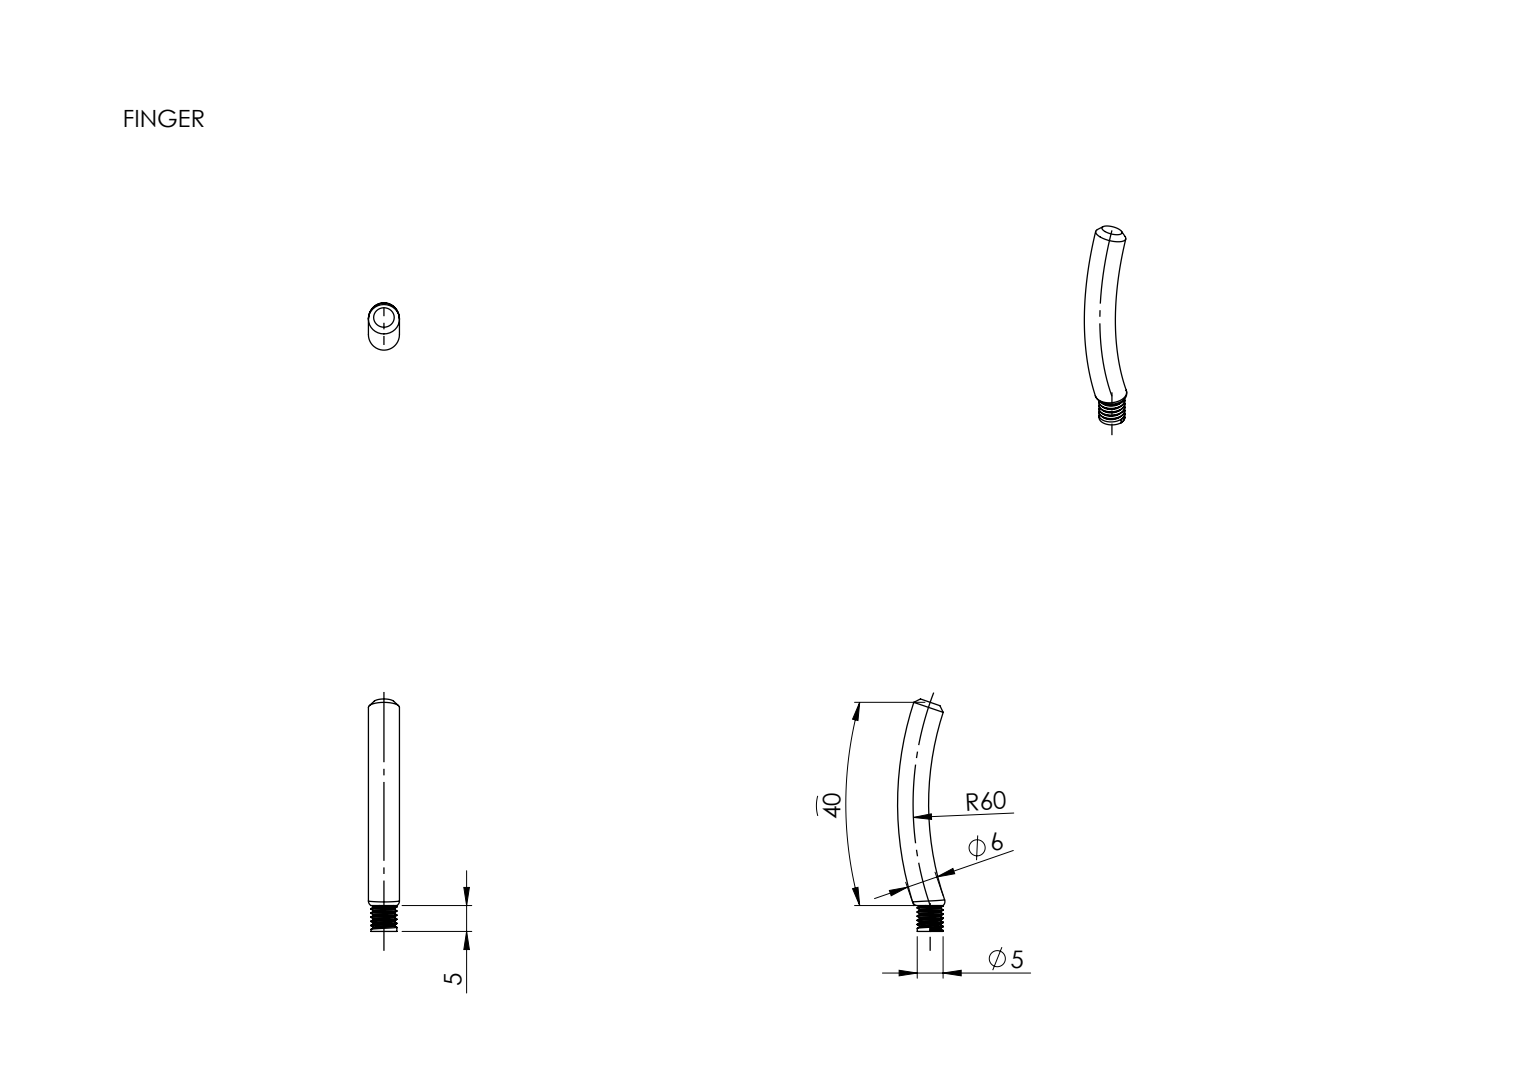
ISO-10303-21;
HEADER;
FILE_DESCRIPTION (('STEP AP214'),
    '1' );
FILE_NAME ('finger.step',
    '2026-10-04T10:31:01',
    ( '' ),
    ( '' ),
    'SwSTEP 2.0',
    'SolidWorks 2026',
    '' );
FILE_SCHEMA (( 'AUTOMOTIVE_DESIGN' ));
ENDSEC;

DATA;
#10=LINE ( 'NONE', #5828, #1733 ) ;
#16=CARTESIAN_POINT ( 'NONE',  ( 0.8561741729129460632, 185.8999999989075036, 9.066987299999999195 ) ) ;
#23=CARTESIAN_POINT ( 'NONE',  ( -2.191511056945971259, 226.6300844452854903, 5.385369267317587472 ) ) ;
#25=VERTEX_POINT ( 'NONE', #11007 ) ;
#31=CARTESIAN_POINT ( 'NONE',  ( -2.499999999999998224, 185.2500000000000284, 8.035533905932741305 ) ) ;
#33=CARTESIAN_POINT ( 'NONE',  ( -2.500000000000000444, 185.8999999978150584, 7.000000000000000000 ) ) ;
#39=CARTESIAN_POINT ( 'NONE',  ( -1.767766952966369320, 186.5999999978150754, 5.232233047033630235 ) ) ;
#40=CARTESIAN_POINT ( 'NONE',  ( 2.467000123265670641, 227.8390626820829823, 8.944723654098295285 ) ) ;
#43=CARTESIAN_POINT ( 'NONE',  ( -2.367714804004699136, 189.3873339094368191, 5.166511778942795452 ) ) ;
#55=CARTESIAN_POINT ( 'NONE',  ( -1.767766952966369765, 186.8300000002185186, 8.767766952966368876 ) ) ;
#57=CARTESIAN_POINT ( 'NONE',  ( 1.989910900261709470, 228.2393533748197569, 6.930657055068108363 ) ) ;
#64=CARTESIAN_POINT ( 'NONE',  ( -0.8561741729129470624, 185.5999999989075206, 9.066987300000000971 ) ) ;
#73=CARTESIAN_POINT ( 'NONE',  ( -1.732476358310940601, 189.0000000000000853, 8.805961798289683173 ) ) ;
#91=CARTESIAN_POINT ( 'NONE',  ( -1.461580736456473018, 188.7499999989075263, 5.538419263543527649 ) ) ;
#100=CARTESIAN_POINT ( 'NONE',  ( -2.809196860006122787, 226.9495188873497966, 6.326437523183426670 ) ) ;
#104=EDGE_LOOP ( 'NONE', ( #9975, #181, #5986, #469 ) ) ;
#106=CARTESIAN_POINT ( 'NONE',  ( 1.753917783834456179, 189.0000000000000568, 8.787807858281036388 ) ) ;
#116=DIRECTION ( 'NONE',  ( -6.123233995736766036E-17, 1.000000000000000000, 0.000000000000000000 ) ) ;
#118=CARTESIAN_POINT ( 'NONE',  ( -7.826584432629735133E-16, 189.2999999978150356, 9.500000000000001776 ) ) ;
#119=CARTESIAN_POINT ( 'NONE',  ( 1.829800800964088481, 226.5245823332902546, 5.074452397578279594 ) ) ;
#121=CARTESIAN_POINT ( 'NONE',  ( -2.425137606382978372, 188.9999999978561505, 7.628313597219490205 ) ) ;
#133=CARTESIAN_POINT ( 'NONE',  ( -2.500000000000000444, 186.7300000002184959, 7.000000000000000000 ) ) ;
#140=CARTESIAN_POINT ( 'NONE',  ( -1.461580736456473906, 186.3499999989074922, 8.461580736456474128 ) ) ;
#143=CARTESIAN_POINT ( 'NONE',  ( 8.809142651444723526E-17, 184.6499999989075320, 4.933012699999999029 ) ) ;
#148=B_SPLINE_CURVE_WITH_KNOTS ( 'NONE', 1,
 ( #12898, #4831 ),
 .UNSPECIFIED., .F., .F.,
 ( 2, 2 ),
 ( 0.000000000000000000, 1.000000000000000000 ),
 .UNSPECIFIED. ) ;
#150=CARTESIAN_POINT ( 'NONE',  ( 1.461580736456472573, 188.9499999989075150, 8.461580736456474128 ) ) ;
#164=VECTOR ( 'NONE', #7946, 1000.000000000000000 ) ;
#177=CARTESIAN_POINT ( 'NONE',  ( -2.923025936753522291, 227.5090509392885281, 7.973756422523831766 ) ) ;
#179=ORIENTED_EDGE ( 'NONE', *, *, #8379, .T. ) ;
#181=ORIENTED_EDGE ( 'NONE', *, *, #13568, .T. ) ;
#194=CARTESIAN_POINT ( 'NONE',  ( 4.404571325722361763E-17, 185.7699999975965568, 4.500000000000000000 ) ) ;
#195=CARTESIAN_POINT ( 'NONE',  ( -1.740752211025599738, 227.9442165381023528, 6.078285037125840340 ) ) ;
#196=CARTESIAN_POINT ( 'NONE',  ( 2.789580270747262780, 227.6450226773988845, 8.373868502673408543 ) ) ;
#197=CARTESIAN_POINT ( 'NONE',  ( 0.3061381340472814627, 189.0451911194899424, 10.17413847366682234 ) ) ;
#200=CARTESIAN_POINT ( 'NONE',  ( -0.2618185962740512407, 189.0446530151151023, 10.17853758010602760 ) ) ;
#208=CARTESIAN_POINT ( 'NONE',  ( 0.9639874461523436633, 228.2061259459514133, 10.02419290002115915 ) ) ;
#210=EDGE_CURVE ( 'NONE', #4790, #898, #15357, .T. ) ;
#217=CARTESIAN_POINT ( 'NONE',  ( -2.500000000000000444, 186.7800000002184504, 8.035533905932737753 ) ) ;
#219=CARTESIAN_POINT ( 'NONE',  ( 0.8799020092372641377, 228.8451675208714562, 8.680282862240067843 ) ) ;
#224=CARTESIAN_POINT ( 'NONE',  ( -2.066987300000001859, 187.8999999989075036, 7.856174172912944620 ) ) ;
#231=CARTESIAN_POINT ( 'NONE',  ( -0.8561741729129471734, 188.7999999989075093, 9.066987300000000971 ) ) ;
#233=CARTESIAN_POINT ( 'NONE',  ( -0.05280792143845736142, 189.0000000000001137, 9.499442202459045248 ) ) ;
#240=CARTESIAN_POINT ( 'NONE',  ( -0.8561741729129455081, 187.0999999989075206, 4.933012699999999029 ) ) ;
#250=CARTESIAN_POINT ( 'NONE',  ( -2.113934160113910998, 227.9745842263959048, 9.343330332359114365 ) ) ;
#251=CARTESIAN_POINT ( 'NONE',  ( -0.8561741729129470624, 188.9999999989074979, 9.066987299999999195 ) ) ;
#258=CARTESIAN_POINT ( 'NONE',  ( -2.548338711267991386, 226.7802694665861338, 5.827877803219676522 ) ) ;
#269=CARTESIAN_POINT ( 'NONE',  ( 1.035533905932737975, 184.8499999978150754, 4.500000000000000888 ) ) ;
#273=CARTESIAN_POINT ( 'NONE',  ( 1.767766952966369320, 185.6699999975965625, 5.232233047033630235 ) ) ;
#274=CARTESIAN_POINT ( 'NONE',  ( 0.1304739971030711432, 227.6100227634930775, 5.113114354890055502 ) ) ;
#276=CARTESIAN_POINT ( 'NONE',  ( -2.974673115704016713, 227.4156934420934419, 7.698994310615434600 ) ) ;
#277=CARTESIAN_POINT ( 'NONE',  ( -2.345330793980067607, 188.9999999986873149, 6.116719614743881372 ) ) ;
#283=CARTESIAN_POINT ( 'NONE',  ( 3.000012661665197200, 227.2854160473209504, 7.315512558684322819 ) ) ;
#291=CARTESIAN_POINT ( 'NONE',  ( -2.500000000000000444, 186.7500000000000000, 5.964466094067261359 ) ) ;
#293=CARTESIAN_POINT ( 'NONE',  ( -0.2610185499608090876, 227.6142484773064325, 5.125318457402467942 ) ) ;
#299=CARTESIAN_POINT ( 'NONE',  ( -1.965116437629976787E-16, 189.2499999989075263, 4.933012699999999029 ) ) ;
#301=CARTESIAN_POINT ( 'NONE',  ( -2.066987300000000971, 188.0999999989074922, 7.856174172912944620 ) ) ;
#309=CARTESIAN_POINT ( 'NONE',  ( 2.593621171579884699, 189.1921907459377792, 8.687688957072346341 ) ) ;
#311=CARTESIAN_POINT ( 'NONE',  ( 3.001999740804089711, 189.8855686313634124, 7.133436250992125416 ) ) ;
#316=CARTESIAN_POINT ( 'NONE',  ( 0.8561741729129460632, 186.6999999989075150, 9.066987299999999195 ) ) ;
#317=( BOUNDED_CURVE ( )  B_SPLINE_CURVE ( 2, ( #9057, #7531, #11422, #13807, #6512 ),
 .UNSPECIFIED., .F., .F. ) 
 B_SPLINE_CURVE_WITH_KNOTS ( ( 3, 2, 3 ),
 ( 0.8571428571428570953, 0.8750000000000000000, 0.8928571428571429047 ),
 .UNSPECIFIED. ) 
 CURVE ( )  GEOMETRIC_REPRESENTATION_ITEM ( )  RATIONAL_B_SPLINE_CURVE ( ( 1.000000000000000000, 0.9238795325112867385, 1.000000000000000000, 0.9238795325112867385, 1.000000000000000000 ) ) 
 REPRESENTATION_ITEM ( '' )  );
#320=VERTEX_POINT ( 'NONE', #684 ) ;
#327=CARTESIAN_POINT ( 'NONE',  ( -2.997549271363485701, 189.8887934741522088, 7.062685571753808844 ) ) ;
#330=( BOUNDED_CURVE ( )  B_SPLINE_CURVE ( 2, ( #15027, #7780, #6448, #7628, #12471, #4120, #1572, #12627, #6600 ),
 .UNSPECIFIED., .F., .F. ) 
 B_SPLINE_CURVE_WITH_KNOTS ( ( 3, 2, 2, 2, 3 ),
 ( 0.3571428571428572063, 0.3750000000000000555, 0.3928571428571429047, 0.4107142857142856984, 0.4285714285714285476 ),
 .UNSPECIFIED. ) 
 CURVE ( )  GEOMETRIC_REPRESENTATION_ITEM ( )  RATIONAL_B_SPLINE_CURVE ( ( 0.9999999999999997780, 0.9238795325112869605, 1.000000000000000000, 0.9238795325112867385, 1.000000000000000000, 0.9238795325112867385, 1.000000000000000000, 0.9238795325112867385, 1.000000000000000000 ) ) 
 REPRESENTATION_ITEM ( '' )  );
#340=CARTESIAN_POINT ( 'NONE',  ( 1.414552619335309291, 189.0000000000000853, 9.066428886377552843 ) ) ;
#347=CARTESIAN_POINT ( 'NONE',  ( -1.035533905932737753, 184.9499999978150413, 4.500000000000000888 ) ) ;
#352=CARTESIAN_POINT ( 'NONE',  ( 2.500000000000000444, 187.1199999975965795, 8.035533905932739529 ) ) ;
#353=CARTESIAN_POINT ( 'NONE',  ( -1.885954199498669270, 228.0508284750123664, 6.386186391668034368 ) ) ;
#354=CARTESIAN_POINT ( 'NONE',  ( -2.087773716237738331, 226.5967140655768048, 5.287030890998575927 ) ) ;
#356=CARTESIAN_POINT ( 'NONE',  ( -2.971600176645282421, 189.3276089958123976, 6.470516599052638540 ) ) ;
#363=CARTESIAN_POINT ( 'NONE',  ( 2.825502441289275968, 227.6141739403474844, 8.283116510204369121 ) ) ;
#369=CARTESIAN_POINT ( 'NONE',  ( -2.500000000000000444, 185.1500000000000057, 5.964466094067261359 ) ) ;
#371=CARTESIAN_POINT ( 'NONE',  ( -1.786743523428754976, 227.9724114945277051, 6.159713679416685572 ) ) ;
#375=CARTESIAN_POINT ( 'NONE',  ( -1.767766952966369542, 184.5000000000000000, 8.767766952966368876 ) ) ;
#377=CARTESIAN_POINT ( 'NONE',  ( -2.066987300000000083, 186.4499999989075150, 7.000000000000000000 ) ) ;
#380=CARTESIAN_POINT ( 'NONE',  ( 0.000000000000000000, 184.0000000000000000, 7.000000000000000000 ) ) ;
#381=CARTESIAN_POINT ( 'NONE',  ( -5.999999999999999112, 227.2817795252328210, 4.165129161027028459 ) ) ;
#383=CARTESIAN_POINT ( 'NONE',  ( 1.818048556411949068, 189.7463703733489524, 9.770364204685183296 ) ) ;
#388=CARTESIAN_POINT ( 'NONE',  ( -0.8070991676978370721, 189.0000000000000000, 4.628151146390497850 ) ) ;
#390=CARTESIAN_POINT ( 'NONE',  ( -1.461580736456473240, 185.7499999989074979, 8.461580736456472351 ) ) ;
#401=CARTESIAN_POINT ( 'NONE',  ( -0.3832019641432907187, 228.2493259063060691, 10.15123907897345568 ) ) ;
#410=CARTESIAN_POINT ( 'NONE',  ( 2.500000000000000444, 186.3499999978150754, 5.964466094067262247 ) ) ;
#414=ORIENTED_EDGE ( 'NONE', *, *, #5071, .T. ) ;
#416=CARTESIAN_POINT ( 'NONE',  ( 1.644293607015084646, 189.0000000000000568, 8.888752495498886574 ) ) ;
#422=CARTESIAN_POINT ( 'NONE',  ( -1.035533905932737975, 186.5499999978150640, 4.500000000000000888 ) ) ;
#423=CARTESIAN_POINT ( 'NONE',  ( 2.500000000000000444, 184.7499999978150527, 5.964466094067262247 ) ) ;
#427=CARTESIAN_POINT ( 'NONE',  ( -1.767766952966369765, 187.6699999975965625, 8.767766952966368876 ) ) ;
#428=CARTESIAN_POINT ( 'NONE',  ( 0.6320692372082544752, 228.2335842258707430, 10.10492066627648988 ) ) ;
#429=CARTESIAN_POINT ( 'NONE',  ( -2.980755195990519191, 227.3998431049529074, 7.652341518474168325 ) ) ;
#431=CARTESIAN_POINT ( 'NONE',  ( -2.464020019946891793, 189.7914691120035400, 9.078875626642586738 ) ) ;
#437=CARTESIAN_POINT ( 'NONE',  ( 2.938271602351877121, 227.0923189680254666, 6.746872328837914878 ) ) ;
#444=CARTESIAN_POINT ( 'NONE',  ( -1.035533905932739751, 186.9499999999999886, 9.500000000000003553 ) ) ;
#447=CARTESIAN_POINT ( 'NONE',  ( -1.385362557672197736, 227.7924883072852822, 5.640085252515396164 ) ) ;
#451=CARTESIAN_POINT ( 'NONE',  ( -1.456896669277396583E-16, 188.4499999989075150, 4.933012699999999029 ) ) ;
#453=CARTESIAN_POINT ( 'NONE',  ( -2.066987300000000527, 188.7999999989075093, 6.143825827087054492 ) ) ;
#454=ORIENTED_EDGE ( 'NONE', *, *, #12708, .F. ) ;
#461=CARTESIAN_POINT ( 'NONE',  ( 2.837060236510290157, 189.8314984584918079, 8.326472016722609837 ) ) ;
#469=ORIENTED_EDGE ( 'NONE', *, *, #9305, .F. ) ;
#470=CARTESIAN_POINT ( 'NONE',  ( -2.066987300000000971, 187.9999999989075263, 6.143825827087054492 ) ) ;
#488=EDGE_CURVE ( 'NONE', #14260, #5268, #1225, .T. ) ;
#504=CARTESIAN_POINT ( 'NONE',  ( -2.500000000000000444, 185.0999999978150754, 7.000000000000000000 ) ) ;
#506=CARTESIAN_POINT ( 'NONE',  ( 1.767766952966368654, 185.4699999975965454, 8.767766952966368876 ) ) ;
#507=CARTESIAN_POINT ( 'NONE',  ( 0.4870669733929915424, 228.2428440931186628, 10.13214456346285708 ) ) ;
#508=CARTESIAN_POINT ( 'NONE',  ( -0.3933619333212962643, 226.3329841201265253, 4.509674143907711041 ) ) ;
#517=CARTESIAN_POINT ( 'NONE',  ( 2.959395828221181191, 227.1267441636075262, 6.848257790201431661 ) ) ;
#523=CARTESIAN_POINT ( 'NONE',  ( -5.929230630780102373E-16, 186.2000000000000171, 9.500000000000001776 ) ) ;
#525=CARTESIAN_POINT ( 'NONE',  ( -1.313542798833678749, 227.7708088449086290, 5.577473728656160645 ) ) ;
#529=CARTESIAN_POINT ( 'NONE',  ( -2.500000000000000444, 185.2000000000000171, 7.000000000000000000 ) ) ;
#531=CARTESIAN_POINT ( 'NONE',  ( 2.066987300000000083, 186.8999999989075320, 6.143825827087054492 ) ) ;
#533=VECTOR ( 'NONE', #5560, 1000.000000000000000 ) ;
#534=EDGE_CURVE ( 'NONE', #7505, #3363, #14632, .T. ) ;
#537=CARTESIAN_POINT ( 'NONE',  ( 0.03982005317027621089, 190.0874997052910658, 4.201869497416318211 ) ) ;
#539=CARTESIAN_POINT ( 'NONE',  ( 3.012851251850296563, 189.2892816699357468, 7.217589605582900525 ) ) ;
#542=CARTESIAN_POINT ( 'NONE',  ( 1.582454879690585958, 190.0440573869416312, 4.656039093731057399 ) ) ;
#547=CARTESIAN_POINT ( 'NONE',  ( 0.8561741729129458411, 187.4999999989075548, 9.066987299999999195 ) ) ;
#555=EDGE_LOOP ( 'NONE', ( #8215, #1137, #7408, #11561, #3893 ) ) ;
#557=EDGE_CURVE ( 'NONE', #1272, #898, #148, .T. ) ;
#569=ORIENTED_EDGE ( 'NONE', *, *, #5071, .F. ) ;
#578=CARTESIAN_POINT ( 'NONE',  ( 2.500000000000000444, 187.0499999978150640, 8.035533905932739529 ) ) ;
#583=CARTESIAN_POINT ( 'NONE',  ( 1.035533905932738197, 189.4199999975965625, 9.500000000000003553 ) ) ;
#584=CARTESIAN_POINT ( 'NONE',  ( 2.379866841847371628, 227.8775224696199473, 9.057852156131547261 ) ) ;
#585=CARTESIAN_POINT ( 'NONE',  ( -2.521794825564176890, 226.7667903661470348, 5.788166807254388146 ) ) ;
#589=ORIENTED_EDGE ( 'NONE', *, *, #3180, .F. ) ;
#592=CARTESIAN_POINT ( 'NONE',  ( 1.461580736456473462, 184.3499999989074922, 5.538419263543526760 ) ) ;
#599=CARTESIAN_POINT ( 'NONE',  ( 2.500000000000000000, 188.7999999999999829, 7.000000000000000000 ) ) ;
#601=CARTESIAN_POINT ( 'NONE',  ( 2.500000000000000444, 186.4000000000000057, 7.000000000000000000 ) ) ;
#602=CARTESIAN_POINT ( 'NONE',  ( -1.938951794131667850, 228.1124887269953092, 6.564264716264994526 ) ) ;
#606=CARTESIAN_POINT ( 'NONE',  ( -2.500000000000000444, 188.3499999999999943, 5.964466094067261359 ) ) ;
#608=CARTESIAN_POINT ( 'NONE',  ( -2.066987300000000527, 187.2999999989075661, 7.856174172912944620 ) ) ;
#611=CARTESIAN_POINT ( 'NONE',  ( 2.500000000000000444, 186.2999999978150356, 7.000000000000000000 ) ) ;
#615=CARTESIAN_POINT ( 'NONE',  ( 1.855150134049648347, 188.9999999974870946, 5.314312548248043555 ) ) ;
#618=CARTESIAN_POINT ( 'NONE',  ( 1.579185070784824285, 228.6572036374857078, 8.137432446265082220 ) ) ;
#623=CARTESIAN_POINT ( 'NONE',  ( 0.8561741729129461742, 186.4999999989075263, 9.066987300000000971 ) ) ;
#625=ORIENTED_EDGE ( 'NONE', *, *, #13568, .F. ) ;
#627=CARTESIAN_POINT ( 'NONE',  ( 2.500000000000000444, 185.5999999999999943, 7.000000000000000000 ) ) ;
#630=CARTESIAN_POINT ( 'NONE',  ( 2.066987300000000527, 184.2499999989074979, 7.000000000000000000 ) ) ;
#649=CARTESIAN_POINT ( 'NONE',  ( -0.8561741729129466183, 184.9999999989074979, 9.066987299999999195 ) ) ;
#656=CARTESIAN_POINT ( 'NONE',  ( 1.498625850689462968, 228.1261123260860018, 9.788931089129667029 ) ) ;
#666=B_SPLINE_CURVE_WITH_KNOTS ( 'NONE', 3,
 ( #4284, #3090, #14057, #693, #7943, #3165, #8023, #4442, #1965, #6841, #9296, #8106, #12945, #2045, #9700, #7070, #6037, #13342, #14371, #11905, #7151, #2363 ),
 .UNSPECIFIED., .F., .F.,
 ( 4, 2, 2, 2, 2, 2, 2, 2, 2, 2, 4 ),
 ( 0.5000000000000000000, 0.5625000000000006661, 0.5937500000000005551, 0.6250000000000004441, 0.6875000000000004441, 0.7500000000000003331, 0.7812500000000003331, 0.8125000000000002220, 0.8750000000000002220, 0.9375000000000001110, 1.000000000000000000 ),
 .UNSPECIFIED. ) ;
#673=CARTESIAN_POINT ( 'NONE',  ( -7.420008617947670970E-16, 188.5999999999999943, 9.500000000000001776 ) ) ;
#674=CARTESIAN_POINT ( 'NONE',  ( -1.813734975128623139, 228.5291423394705532, 7.767584113458720019 ) ) ;
#681=CARTESIAN_POINT ( 'NONE',  ( 2.500000000000000444, 187.1499999999999773, 8.035533905932739529 ) ) ;
#683=ADVANCED_FACE ( 'NONE', ( #7913 ), #4483, .T. ) ;
#684=CARTESIAN_POINT ( 'NONE',  ( 2.500000000000000444, 184.7999999999999829, 7.000000000000000000 ) ) ;
#686=LINE ( 'NONE', #12938, #533 ) ;
#690=CARTESIAN_POINT ( 'NONE',  ( -0.9617334577332378176, 228.2042837055383302, 10.01878807149740602 ) ) ;
#691=CARTESIAN_POINT ( 'NONE',  ( 0.4407554187462536799, 188.9999999991368895, 4.532388850900320065 ) ) ;
#693=CARTESIAN_POINT ( 'NONE',  ( -0.8829701019949064422, 227.6750070165890349, 5.300792584290398679 ) ) ;
#694=CARTESIAN_POINT ( 'NONE',  ( 1.851056454904606685, 228.5003429013454763, 7.684409693542115782 ) ) ;
#699=CARTESIAN_POINT ( 'NONE',  ( -1.461580736456473018, 188.7499999989075263, 5.538419263543527649 ) ) ;
#701=CARTESIAN_POINT ( 'NONE',  ( 1.035533905932738419, 184.6500000000000057, 9.500000000000000000 ) ) ;
#710=CARTESIAN_POINT ( 'NONE',  ( -1.767766952966369098, 185.0999999999999943, 5.232233047033630235 ) ) ;
#716=CARTESIAN_POINT ( 'NONE',  ( -5.999999999999999112, 229.2449477060184222, 9.834870838912449287 ) ) ;
#728=CARTESIAN_POINT ( 'NONE',  ( 2.500000000000000444, 184.7999999999999829, 7.000000000000000000 ) ) ;
#733=CARTESIAN_POINT ( 'NONE',  ( -1.035533905932737975, 188.9499999978150697, 4.500000000000000888 ) ) ;
#741=CARTESIAN_POINT ( 'NONE',  ( 0.09789622041826544219, 228.2551367208810689, 10.16828408546989237 ) ) ;
#749=CARTESIAN_POINT ( 'NONE',  ( 1.035533905932738197, 189.3499999978150754, 9.500000000000000000 ) ) ;
#759=CARTESIAN_POINT ( 'NONE',  ( -1.035533905932737975, 188.2500000000000000, 4.500000000000000888 ) ) ;
#761=CARTESIAN_POINT ( 'NONE',  ( -1.987493679921816137, 228.2178828950600860, 6.868649084925799286 ) ) ;
#763=AXIS2_PLACEMENT_3D ( 'NONE', #4855, #7470, #14549 ) ;
#766=CARTESIAN_POINT ( 'NONE',  ( 1.767766952966369098, 187.2999999999999829, 5.232233047033630235 ) ) ;
#774=CARTESIAN_POINT ( 'NONE',  ( -0.1991118202061275544, 190.0875178197513549, 4.201689379953633008 ) ) ;
#777=CARTESIAN_POINT ( 'NONE',  ( 1.035533905932737975, 184.0800000002185186, 4.500000000000000888 ) ) ;
#779=CARTESIAN_POINT ( 'NONE',  ( 1.725625307041983136, 227.9349420198840903, 6.051499699527947307 ) ) ;
#784=CARTESIAN_POINT ( 'NONE',  ( 5.082197683525802034E-17, 185.2499999989074979, 4.933012699999999029 ) ) ;
#791=CARTESIAN_POINT ( 'NONE',  ( -1.461580736456473018, 185.3499999989074922, 5.538419263543526760 ) ) ;
#796=CARTESIAN_POINT ( 'NONE',  ( 3.659182332138577465E-16, 187.9952603975225713, 3.440894205938198613 ) ) ;
#811=CARTESIAN_POINT ( 'NONE',  ( -1.767766952966369765, 189.1999999978150697, 8.767766952966368876 ) ) ;
#813=CARTESIAN_POINT ( 'NONE',  ( 2.500000000000000444, 185.4999999978150527, 7.000000000000000000 ) ) ;
#819=CARTESIAN_POINT ( 'NONE',  ( 3.000032282732917555, 227.2742683068891552, 7.282695486718367306 ) ) ;
#823=( BOUNDED_CURVE ( )  B_SPLINE_CURVE ( 2, ( #1831, #12882, #13771, #14977, #5431, #11461, #11535, #11617, #4068 ),
 .UNSPECIFIED., .F., .F. ) 
 B_SPLINE_CURVE_WITH_KNOTS ( ( 3, 2, 2, 2, 3 ),
 ( 0.5000000000000000000, 0.5178571428571429047, 0.5357142857142856984, 0.5535714285714286031, 0.5714285714285713969 ),
 .UNSPECIFIED. ) 
 CURVE ( )  GEOMETRIC_REPRESENTATION_ITEM ( )  RATIONAL_B_SPLINE_CURVE ( ( 1.000000000000000000, 0.9238795325112867385, 1.000000000000000000, 0.9238795325112867385, 1.000000000000000000, 0.9238795325112867385, 1.000000000000000000, 0.9238795325112867385, 1.000000000000000000 ) ) 
 REPRESENTATION_ITEM ( '' )  );
#832=PRESENTATION_STYLE_ASSIGNMENT (( #6370 ) ) ;
#837=CARTESIAN_POINT ( 'NONE',  ( 1.035533905932737975, 184.8499999978150754, 4.500000000000000888 ) ) ;
#839=CARTESIAN_POINT ( 'NONE',  ( -0.6401557763822781633, 228.8776351522889172, 8.774051233606112277 ) ) ;
#843=CARTESIAN_POINT ( 'NONE',  ( 0.03582210218219494119, 189.0000000000000284, 4.500171129856880725 ) ) ;
#844=CARTESIAN_POINT ( 'NONE',  ( 2.500000000000000444, 188.0500000000000114, 5.964466094067262247 ) ) ;
#845=CARTESIAN_POINT ( 'NONE',  ( -1.767766952966369320, 187.3999999978150584, 5.232233047033630235 ) ) ;
#851=CARTESIAN_POINT ( 'NONE',  ( -2.781333881087624249, 226.9279571253883319, 6.262926915399051886 ) ) ;
#856=CARTESIAN_POINT ( 'NONE',  ( 1.362382138968808887, 227.7849605967929847, 5.618344795260735935 ) ) ;
#861=CARTESIAN_POINT ( 'NONE',  ( 2.066987299999999639, 189.2499999989075263, 7.000000000000000000 ) ) ;
#864=CARTESIAN_POINT ( 'NONE',  ( 2.500000000000000444, 186.4000000000000057, 7.000000000000000000 ) ) ;
#865=CARTESIAN_POINT ( 'NONE',  ( 1.461580736456473018, 185.3499999989075206, 5.538419263543527649 ) ) ;
#867=CARTESIAN_POINT ( 'NONE',  ( -9.825582188149883933E-17, 187.6499999989075320, 4.933012699999999029 ) ) ;
#872=CARTESIAN_POINT ( 'NONE',  ( 3.659182332138577465E-16, 195.9172377311516016, 6.220370292208427188 ) ) ;
#875=DIRECTION ( 'NONE',  ( -6.123233995736766036E-17, 1.000000000000000000, 0.000000000000000000 ) ) ;
#881=CARTESIAN_POINT ( 'NONE',  ( 1.002352689154774934, 228.8297273714526625, 8.635690830070354096 ) ) ;
#886=CARTESIAN_POINT ( 'NONE',  ( 0.8561741729129461742, 185.0999999989074922, 9.066987299999999195 ) ) ;
#892=CARTESIAN_POINT ( 'NONE',  ( 2.998712701283978710, 227.3219367242041926, 7.423021690895281743 ) ) ;
#893=CARTESIAN_POINT ( 'NONE',  ( -1.238695443643032412, 228.1695118093442716, 9.916540120957755278 ) ) ;
#898=VERTEX_POINT ( 'NONE', #13447 ) ;
#911=CARTESIAN_POINT ( 'NONE',  ( 2.500000000000000444, 185.5499999978150640, 5.964466094067262247 ) ) ;
#912=CARTESIAN_POINT ( 'NONE',  ( -1.785671180686238868, 228.5485690224869586, 7.823689482036285447 ) ) ;
#915=CARTESIAN_POINT ( 'NONE',  ( -0.1354819475358782221, 189.4421779970482760, 3.974290229956241038 ) ) ;
#916=CARTESIAN_POINT ( 'NONE',  ( 1.035533905932737753, 186.5499999999999829, 4.500000000000000888 ) ) ;
#923=EDGE_CURVE ( 'NONE', #15371, #5418, #15489, .T. ) ;
#925=CARTESIAN_POINT ( 'NONE',  ( -2.774519402982507543, 226.9225964823893378, 6.247138756163614914 ) ) ;
#926=PRESENTATION_STYLE_ASSIGNMENT (( #5953 ) ) ;
#927=CARTESIAN_POINT ( 'NONE',  ( 1.616071383507818870, 190.0421234246860820, 4.677467377199475251 ) ) ;
#928=CARTESIAN_POINT ( 'NONE',  ( -2.500000000000000444, 184.3800000002184731, 8.035533905932737753 ) ) ;
#931=CARTESIAN_POINT ( 'NONE',  ( 1.050562149602352946, 228.8138732705275231, 8.589903282340008772 ) ) ;
#936=CARTESIAN_POINT ( 'NONE',  ( -2.066987300000001415, 188.8999999989075320, 7.856174172912944620 ) ) ;
#946=CARTESIAN_POINT ( 'NONE',  ( -0.8561741729129457301, 185.2999999989075661, 4.933012699999999029 ) ) ;
#951=CARTESIAN_POINT ( 'NONE',  ( -5.999999999999999112, 187.2933328889893403, 9.583808270834989429 ) ) ;
#952=CARTESIAN_POINT ( 'NONE',  ( -1.097593809647108287, 189.0000000000000000, 9.257041379597499287 ) ) ;
#956=AXIS2_PLACEMENT_3D ( 'NONE', #13283, #2700, #14724 ) ;
#961=CARTESIAN_POINT ( 'NONE',  ( -0.8561741729129467293, 184.9999999989074979, 9.066987299999999195 ) ) ;
#963=ORIENTED_EDGE ( 'NONE', *, *, #15525, .T. ) ;
#967=CARTESIAN_POINT ( 'NONE',  ( -0.8561741729129455081, 186.2999999989075093, 4.933012699999999029 ) ) ;
#968=EDGE_CURVE ( 'NONE', #3363, #12097, #1421, .T. ) ;
#974=CARTESIAN_POINT ( 'NONE',  ( 2.257611286988003396, 226.6535225833466427, 5.454435118953909978 ) ) ;
#981=ORIENTED_EDGE ( 'NONE', *, *, #4957, .F. ) ;
#995=CARTESIAN_POINT ( 'NONE',  ( 2.500000000000000000, 188.0000000000000000, 7.000000000000000000 ) ) ;
#996=CARTESIAN_POINT ( 'NONE',  ( 1.455795469679321608, 228.1339131991090596, 9.811868761735363265 ) ) ;
#998=CARTESIAN_POINT ( 'NONE',  ( 0.07162669437691278340, 189.0000000000000000, 4.501026287322612340 ) ) ;
#1010=CARTESIAN_POINT ( 'NONE',  ( -2.999884802989111421, 227.2993432378640932, 7.356512168893465820 ) ) ;
#1011=( NAMED_UNIT ( * ) PLANE_ANGLE_UNIT ( ) SI_UNIT ( $, .RADIAN. ) );
#1013=CARTESIAN_POINT ( 'NONE',  ( -1.767766952966369542, 184.4300000002185129, 8.767766952966368876 ) ) ;
#1015=CARTESIAN_POINT ( 'NONE',  ( -1.986723294250032357, 228.3028615258686500, 7.114072217564876510 ) ) ;
#1020=CARTESIAN_POINT ( 'NONE',  ( 0.8561741729129460632, 188.0999999989074922, 9.066987300000000971 ) ) ;
#1023=CARTESIAN_POINT ( 'NONE',  ( 2.500000000000000444, 186.3499999999999943, 8.035533905932739529 ) ) ;
#1026=CARTESIAN_POINT ( 'NONE',  ( -2.500000000000000444, 186.6999999978150697, 7.000000000000000000 ) ) ;
#1027=CARTESIAN_POINT ( 'NONE',  ( -0.8561741729129469514, 186.3999999989075320, 9.066987300000000971 ) ) ;
#1041=CARTESIAN_POINT ( 'NONE',  ( -2.066987300000000083, 185.5999999989075491, 6.143825827087054492 ) ) ;
#1048=CARTESIAN_POINT ( 'NONE',  ( 2.066987299999999195, 188.3999999989075036, 7.856174172912946396 ) ) ;
#1054=CARTESIAN_POINT ( 'NONE',  ( 2.191560967657306680, 226.6301005958437145, 5.385416860794732585 ) ) ;
#1075=CARTESIAN_POINT ( 'NONE',  ( -1.035533905932739751, 188.4499999978150413, 9.500000000000003553 ) ) ;
#1076=CARTESIAN_POINT ( 'NONE',  ( 2.441738273555474681, 226.7282248110694809, 5.674544857840881029 ) ) ;
#1078=CARTESIAN_POINT ( 'NONE',  ( -2.102556124205833044, 189.0000000003525997, 5.635613679834785117 ) ) ;
#1079=EDGE_CURVE ( 'NONE', #14331, #15449, #9378, .T. ) ;
#1087=CARTESIAN_POINT ( 'NONE',  ( 2.658620627125748204, 226.8422998350077080, 6.010601022363255552 ) ) ;
#1090=CARTESIAN_POINT ( 'NONE',  ( -2.985771267271970064, 227.3851189813470910, 7.609035584520301043 ) ) ;
#1092=CARTESIAN_POINT ( 'NONE',  ( 1.035533905932737753, 188.0800000002184902, 4.500000000000000888 ) ) ;
#1094=CARTESIAN_POINT ( 'NONE',  ( -0.06647456835015956578, 227.6089819833846093, 5.110108522575333545 ) ) ;
#1098=ORIENTED_EDGE ( 'NONE', *, *, #5480, .T. ) ;
#1099=CARTESIAN_POINT ( 'NONE',  ( -0.8561741729129471734, 187.9999999989075263, 9.066987300000000971 ) ) ;
#1101=CARTESIAN_POINT ( 'NONE',  ( 2.066987300000000083, 187.3999999989075320, 7.856174172912946396 ) ) ;
#1107=CARTESIAN_POINT ( 'NONE',  ( 5.999999999999999112, 229.2449477060184222, 9.834870838912449287 ) ) ;
#1108=CARTESIAN_POINT ( 'NONE',  ( 1.461580736456472573, 188.1499999989075036, 8.461580736456474128 ) ) ;
#1113=DIRECTION ( 'NONE',  ( 2.168404344970946942E-15, -1.000000000000000000, -0.000000000000000000 ) ) ;
#1125=CARTESIAN_POINT ( 'NONE',  ( 1.461580736456472795, 188.5499999989075093, 5.538419263543527649 ) ) ;
#1131=CARTESIAN_POINT ( 'NONE',  ( 0.4902782441471901231, 226.3376063806459513, 4.523301387120397088 ) ) ;
#1136=ORIENTED_EDGE ( 'NONE', *, *, #3553, .F. ) ;
#1137=ORIENTED_EDGE ( 'NONE', *, *, #5238, .T. ) ;
#1150=CARTESIAN_POINT ( 'NONE',  ( -2.500000000000000444, 188.2499999978150242, 5.964466094067261359 ) ) ;
#1151=CARTESIAN_POINT ( 'NONE',  ( 2.734462269239809729, 226.8914732116195125, 6.155466831691636109 ) ) ;
#1158=EDGE_LOOP ( 'NONE', ( #4293, #1590, #2533, #13794 ) ) ;
#1164=CARTESIAN_POINT ( 'NONE',  ( -1.569056679521910747, 226.4669167303270285, 4.904463601914050841 ) ) ;
#1168=CARTESIAN_POINT ( 'NONE',  ( 2.500000000000000444, 187.9800000002184959, 5.964466094067262247 ) ) ;
#1170=CARTESIAN_POINT ( 'NONE',  ( 1.986575337946455022, 228.3035988107396292, 7.116201538324070874 ) ) ;
#1175=CARTESIAN_POINT ( 'NONE',  ( -2.066987300000000971, 187.8499999989074922, 7.000000000000000000 ) ) ;
#1176=CARTESIAN_POINT ( 'NONE',  ( -4.811147140404425926E-16, 185.6499999989075320, 9.066987300000000971 ) ) ;
#1185=CARTESIAN_POINT ( 'NONE',  ( 1.214065608363191773, 189.0732342899627554, 9.931872992141947520 ) ) ;
#1190=CARTESIAN_POINT ( 'NONE',  ( 2.500000000000000444, 187.2500000000000000, 5.964466094067262247 ) ) ;
#1192=ORIENTED_EDGE ( 'NONE', *, *, #7499, .T. ) ;
#1196=ORIENTED_EDGE ( 'NONE', *, *, #14425, .T. ) ;
#1201=CARTESIAN_POINT ( 'NONE',  ( -0.8561741729129467293, 186.5999999989075206, 9.066987299999999195 ) ) ;
#1208=CARTESIAN_POINT ( 'NONE',  ( -1.586193948774629714, 228.1096603596491832, 9.740555404025270647 ) ) ;
#1225=( BOUNDED_CURVE ( )  B_SPLINE_CURVE ( 2, ( #7222, #1312, #3703, #5945, #2434, #10948, #6026, #13171, #4990 ),
 .UNSPECIFIED., .F., .F. ) 
 B_SPLINE_CURVE_WITH_KNOTS ( ( 3, 2, 2, 2, 3 ),
 ( 0.6428571428571429047, 0.6607142857142856984, 0.6785714285714286031, 0.6964285714285713969, 0.7142857142857143016 ),
 .UNSPECIFIED. ) 
 CURVE ( )  GEOMETRIC_REPRESENTATION_ITEM ( )  RATIONAL_B_SPLINE_CURVE ( ( 1.000000000000000000, 0.9238795325112867385, 1.000000000000000000, 0.9238795325112867385, 1.000000000000000000, 0.9238795325112867385, 1.000000000000000000, 0.9238795325112867385, 1.000000000000000000 ) ) 
 REPRESENTATION_ITEM ( '' )  );
#1227=CARTESIAN_POINT ( 'NONE',  ( -1.767766952966369320, 188.2999999999999829, 5.232233047033630235 ) ) ;
#1230=CARTESIAN_POINT ( 'NONE',  ( 1.035533905932737753, 188.0499999978150640, 4.500000000000000888 ) ) ;
#1231=CARTESIAN_POINT ( 'NONE',  ( 1.978507955918972439, 228.0159604248740663, 9.465015589616863068 ) ) ;
#1235=CARTESIAN_POINT ( 'NONE',  ( -1.760080037233190620, 188.9999999985105887, 5.215340696719847458 ) ) ;
#1247=CARTESIAN_POINT ( 'NONE',  ( 1.767766952966369320, 184.0999999999999943, 5.232233047033630235 ) ) ;
#1249=CARTESIAN_POINT ( 'NONE',  ( 0.5151998000674417044, 228.8897689535086784, 8.809094343595948118 ) ) ;
#1253=CARTESIAN_POINT ( 'NONE',  ( -1.456896669277396583E-16, 188.4499999989075150, 4.933012699999999029 ) ) ;
#1254=CARTESIAN_POINT ( 'NONE',  ( 1.461580736456472573, 187.3499999989074922, 8.461580736456474128 ) ) ;
#1262=CARTESIAN_POINT ( 'NONE',  ( -1.474837674502392115, 189.0000000000000568, 9.021725798137643082 ) ) ;
#1272=VERTEX_POINT ( 'NONE', #10086 ) ;
#1281=CARTESIAN_POINT ( 'NONE',  ( -5.421010862427522170E-16, 186.6499999989075320, 9.066987300000000971 ) ) ;
#1288=CARTESIAN_POINT ( 'NONE',  ( -3.000008639299222235, 227.3051114066062155, 7.373492455173472848 ) ) ;
#1301=CARTESIAN_POINT ( 'NONE',  ( 0.000000000000000000, 184.0000000000000000, 7.000000000000000000 ) ) ;
#1303=CARTESIAN_POINT ( 'NONE',  ( -4.743384504624081899E-17, 187.2999999978150356, 4.500000000000000000 ) ) ;
#1305=CARTESIAN_POINT ( 'NONE',  ( 2.053141855112443626, 226.5855735425530497, 5.254201149538955562 ) ) ;
#1308=CARTESIAN_POINT ( 'NONE',  ( -2.990615845299959386, 189.8642828410552568, 7.611177514557324386 ) ) ;
#1312=CARTESIAN_POINT ( 'NONE',  ( -2.500000000000001776, 187.6500000000000057, 8.035533905932737753 ) ) ;
#1316=( BOUNDED_CURVE ( )  B_SPLINE_CURVE ( 2, ( #3770, #7290, #8570, #6015, #13628, #12126, #1227, #6178, #2507 ),
 .UNSPECIFIED., .F., .F. ) 
 B_SPLINE_CURVE_WITH_KNOTS ( ( 3, 2, 2, 2, 3 ),
 ( 0.7142857142857143016, 0.7321428571428570953, 0.7500000000000000000, 0.7678571428571429047, 0.7857142857142856984 ),
 .UNSPECIFIED. ) 
 CURVE ( )  GEOMETRIC_REPRESENTATION_ITEM ( )  RATIONAL_B_SPLINE_CURVE ( ( 1.000000000000000000, 0.9238795325112867385, 1.000000000000000000, 0.9238795325112867385, 1.000000000000000000, 0.9238795325112867385, 1.000000000000000000, 0.9238795325112867385, 1.000000000000000000 ) ) 
 REPRESENTATION_ITEM ( '' )  );
#1322=CARTESIAN_POINT ( 'NONE',  ( 1.035533905932738197, 186.9800000002184674, 9.500000000000003553 ) ) ;
#1325=CARTESIAN_POINT ( 'NONE',  ( 1.159630251547017377, 228.7900363578050928, 8.521060918829135744 ) ) ;
#1329=ADVANCED_FACE ( 'NONE', ( #15019 ), #4027, .T. ) ;
#1331=CARTESIAN_POINT ( 'NONE',  ( 1.461580736456473240, 186.7499999989075263, 5.538419263543526760 ) ) ;
#1332=CARTESIAN_POINT ( 'NONE',  ( -0.8561741729129469514, 184.7999999989075093, 9.066987300000000971 ) ) ;
#1340=CARTESIAN_POINT ( 'NONE',  ( 5.999999999999999112, 188.6555110544239824, 3.692234042173051289 ) ) ;
#1348=( BOUNDED_CURVE ( )  B_SPLINE_CURVE ( 2, ( #10407, #14208, #8258, #15500, #4597, #14130, #12939, #9217, #6837 ),
 .UNSPECIFIED., .F., .F. ) 
 B_SPLINE_CURVE_WITH_KNOTS ( ( 3, 2, 2, 2, 3 ),
 ( 0.4285714285714285476, 0.4464285714285714524, 0.4642857142857143016, 0.4821428571428571508, 0.5000000000000000000 ),
 .UNSPECIFIED. ) 
 CURVE ( )  GEOMETRIC_REPRESENTATION_ITEM ( )  RATIONAL_B_SPLINE_CURVE ( ( 1.000000000000000000, 0.9238795325112867385, 1.000000000000000000, 0.9238795325112867385, 1.000000000000000000, 0.9238795325112867385, 1.000000000000000000, 0.9238795325112867385, 1.000000000000000000 ) ) 
 REPRESENTATION_ITEM ( '' )  );
#1353=DIRECTION ( 'NONE',  ( -1.000000000000000000, -6.123233995736766036E-17, 0.000000000000000000 ) ) ;
#1368=CARTESIAN_POINT ( 'NONE',  ( -2.980755195990519191, 227.3998431049529074, 7.652341518474168325 ) ) ;
#1374=CARTESIAN_POINT ( 'NONE',  ( 0.6408967124214390854, 189.0000000000000000, 9.420550828545728450 ) ) ;
#1383=CARTESIAN_POINT ( 'NONE',  ( 1.035533905932737975, 185.7199999975966023, 4.500000000000000888 ) ) ;
#1384=CARTESIAN_POINT ( 'NONE',  ( -1.673363231402341000, 227.9073979391035891, 5.971950823222174520 ) ) ;
#1385=CARTESIAN_POINT ( 'NONE',  ( 1.059913075168976260, 226.3867898013274669, 4.668296007112484602 ) ) ;
#1386=CARTESIAN_POINT ( 'NONE',  ( -0.2831953767659359800, 189.6983146630735177, 10.38325066061015178 ) ) ;
#1392=CARTESIAN_POINT ( 'NONE',  ( 0.07962197837297851910, 190.0874091994478761, 4.202769589527710181 ) ) ;
#1397=CARTESIAN_POINT ( 'NONE',  ( -1.035533905932737975, 186.5800000002185470, 4.500000000000000888 ) ) ;
#1400=CARTESIAN_POINT ( 'NONE',  ( 1.637003574519428017, 228.6312591184326948, 8.062503195461440342 ) ) ;
#1405=CARTESIAN_POINT ( 'NONE',  ( 1.767766952966368654, 185.5000000000000000, 8.767766952966368876 ) ) ;
#1421=LINE ( 'NONE', #10104, #7537 ) ;
#1424=CARTESIAN_POINT ( 'NONE',  ( -6.403569081242510563E-16, 188.2499999989075263, 9.066987300000000971 ) ) ;
#1434=CARTESIAN_POINT ( 'NONE',  ( -1.815878914417024204, 228.0587508443335309, 9.590870893335578629 ) ) ;
#1441=CARTESIAN_POINT ( 'NONE',  ( -1.585166063744550602, 226.4701105292460568, 4.913902397277155387 ) ) ;
#1446=CARTESIAN_POINT ( 'NONE',  ( 1.742858872693429761, 189.0000000000000000, 5.171082332538968984 ) ) ;
#1453=CARTESIAN_POINT ( 'NONE',  ( -6.844026213814746740E-16, 187.6999999978150697, 9.500000000000001776 ) ) ;
#1454=CARTESIAN_POINT ( 'NONE',  ( 2.066987300000000527, 185.0499999989075093, 7.000000000000000000 ) ) ;
#1459=CARTESIAN_POINT ( 'NONE',  ( 1.767766952966369320, 184.8699999975965511, 5.232233047033630235 ) ) ;
#1460=CARTESIAN_POINT ( 'NONE',  ( -1.987493679921816137, 228.2178828950600860, 6.868649084925799286 ) ) ;
#1461=CARTESIAN_POINT ( 'NONE',  ( -2.753288529192227774, 227.6732037325579654, 8.456785184543583966 ) ) ;
#1464=CARTESIAN_POINT ( 'NONE',  ( -2.880481771649630485, 189.8381383517797758, 8.187469944237161457 ) ) ;
#1470=CARTESIAN_POINT ( 'NONE',  ( 2.773164530494548696, 227.6577475117620679, 8.411308552413421680 ) ) ;
#1478=CARTESIAN_POINT ( 'NONE',  ( -1.035533905932739529, 185.3499999999999659, 9.500000000000003553 ) ) ;
#1480=CARTESIAN_POINT ( 'NONE',  ( 0.6402346998162695701, 228.8776282932165600, 8.774031424212344277 ) ) ;
#1484=CARTESIAN_POINT ( 'NONE',  ( 2.066987300000000083, 189.0999999989075206, 6.143825827087054492 ) ) ;
#1487=CARTESIAN_POINT ( 'NONE',  ( -0.8561741729129455081, 186.2999999989075093, 4.933012699999999029 ) ) ;
#1493=CARTESIAN_POINT ( 'NONE',  ( -5.999999999999999112, 194.5935680195190116, 12.11154058223188379 ) ) ;
#1497=FACE_OUTER_BOUND ( 'NONE', #555, .T. ) ;
#1499=CARTESIAN_POINT ( 'NONE',  ( -2.500000000000000444, 188.2499999978150527, 5.964466094067261359 ) ) ;
#1500=CARTESIAN_POINT ( 'NONE',  ( 2.390857953333830554, 189.7853064097493530, 9.182117214708636510 ) ) ;
#1505=CARTESIAN_POINT ( 'NONE',  ( 2.066987300000000083, 186.0499999989075093, 7.000000000000000000 ) ) ;
#1515=CARTESIAN_POINT ( 'NONE',  ( -1.055448890735882106, 228.1934063406578446, 9.986798501930948646 ) ) ;
#1524=CARTESIAN_POINT ( 'NONE',  ( -1.035533905932737975, 186.5499999978150356, 4.500000000000001776 ) ) ;
#1531=CARTESIAN_POINT ( 'NONE',  ( 2.392413149609226686, 188.9999999999999716, 7.742749228504306025 ) ) ;
#1538=CARTESIAN_POINT ( 'NONE',  ( -1.767766952966369765, 186.7999999978150356, 8.767766952966368876 ) ) ;
#1543=CARTESIAN_POINT ( 'NONE',  ( -2.500000000000000444, 185.2199999975965738, 8.035533905932737753 ) ) ;
#1544=CARTESIAN_POINT ( 'NONE',  ( 0.8818167416564541838, 227.6759890937897239, 5.303628879260831042 ) ) ;
#1545=CARTESIAN_POINT ( 'NONE',  ( -1.104351905119298705, 226.3927175376774699, 4.685770134608635118 ) ) ;
#1546=CARTESIAN_POINT ( 'NONE',  ( -1.934526094385236483, 189.7531569016572632, 9.674728188581434907 ) ) ;
#1547=B_SPLINE_CURVE_WITH_KNOTS ( 'NONE', 3,
 ( #15097, #11740, #843, #5708, #10551 ),
 .UNSPECIFIED., .F., .F.,
 ( 4, 1, 4 ),
 ( 0.7688659053744423266, 0.7708896602024635225, 0.7729134150304846074 ),
 .UNSPECIFIED. ) ;
#1553=CARTESIAN_POINT ( 'NONE',  ( 2.968835193067500988, 227.4419886495170715, 7.776466547877070923 ) ) ;
#1560=CARTESIAN_POINT ( 'NONE',  ( -1.767766952966369098, 185.0999999999999943, 5.232233047033630235 ) ) ;
#1562=CARTESIAN_POINT ( 'NONE',  ( -1.454198809819935878, 227.8150368499753995, 5.705206729889046535 ) ) ;
#1567=CARTESIAN_POINT ( 'NONE',  ( 2.066987300000000083, 188.2999999989075093, 6.143825827087054492 ) ) ;
#1569=CARTESIAN_POINT ( 'NONE',  ( -1.461580736456473462, 188.1499999989075320, 8.461580736456472351 ) ) ;
#1572=CARTESIAN_POINT ( 'NONE',  ( 1.767766952966368432, 186.9999999978150527, 8.767766952966368876 ) ) ;
#1573=CARTESIAN_POINT ( 'NONE',  ( 3.659182332138577465E-16, 221.4150671951173308, 6.196499129422101682 ) ) ;
#1576=CARTESIAN_POINT ( 'NONE',  ( 1.447897648385842562, 188.9999999996366569, 4.953942678156875168 ) ) ;
#1578=CARTESIAN_POINT ( 'NONE',  ( 1.410416696976425799, 190.0533888663666175, 4.554553427631445217 ) ) ;
#1583=CARTESIAN_POINT ( 'NONE',  ( 2.066987300000000083, 186.8499999989075206, 7.000000000000000000 ) ) ;
#1590=ORIENTED_EDGE ( 'NONE', *, *, #15629, .T. ) ;
#1593=CARTESIAN_POINT ( 'NONE',  ( -2.986011043896227513, 189.8622845448325052, 7.656297732253541710 ) ) ;
#1606=CARTESIAN_POINT ( 'NONE',  ( 0.2265647687538700217, 188.9999999999999716, 9.493607779905927302 ) ) ;
#1614=CARTESIAN_POINT ( 'NONE',  ( -2.500000000000000444, 186.6999999978150697, 7.000000000000000000 ) ) ;
#1619=CARTESIAN_POINT ( 'NONE',  ( -2.500000000000000444, 186.0199999975965568, 8.035533905932737753 ) ) ;
#1620=CARTESIAN_POINT ( 'NONE',  ( -1.212431555520800508, 228.7775460029053534, 8.484988061474600940 ) ) ;
#1621=CARTESIAN_POINT ( 'NONE',  ( -2.191511056945971259, 226.6300844452854903, 5.385369267317587472 ) ) ;
#1623=CARTESIAN_POINT ( 'NONE',  ( -2.353560662074906773, 189.1623160119228544, 9.042440134401656948 ) ) ;
#1627=EDGE_CURVE ( 'NONE', #1738, #3723, #666, .T. ) ;
#1631=CARTESIAN_POINT ( 'NONE',  ( 2.988911113477941583, 227.2040587690521534, 7.075956526733278018 ) ) ;
#1634=CARTESIAN_POINT ( 'NONE',  ( -2.500000000000001776, 188.4500000000000171, 8.035533905932737753 ) ) ;
#1635=CARTESIAN_POINT ( 'NONE',  ( 2.500000000000000444, 185.5500000000000114, 8.035533905932739529 ) ) ;
#1638=CARTESIAN_POINT ( 'NONE',  ( 0.8818167416564541838, 227.6759890937897239, 5.303628879260831042 ) ) ;
#1643=CARTESIAN_POINT ( 'NONE',  ( -2.066987300000001415, 187.7999999989075093, 6.143825827087054492 ) ) ;
#1645=CARTESIAN_POINT ( 'NONE',  ( 2.066987299999999195, 188.3999999989075320, 7.856174172912946396 ) ) ;
#1651=DIRECTION ( 'NONE',  ( 1.000000000000000000, 0.000000000000000000, 0.000000000000000000 ) ) ;
#1652=CARTESIAN_POINT ( 'NONE',  ( 1.292454554785913867, 188.9999999995436610, 9.144800990124029028 ) ) ;
#1653=CARTESIAN_POINT ( 'NONE',  ( -2.500000000000000888, 188.2999999978150356, 7.000000000000000000 ) ) ;
#1660=CARTESIAN_POINT ( 'NONE',  ( -1.084202172485504434E-16, 187.8499999989074922, 4.933012699999999029 ) ) ;
#1661=AXIS2_PLACEMENT_3D ( 'NONE', #4362, #10562, #11676 ) ;
#1665=LINE ( 'NONE', #12794, #2767 ) ;
#1671=CARTESIAN_POINT ( 'NONE',  ( 1.461580736456472351, 189.1499999989075320, 8.461580736456474128 ) ) ;
#1684=ORIENTED_EDGE ( 'NONE', *, *, #2925, .F. ) ;
#1689=CARTESIAN_POINT ( 'NONE',  ( 1.035533905932738419, 185.3499999978151038, 9.500000000000003553 ) ) ;
#1694=CARTESIAN_POINT ( 'NONE',  ( -1.767766952966369098, 185.8699999975965511, 5.232233047033630235 ) ) ;
#1695=CARTESIAN_POINT ( 'NONE',  ( 1.057043591443594943, 228.1937260751906820, 9.987734910156856216 ) ) ;
#1696=CARTESIAN_POINT ( 'NONE',  ( -1.585166063744550602, 226.4701105292460568, 4.913902397277155387 ) ) ;
#1711=CARTESIAN_POINT ( 'NONE',  ( -2.500000000000000888, 187.5999999999999943, 7.000000000000000000 ) ) ;
#1714=CARTESIAN_POINT ( 'NONE',  ( -0.7328022267957914337, 227.6546247107034446, 5.241927322362504249 ) ) ;
#1719=CARTESIAN_POINT ( 'NONE',  ( -2.066987300000000971, 187.8499999989074922, 7.000000000000000000 ) ) ;
#1722=CARTESIAN_POINT ( 'NONE',  ( -2.066987300000000083, 187.1999999989075434, 6.143825827087054492 ) ) ;
#1727=CARTESIAN_POINT ( 'NONE',  ( 0.000000000000000000, 185.8606548077538321, 9.048340948986950849 ) ) ;
#1729=CARTESIAN_POINT ( 'NONE',  ( 1.382634503510036250, 189.0823306087117430, 9.850504157829032437 ) ) ;
#1732=CARTESIAN_POINT ( 'NONE',  ( 2.866460994376960336, 189.9235028716541933, 6.357051353814127559 ) ) ;
#1733=VECTOR ( 'NONE', #8292, 1000.000000000000000 ) ;
#1738=VERTEX_POINT ( 'NONE', #10723 ) ;
#1739=CARTESIAN_POINT ( 'NONE',  ( -0.8561741729129455081, 186.2999999989075093, 4.933012699999999029 ) ) ;
#1770=CARTESIAN_POINT ( 'NONE',  ( 2.500000000000000444, 187.1499999978150868, 5.964466094067262247 ) ) ;
#1771=CIRCLE ( 'NONE', #763, 1.000000000000000444 ) ;
#1772=CARTESIAN_POINT ( 'NONE',  ( -1.035533905932737753, 184.9499999978150413, 4.500000000000001776 ) ) ;
#1776=CARTESIAN_POINT ( 'NONE',  ( 2.255245247391631569, 227.9269692368775395, 9.203290779546277278 ) ) ;
#1777=CARTESIAN_POINT ( 'NONE',  ( -1.979540121751099724, 226.5646310999674427, 5.192482286045976281 ) ) ;
#1782=CARTESIAN_POINT ( 'NONE',  ( -2.500000000000000444, 189.0500374527063343, 5.965241810263807842 ) ) ;
#1785=CARTESIAN_POINT ( 'NONE',  ( 2.174380334507205248, 227.9547525935562646, 9.285006124859036092 ) ) ;
#1791=CARTESIAN_POINT ( 'NONE',  ( 1.767766952966369320, 185.7000000000000171, 5.232233047033630235 ) ) ;
#1792=CARTESIAN_POINT ( 'NONE',  ( -1.914314807121730633, 228.0813985855225212, 6.474474614426593888 ) ) ;
#1797=CARTESIAN_POINT ( 'NONE',  ( 2.500000000000000444, 185.6500000000000341, 5.964466094067262247 ) ) ;
#1799=CARTESIAN_POINT ( 'NONE',  ( 2.066987299999999639, 186.7999999989075093, 7.856174172912946396 ) ) ;
#1807=CARTESIAN_POINT ( 'NONE',  ( 2.989629975077807256, 189.8928756713021357, 6.972882067819393015 ) ) ;
#1811=CARTESIAN_POINT ( 'NONE',  ( 1.813601955701626300, 228.5298646585827385, 7.769670212251800656 ) ) ;
#1816=CARTESIAN_POINT ( 'NONE',  ( -5.285485590866834116E-16, 186.4499999989075150, 9.066987300000000971 ) ) ;
#1826=( BOUNDED_CURVE ( )  B_SPLINE_CURVE ( 2, ( #10332, #15186, #11209, #4283, #3089, #8836, #7632, #1499, #1653 ),
 .UNSPECIFIED., .F., .F. ) 
 B_SPLINE_CURVE_WITH_KNOTS ( ( 3, 2, 2, 2, 3 ),
 ( 0.5714285714285713969, 0.5892857142857143016, 0.6071428571428570953, 0.6250000000000000000, 0.6428571428571429047 ),
 .UNSPECIFIED. ) 
 CURVE ( )  GEOMETRIC_REPRESENTATION_ITEM ( )  RATIONAL_B_SPLINE_CURVE ( ( 1.000000000000000000, 0.9238795325112867385, 1.000000000000000000, 0.9238795325112867385, 1.000000000000000000, 0.9238795325112867385, 1.000000000000000000, 0.9238795325112867385, 1.000000000000000000 ) ) 
 REPRESENTATION_ITEM ( '' )  );
#1831=CARTESIAN_POINT ( 'NONE',  ( -2.500000000000000444, 186.7999999999999829, 7.000000000000000000 ) ) ;
#1844=CARTESIAN_POINT ( 'NONE',  ( 1.767766952966368432, 187.7999999978150356, 8.767766952966368876 ) ) ;
#1845=CARTESIAN_POINT ( 'NONE',  ( -1.035533905932739751, 189.2499999978150811, 9.500000000000003553 ) ) ;
#1851=CARTESIAN_POINT ( 'NONE',  ( -1.035533905932739751, 189.3199999975965682, 9.500000000000003553 ) ) ;
#1852=CARTESIAN_POINT ( 'NONE',  ( -0.6401557763822781633, 228.8776351522889172, 8.774051233606112277 ) ) ;
#1859=ORIENTED_EDGE ( 'NONE', *, *, #3113, .F. ) ;
#1864=LINE ( 'NONE', #3218, #4114 ) ;
#1870=CARTESIAN_POINT ( 'NONE',  ( -1.035533905932739529, 186.0499999978150356, 9.500000000000003553 ) ) ;
#1871=CARTESIAN_POINT ( 'NONE',  ( 0.5489208960863538600, 227.6341400683239726, 5.182766506802777506 ) ) ;
#1875=CARTESIAN_POINT ( 'NONE',  ( -1.035533905932737975, 185.8500000000000227, 4.500000000000000888 ) ) ;
#1881=AXIS2_PLACEMENT_3D ( 'NONE', #7229, #12222, #14622 ) ;
#1883=CARTESIAN_POINT ( 'NONE',  ( -1.898822140593172669, 189.7510425599547261, 9.704729509603533089 ) ) ;
#1886=CARTESIAN_POINT ( 'NONE',  ( -4.912791094074941967E-16, 184.5300000002184788, 9.500000000000001776 ) ) ;
#1888=CARTESIAN_POINT ( 'NONE',  ( 0.06495987523896813720, 228.9118724015956730, 8.872930362369002566 ) ) ;
#1892=EDGE_LOOP ( 'NONE', ( #8151, #8211, #9561, #6789 ) ) ;
#1893=CARTESIAN_POINT ( 'NONE',  ( 1.461580736456473462, 185.1499999989075320, 5.538419263543526760 ) ) ;
#1895=CARTESIAN_POINT ( 'NONE',  ( 2.500000000000000444, 184.7500000000000000, 8.035533905932739529 ) ) ;
#1900=CARTESIAN_POINT ( 'NONE',  ( -2.066987300000000083, 184.7999999989075093, 6.143825827087054492 ) ) ;
#1902=CARTESIAN_POINT ( 'NONE',  ( -2.066987300000000527, 184.6499999989075320, 7.000000000000000000 ) ) ;
#1907=CARTESIAN_POINT ( 'NONE',  ( 0.000000000000000000, 201.6409668649146738, 13.30942870683726298 ) ) ;
#1924=CARTESIAN_POINT ( 'NONE',  ( 2.500000000000000000, 188.6499999978150584, 8.035533905932739529 ) ) ;
#1929=CARTESIAN_POINT ( 'NONE',  ( -1.524659305057740610E-16, 188.9699999975965738, 4.500000000000000000 ) ) ;
#1930=CARTESIAN_POINT ( 'NONE',  ( -1.864336199031810581, 228.4898043637318779, 7.653973795834509097 ) ) ;
#1939=ORIENTED_EDGE ( 'NONE', *, *, #7499, .F. ) ;
#1944=CYLINDRICAL_SURFACE ( 'NONE', #14809, 2.500000000000000444 ) ;
#1949=CARTESIAN_POINT ( 'NONE',  ( 1.767766952966368654, 185.3999999978150584, 8.767766952966368876 ) ) ;
#1950=CARTESIAN_POINT ( 'NONE',  ( -1.990689658724532629, 228.2709309767465697, 7.021854970500988280 ) ) ;
#1954=CARTESIAN_POINT ( 'NONE',  ( -2.500000000000000444, 186.7999999999999829, 7.000000000000000000 ) ) ;
#1962=CARTESIAN_POINT ( 'NONE',  ( -2.977464457213339077, 189.8978568417799693, 6.866500699578031330 ) ) ;
#1963=CARTESIAN_POINT ( 'NONE',  ( 0.07162629256299407610, 188.9999999999999716, 4.501026275805653398 ) ) ;
#1964=CARTESIAN_POINT ( 'NONE',  ( -1.767766952966369098, 185.0300000002184788, 5.232233047033630235 ) ) ;
#1965=CARTESIAN_POINT ( 'NONE',  ( -1.739397458836472676, 227.9323402172746853, 6.043985545194606956 ) ) ;
#1966=CARTESIAN_POINT ( 'NONE',  ( 1.923823996436629047, 228.4292023995385250, 7.478951866735841669 ) ) ;
#1971=CARTESIAN_POINT ( 'NONE',  ( -1.461580736456473906, 186.3499999989074922, 8.461580736456474128 ) ) ;
#1973=CARTESIAN_POINT ( 'NONE',  ( -1.035533905932739529, 184.5499999999999829, 9.500000000000000000 ) ) ;
#1982=CARTESIAN_POINT ( 'NONE',  ( 1.461580736456472795, 184.9499999989075150, 8.461580736456474128 ) ) ;
#1987=CARTESIAN_POINT ( 'NONE',  ( 5.999999999999999112, 221.4150671951173592, 6.196499129422101682 ) ) ;
#1990=LINE ( 'NONE', #7015, #12015 ) ;
#1992=ORIENTED_EDGE ( 'NONE', *, *, #488, .T. ) ;
#1995=CARTESIAN_POINT ( 'NONE',  ( 3.659182332138073087E-16, 190.0875178197511275, 4.201689379953569947 ) ) ;
#2002=CARTESIAN_POINT ( 'NONE',  ( -1.461580736456473240, 184.9499999989075150, 8.461580736456472351 ) ) ;
#2005=CARTESIAN_POINT ( 'NONE',  ( 2.283493650000000486, 184.1249999994537632, 7.000000000000000000 ) ) ;
#2009=CARTESIAN_POINT ( 'NONE',  ( 2.809728313654571430, 226.9499418402095046, 6.327683296853605199 ) ) ;
#2025=CARTESIAN_POINT ( 'NONE',  ( 1.035533905932738197, 187.8500000000000227, 9.500000000000003553 ) ) ;
#2027=CARTESIAN_POINT ( 'NONE',  ( -1.964265005259087538, 228.3667458257928047, 7.298573719466742382 ) ) ;
#2032=CARTESIAN_POINT ( 'NONE',  ( -5.421010862427522170E-17, 187.4000000000000057, 4.500000000000000000 ) ) ;
#2036=EDGE_CURVE ( 'NONE', #7505, #5259, #3571, .T. ) ;
#2040=CARTESIAN_POINT ( 'NONE',  ( -3.000003100478683571, 227.2950289990915564, 7.343811503137294139 ) ) ;
#2041=( LENGTH_UNIT ( ) NAMED_UNIT ( * ) SI_UNIT ( .MILLI., .METRE. ) );
#2044=CARTESIAN_POINT ( 'NONE',  ( 9.486769009248163798E-17, 184.9300000002185129, 4.500000000000000000 ) ) ;
#2045=CARTESIAN_POINT ( 'NONE',  ( -1.926973947205288917, 228.4293926868652136, 7.479501427387623913 ) ) ;
#2046=CARTESIAN_POINT ( 'NONE',  ( 1.498060502294345175, 227.8308734224802095, 5.750943654540091821 ) ) ;
#2051=CARTESIAN_POINT ( 'NONE',  ( -2.066987300000000971, 188.7999999989075093, 6.143825827087054492 ) ) ;
#2056=CARTESIAN_POINT ( 'NONE',  ( 2.066987300000000083, 185.2999999989075377, 6.143825827087054492 ) ) ;
#2058=CARTESIAN_POINT ( 'NONE',  ( 2.066987300000000527, 187.4999999989075263, 6.143825827087054492 ) ) ;
#2062=B_SPLINE_CURVE_WITH_KNOTS ( 'NONE', 3,
 ( #7636, #8840, #3888, #10029, #388, #12560, #11291, #5258 ),
 .UNSPECIFIED., .F., .F.,
 ( 4, 2, 2, 4 ),
 ( 0.7729134150304844963, 0.8008314270218360731, 0.8287494390131875388, 0.8845854629958906923 ),
 .UNSPECIFIED. ) ;
#2063=CARTESIAN_POINT ( 'NONE',  ( 0.000000000000000000, 201.6409668649146738, 13.30942870683726298 ) ) ;
#2072=CARTESIAN_POINT ( 'NONE',  ( 0.8561741729129455081, 186.1999999989075150, 4.933012699999999029 ) ) ;
#2079=CARTESIAN_POINT ( 'NONE',  ( 0.8561741729129456191, 184.5999999989075206, 4.933012699999999029 ) ) ;
#2082=CARTESIAN_POINT ( 'NONE',  ( 1.767766952966369098, 188.8999999999999773, 5.232233047033630235 ) ) ;
#2085=CARTESIAN_POINT ( 'NONE',  ( 0.8272382227408706656, 226.3624115040579738, 4.596429122765971265 ) ) ;
#2104=CARTESIAN_POINT ( 'NONE',  ( 1.767766952966369320, 186.3999999978150584, 5.232233047033630235 ) ) ;
#2106=CARTESIAN_POINT ( 'NONE',  ( 1.237590631448066469, 228.1696616696178808, 9.916980740552745033 ) ) ;
#2111=CARTESIAN_POINT ( 'NONE',  ( -1.035533905932737975, 188.2500000000000000, 4.500000000000000888 ) ) ;
#2120=CARTESIAN_POINT ( 'NONE',  ( 1.035533905932737975, 185.6800000002185129, 4.500000000000000888 ) ) ;
#2122=CARTESIAN_POINT ( 'NONE',  ( 1.454231928715901123, 227.8150477629479269, 5.705238247175231869 ) ) ;
#2127=CARTESIAN_POINT ( 'NONE',  ( 0.8561741729129461742, 185.6999999989075434, 9.066987300000000971 ) ) ;
#2134=CARTESIAN_POINT ( 'NONE',  ( -2.066987300000000971, 187.7999999989075093, 6.143825827087054492 ) ) ;
#2138=CARTESIAN_POINT ( 'NONE',  ( 5.999999999999999112, 187.9952603975225429, 3.440894205938198613 ) ) ;
#2143=ORIENTED_EDGE ( 'NONE', *, *, #2200, .F. ) ;
#2154=CARTESIAN_POINT ( 'NONE',  ( -1.461580736456472795, 184.7499999989074979, 5.538419263543527649 ) ) ;
#2160=CARTESIAN_POINT ( 'NONE',  ( 2.961265621965179395, 227.4473031124620377, 7.792030372366526514 ) ) ;
#2163=CARTESIAN_POINT ( 'NONE',  ( -1.035533905932739529, 186.0499999978150356, 9.500000000000000000 ) ) ;
#2170=CARTESIAN_POINT ( 'NONE',  ( -5.454892180317694184E-16, 185.4000000000000057, 9.500000000000001776 ) ) ;
#2179=CARTESIAN_POINT ( 'NONE',  ( 2.500000000000000444, 188.0500000000000114, 5.964466094067262247 ) ) ;
#2180=ADVANCED_FACE ( 'NONE', ( #2774 ), #3877, .T. ) ;
#2181=CARTESIAN_POINT ( 'NONE',  ( -1.212431555520800508, 228.7775460029053534, 8.484988061474600940 ) ) ;
#2183=CARTESIAN_POINT ( 'NONE',  ( -0.1126307680551840440, 188.9999999999637623, 4.495745018146146244 ) ) ;
#2194=CARTESIAN_POINT ( 'NONE',  ( -2.175328470913686196, 226.6252516911083603, 5.371125302583743988 ) ) ;
#2198=CARTESIAN_POINT ( 'NONE',  ( -5.895349312889930360E-16, 186.1300000002185016, 9.500000000000001776 ) ) ;
#2200=EDGE_CURVE ( 'NONE', #2929, #7504, #330, .T. ) ;
#2202=CARTESIAN_POINT ( 'NONE',  ( -1.618809023786734747, 227.8806835185142461, 5.894798052868548410 ) ) ;
#2208=CARTESIAN_POINT ( 'NONE',  ( -1.965116437629976787E-16, 189.2499999989075263, 4.933012699999999029 ) ) ;
#2215=CARTESIAN_POINT ( 'NONE',  ( -0.8561741729129457301, 186.0999999989074922, 4.933012699999999029 ) ) ;
#2219=CARTESIAN_POINT ( 'NONE',  ( 0.000000000000000000, 187.2933328889893687, 9.583808270834989429 ) ) ;
#2227=EDGE_LOOP ( 'NONE', ( #15670, #11895 ) ) ;
#2229=CARTESIAN_POINT ( 'NONE',  ( 1.583819872848719834, 227.8634474321731034, 5.845019252434271451 ) ) ;
#2235=CARTESIAN_POINT ( 'NONE',  ( -2.066987300000000527, 188.0499999989075093, 7.000000000000000000 ) ) ;
#2242=CARTESIAN_POINT ( 'NONE',  ( 2.856278104602718138, 227.5851434513726019, 8.197675965640897289 ) ) ;
#2253=CARTESIAN_POINT ( 'NONE',  ( -1.035533905932739529, 185.3499999999999943, 9.500000000000000000 ) ) ;
#2262=CARTESIAN_POINT ( 'NONE',  ( -2.500000000000000444, 186.6499999978150299, 5.964466094067261359 ) ) ;
#2263=CARTESIAN_POINT ( 'NONE',  ( 0.1954887924997270876, 228.2535971796124556, 10.16375797564445804 ) ) ;
#2265=CARTESIAN_POINT ( 'NONE',  ( -1.815566070620405315, 190.0296528384676549, 4.819757843237718831 ) ) ;
#2274=CARTESIAN_POINT ( 'NONE',  ( 2.363901779514900880, 226.6922819415928245, 5.568617383738656557 ) ) ;
#2278=CARTESIAN_POINT ( 'NONE',  ( -1.485687618429907486, 226.4511214500596168, 4.857910484922783212 ) ) ;
#2281=CARTESIAN_POINT ( 'NONE',  ( 1.767766952966368432, 187.0300000002185072, 8.767766952966368876 ) ) ;
#2283=CARTESIAN_POINT ( 'NONE',  ( -1.361823383409473953, 227.7851450847494448, 5.618877607002349173 ) ) ;
#2288=CARTESIAN_POINT ( 'NONE',  ( 1.461580736456472795, 185.7499999989074979, 8.461580736456474128 ) ) ;
#2297=CARTESIAN_POINT ( 'NONE',  ( -1.461580736456473906, 187.9499999989075150, 8.461580736456474128 ) ) ;
#2302=CARTESIAN_POINT ( 'NONE',  ( -1.768703179866833342, 189.0000639513403939, 5.233169770031948609 ) ) ;
#2308=ORIENTED_EDGE ( 'NONE', *, *, #15367, .T. ) ;
#2309=CARTESIAN_POINT ( 'NONE',  ( 1.938829455441115623, 228.0900040983942745, 6.499327826426426924 ) ) ;
#2315=CARTESIAN_POINT ( 'NONE',  ( -2.066987300000000083, 187.1999999989075434, 6.143825827087054492 ) ) ;
#2319=DIRECTION ( 'NONE',  ( -6.123233995736766036E-17, 1.000000000000000000, 0.000000000000000000 ) ) ;
#2320=CARTESIAN_POINT ( 'NONE',  ( -0.9181233697252281223, 226.3712865412501003, 4.622592831843514993 ) ) ;
#2321=CARTESIAN_POINT ( 'NONE',  ( 2.500000000000000444, 187.2000000000000171, 7.000000000000000000 ) ) ;
#2326=VERTEX_POINT ( 'NONE', #611 ) ;
#2327=ORIENTED_EDGE ( 'NONE', *, *, #5021, .F. ) ;
#2344=CARTESIAN_POINT ( 'NONE',  ( 1.767766952966368432, 186.9999999978150527, 8.767766952966368876 ) ) ;
#2345=CARTESIAN_POINT ( 'NONE',  ( 2.976061188595913176, 227.1638826975962502, 6.957706536906315797 ) ) ;
#2349=ORIENTED_EDGE ( 'NONE', *, *, #11851, .F. ) ;
#2360=CARTESIAN_POINT ( 'NONE',  ( -2.773146674828778302, 226.9215239162201669, 6.243979701131443072 ) ) ;
#2362=CARTESIAN_POINT ( 'NONE',  ( 2.500000000000000000, 188.7300000002184959, 7.000000000000000000 ) ) ;
#2363=CARTESIAN_POINT ( 'NONE',  ( -2.940898392866930777E-15, 228.9118723800512498, 8.872930300147352511 ) ) ;
#2364=CARTESIAN_POINT ( 'NONE',  ( -1.454198809819935878, 227.8150368499753995, 5.705206729889046535 ) ) ;
#2365=CARTESIAN_POINT ( 'NONE',  ( 1.895314869936763680, 228.4599366835234093, 7.567714231851713436 ) ) ;
#2369=CARTESIAN_POINT ( 'NONE',  ( -2.066987300000001415, 187.7999999989075093, 6.143825827087054492 ) ) ;
#2370=CARTESIAN_POINT ( 'NONE',  ( -2.066987300000000971, 185.3999999989075604, 6.143825827087054492 ) ) ;
#2379=CARTESIAN_POINT ( 'NONE',  ( 0.8561741729129461742, 186.4999999989074695, 9.066987300000000971 ) ) ;
#2383=CARTESIAN_POINT ( 'NONE',  ( 2.500000000000000444, 184.0499999999999829, 5.964466094067262247 ) ) ;
#2389=EDGE_LOOP ( 'NONE', ( #13309, #7223, #2539, #4850 ) ) ;
#2396=CARTESIAN_POINT ( 'NONE',  ( 1.461580736456472351, 186.7499999989075263, 8.461580736456474128 ) ) ;
#2404=CARTESIAN_POINT ( 'NONE',  ( -1.238695443643032412, 228.1695118093442716, 9.916540120957755278 ) ) ;
#2406=VERTEX_POINT ( 'NONE', #33 ) ;
#2407=ORIENTED_EDGE ( 'NONE', *, *, #15632, .T. ) ;
#2409=CARTESIAN_POINT ( 'NONE',  ( 1.767766952966368654, 186.1999999978150697, 8.767766952966368876 ) ) ;
#2423=CARTESIAN_POINT ( 'NONE',  ( -2.500000000000000444, 187.5499999978150356, 8.035533905932737753 ) ) ;
#2424=CARTESIAN_POINT ( 'NONE',  ( 2.843216347914732101, 226.9801049014886587, 6.416521247196312672 ) ) ;
#2427=EDGE_CURVE ( 'NONE', #13484, #14260, #6091, .T. ) ;
#2428=CARTESIAN_POINT ( 'NONE',  ( -2.276077516478379525, 188.9999999996472866, 5.950350810759988285 ) ) ;
#2433=ADVANCED_FACE ( 'NONE', ( #14677 ), #9904, .T. ) ;
#2434=CARTESIAN_POINT ( 'NONE',  ( -6.911788849595090767E-16, 187.7999999999999829, 9.500000000000001776 ) ) ;
#2437=FACE_OUTER_BOUND ( 'NONE', #2227, .T. ) ;
#2444=CARTESIAN_POINT ( 'NONE',  ( 2.500000000000000444, 184.0500000000000114, 5.964466094067262247 ) ) ;
#2446=CARTESIAN_POINT ( 'NONE',  ( 1.312858199469658427, 228.7505821040874139, 8.407114783769989330 ) ) ;
#2452=CARTESIAN_POINT ( 'NONE',  ( -6.268043809681822509E-16, 188.0499999989075093, 9.066987300000000971 ) ) ;
#2453=CARTESIAN_POINT ( 'NONE',  ( 2.066987300000000527, 185.0499999989075093, 7.000000000000000000 ) ) ;
#2454=CARTESIAN_POINT ( 'NONE',  ( -1.965116437629976787E-16, 189.2499999989075263, 4.933012699999999029 ) ) ;
#2460=CARTESIAN_POINT ( 'NONE',  ( 0.000000000000000000, 186.5669965222008386, 9.317226423031119253 ) ) ;
#2461=CARTESIAN_POINT ( 'NONE',  ( -2.066987300000001415, 188.6999999989075150, 7.856174172912944620 ) ) ;
#2468=( BOUNDED_CURVE ( )  B_SPLINE_CURVE ( 2, ( #14032, #1782, #4490, #3141, #11647, #12915, #7993, #749, #4256, #11488, #5614, #7837, #4176, #12685, #4417 ),
 .UNSPECIFIED., .F., .F. ) 
 B_SPLINE_CURVE_WITH_KNOTS ( ( 3, 2, 2, 2, 2, 2, 2, 3 ),
 ( 0.7678695020645334157, 0.7857142857142856984, 0.8035714285714286031, 0.8214285714285713969, 0.8392857142857143016, 0.8571428571428570953, 0.8750000000000000000, 0.8928571428571429047 ),
 .UNSPECIFIED. ) 
 CURVE ( )  GEOMETRIC_REPRESENTATION_ITEM ( )  RATIONAL_B_SPLINE_CURVE ( ( 0.9998947045988972882, 0.9239322166753706211, 1.000000000000000000, 0.9238795325112867385, 1.000000000000000000, 0.9238795325112867385, 1.000000000000000000, 0.9238795325112867385, 1.000000000000000000, 0.9238795325112867385, 1.000000000000000000, 0.9238795325112867385, 1.000000000000000000, 0.9238795325112867385, 1.000000000000000000 ) ) 
 REPRESENTATION_ITEM ( '' )  );
#2473=ORIENTED_EDGE ( 'NONE', *, *, #2427, .F. ) ;
#2482=CARTESIAN_POINT ( 'NONE',  ( -1.461580736456473018, 187.1499999989075320, 5.538419263543527649 ) ) ;
#2489=CARTESIAN_POINT ( 'NONE',  ( -2.995192278888715975, 227.2265329420484647, 7.142163989385624134 ) ) ;
#2496=CARTESIAN_POINT ( 'NONE',  ( 0.9085682363223165359, 189.0000000000000000, 9.333306381406472951 ) ) ;
#2502=UNCERTAINTY_MEASURE_WITH_UNIT (LENGTH_MEASURE( 1.000000000000000082E-05 ), #2041, 'distance_accuracy_value', 'NONE');
#2507=CARTESIAN_POINT ( 'NONE',  ( -2.500000000000000888, 188.3999999999999773, 7.000000000000000000 ) ) ;
#2511=CARTESIAN_POINT ( 'NONE',  ( 2.500000000000000444, 187.8499999978150470, 8.035533905932739529 ) ) ;
#2513=CARTESIAN_POINT ( 'NONE',  ( 2.961752869269595134, 227.1327854310254111, 6.866142280206398496 ) ) ;
#2515=CARTESIAN_POINT ( 'NONE',  ( -0.8793070671816629602, 189.7084256268280456, 10.26238677585280179 ) ) ;
#2521=CARTESIAN_POINT ( 'NONE',  ( 1.129999918305732987, 226.3961343599838756, 4.695842443849920222 ) ) ;
#2526=CARTESIAN_POINT ( 'NONE',  ( 1.035533905932738197, 187.7800000002184788, 9.500000000000003553 ) ) ;
#2529=CARTESIAN_POINT ( 'NONE',  ( 1.814481968427068992, 227.9916212483514641, 6.215192544112370321 ) ) ;
#2533=ORIENTED_EDGE ( 'NONE', *, *, #557, .T. ) ;
#2534=CARTESIAN_POINT ( 'NONE',  ( 2.066987300000000083, 187.3999999989075320, 7.856174172912946396 ) ) ;
#2536=CARTESIAN_POINT ( 'NONE',  ( 0.8561741729129461742, 184.8999999989075320, 9.066987300000000971 ) ) ;
#2539=ORIENTED_EDGE ( 'NONE', *, *, #6410, .F. ) ;
#2543=CARTESIAN_POINT ( 'NONE',  ( 5.999999999999999112, 215.7452399395091618, 13.29567785264566027 ) ) ;
#2544=CARTESIAN_POINT ( 'NONE',  ( -2.369853004795346330, 188.9999999999999716, 6.157114161223693038 ) ) ;
#2555=ORIENTED_EDGE ( 'NONE', *, *, #7831, .F. ) ;
#2556=DIRECTION ( 'NONE',  ( -6.123233995736766036E-17, 1.000000000000000000, 0.000000000000000000 ) ) ;
#2561=CARTESIAN_POINT ( 'NONE',  ( 1.461580736456472351, 188.3499999989074922, 8.461580736456474128 ) ) ;
#2567=CARTESIAN_POINT ( 'NONE',  ( -2.842171547016528965, 226.9791356524935395, 6.413666598675894726 ) ) ;
#2584=CARTESIAN_POINT ( 'NONE',  ( -1.456896669277396583E-16, 188.8999999978150584, 4.500000000000000000 ) ) ;
#2585=CARTESIAN_POINT ( 'NONE',  ( 2.923766376317260551, 227.0711491207812855, 6.684645050985161596 ) ) ;
#2587=CARTESIAN_POINT ( 'NONE',  ( -0.4847600579890295469, 189.7005989459862860, 10.35649496429148897 ) ) ;
#2598=CARTESIAN_POINT ( 'NONE',  ( -2.500000000000000888, 187.5300000002185072, 7.000000000000000000 ) ) ;
#2601=CARTESIAN_POINT ( 'NONE',  ( 0.06495987523896813720, 228.9118724015956730, 8.872930362369002566 ) ) ;
#2608=CARTESIAN_POINT ( 'NONE',  ( -2.066987300000000971, 184.5999999989074922, 6.143825827087054492 ) ) ;
#2618=CARTESIAN_POINT ( 'NONE',  ( 0.000000000000000000, 215.7452399395091049, 13.29567785264566027 ) ) ;
#2619=CARTESIAN_POINT ( 'NONE',  ( 0.8561741729129458411, 188.8999999989075320, 9.066987300000000971 ) ) ;
#2628=CARTESIAN_POINT ( 'NONE',  ( -1.461580736456473462, 187.3499999989075206, 8.461580736456472351 ) ) ;
#2629=ADVANCED_FACE ( 'NONE', ( #9885 ), #6153, .T. ) ;
#2638=CARTESIAN_POINT ( 'NONE',  ( -1.735141101668105090, 228.0777902684043852, 9.646862769529031212 ) ) ;
#2648=CARTESIAN_POINT ( 'NONE',  ( -1.747606509155581689, 226.5054486174500994, 5.018058692477180394 ) ) ;
#2658=CARTESIAN_POINT ( 'NONE',  ( -5.861467994999758346E-16, 186.0999999978150754, 9.500000000000001776 ) ) ;
#2663=CARTESIAN_POINT ( 'NONE',  ( 1.767766952966369098, 187.2699999975965568, 5.232233047033630235 ) ) ;
#2664=CARTESIAN_POINT ( 'NONE',  ( -1.786743523428754976, 227.9724114945277051, 6.159713679416685572 ) ) ;
#2665=CARTESIAN_POINT ( 'NONE',  ( -2.809592974547592714, 227.6294044507834542, 8.327915135215583575 ) ) ;
#2668=CARTESIAN_POINT ( 'NONE',  ( -1.830453387431577816, 189.0000000012350938, 8.709453706375219539 ) ) ;
#2674=CARTESIAN_POINT ( 'NONE',  ( 2.903473946076591705, 227.5344354822965443, 8.048524736755723552 ) ) ;
#2680=CARTESIAN_POINT ( 'NONE',  ( 1.767766952966369098, 186.5000000000000000, 5.232233047033630235 ) ) ;
#2686=CARTESIAN_POINT ( 'NONE',  ( -6.776263578034402713E-16, 188.8499999989074922, 9.066987300000000971 ) ) ;
#2689=CARTESIAN_POINT ( 'NONE',  ( -0.8561741729129467293, 186.5999999989075206, 9.066987299999999195 ) ) ;
#2695=( NAMED_UNIT ( * ) SI_UNIT ( $, .STERADIAN. ) SOLID_ANGLE_UNIT ( ) );
#2697=CARTESIAN_POINT ( 'NONE',  ( -6.776263578034402713E-16, 188.8499999989074922, 9.066987300000000971 ) ) ;
#2700=DIRECTION ( 'NONE',  ( -6.123233995736766036E-17, 1.000000000000000000, 0.000000000000000000 ) ) ;
#2701=CARTESIAN_POINT ( 'NONE',  ( 0.8628399698974030807, 190.0753276663367330, 4.324387286082350457 ) ) ;
#2707=CARTESIAN_POINT ( 'NONE',  ( -1.461580736456473462, 186.5499999989075093, 8.461580736456472351 ) ) ;
#2717=CARTESIAN_POINT ( 'NONE',  ( -1.839562682118536241, 190.0280088719464402, 4.838899882289354970 ) ) ;
#2718=CARTESIAN_POINT ( 'NONE',  ( -1.461580736456473462, 188.9499999989075150, 8.461580736456472351 ) ) ;
#2725=CARTESIAN_POINT ( 'NONE',  ( -1.748661130334981051, 228.0746845563984095, 9.637707355516731411 ) ) ;
#2726=ORIENTED_EDGE ( 'NONE', *, *, #10094, .T. ) ;
#2731=CARTESIAN_POINT ( 'NONE',  ( 2.208001385524885674, 189.0000000000000000, 8.182568187910820967 ) ) ;
#2737=CARTESIAN_POINT ( 'NONE',  ( -1.035533905932739751, 187.6499999978150584, 9.500000000000000000 ) ) ;
#2738=CARTESIAN_POINT ( 'NONE',  ( 2.500000000000000444, 185.4999999978150527, 7.000000000000000000 ) ) ;
#2744=CARTESIAN_POINT ( 'NONE',  ( 9.486769009248163798E-17, 184.9699999975965454, 4.500000000000000000 ) ) ;
#2745=CARTESIAN_POINT ( 'NONE',  ( -1.923034433439944513, 228.0917019039344495, 6.504231185664401949 ) ) ;
#2746=CARTESIAN_POINT ( 'NONE',  ( -1.978640506925948062, 228.0159251728749155, 9.464911921216582869 ) ) ;
#2748=CARTESIAN_POINT ( 'NONE',  ( -1.383648599222811360, 188.9999999995481517, 9.087128311603166253 ) ) ;
#2761=CARTESIAN_POINT ( 'NONE',  ( 2.500000000000000444, 184.7999999999999829, 7.000000000000000000 ) ) ;
#2763=CARTESIAN_POINT ( 'NONE',  ( -0.9962072163307928996, 227.6960174938032537, 5.361472040843871412 ) ) ;
#2767=VECTOR ( 'NONE', #7880, 1000.000000000000000 ) ;
#2768=CARTESIAN_POINT ( 'NONE',  ( 0.8561741729129456191, 188.3999999989075036, 4.933012699999999029 ) ) ;
#2771=CARTESIAN_POINT ( 'NONE',  ( 2.066987299999999195, 189.1999999989075434, 7.856174172912946396 ) ) ;
#2774=FACE_OUTER_BOUND ( 'NONE', #12641, .T. ) ;
#2775=CARTESIAN_POINT ( 'NONE',  ( 0.000000000000000000, 187.2933328889893687, 9.583808270834989429 ) ) ;
#2778=CARTESIAN_POINT ( 'NONE',  ( 2.746701853510111757, 189.9419816681355542, 6.030501831987404415 ) ) ;
#2780=CARTESIAN_POINT ( 'NONE',  ( 2.997605338728016378, 189.8677746345552748, 7.530719179693556420 ) ) ;
#2785=CARTESIAN_POINT ( 'NONE',  ( 2.066987300000000083, 186.0999999989075206, 6.143825827087054492 ) ) ;
#2796=CARTESIAN_POINT ( 'NONE',  ( -1.514810195292803918, 190.0478454264466848, 4.614282054999431004 ) ) ;
#2805=CARTESIAN_POINT ( 'NONE',  ( -0.09789622041826565035, 228.2551366570249343, 10.16828389758070550 ) ) ;
#2818=CARTESIAN_POINT ( 'NONE',  ( -1.035533905932737753, 185.7499999978150527, 4.500000000000000888 ) ) ;
#2824=CARTESIAN_POINT ( 'NONE',  ( 2.500000000000000444, 187.1699999975965625, 7.000000000000000000 ) ) ;
#2825=CARTESIAN_POINT ( 'NONE',  ( -0.3256308520141213414, 228.9034500205340237, 8.848606045481535176 ) ) ;
#2826=CARTESIAN_POINT ( 'NONE',  ( -2.990426535912302786, 227.3682058476787233, 7.559219386994686651 ) ) ;
#2828=CARTESIAN_POINT ( 'NONE',  ( -0.9975586949907861989, 189.0634563462267010, 10.01833148473745894 ) ) ;
#2836=EDGE_CURVE ( 'NONE', #15371, #8616, #14150, .T. ) ;
#2840=CARTESIAN_POINT ( 'NONE',  ( 1.767766952966368432, 188.7000000000000171, 8.767766952966368876 ) ) ;
#2843=CARTESIAN_POINT ( 'NONE',  ( -5.421010862427522170E-17, 187.4000000000000057, 4.500000000000000000 ) ) ;
#2845=CARTESIAN_POINT ( 'NONE',  ( 1.314367061980813878, 227.7707019980692564, 5.577165148888615143 ) ) ;
#2849=CARTESIAN_POINT ( 'NONE',  ( -1.461580736456473906, 187.9499999989075150, 8.461580736456474128 ) ) ;
#2851=CARTESIAN_POINT ( 'NONE',  ( 0.8561741729129455081, 186.9999999989075263, 4.933012699999999029 ) ) ;
#2856=CARTESIAN_POINT ( 'NONE',  ( 2.265240160886509813, 189.1526725940605331, 9.149827916924719418 ) ) ;
#2859=CARTESIAN_POINT ( 'NONE',  ( 2.985698417011507733, 189.8946583874339638, 6.934546546956198654 ) ) ;
#2864=CARTESIAN_POINT ( 'NONE',  ( -2.066987300000000083, 185.6499999989075320, 7.000000000000000000 ) ) ;
#2874=CARTESIAN_POINT ( 'NONE',  ( -2.900132499248337936, 189.9172581111519094, 6.475756817537924093 ) ) ;
#2875=CARTESIAN_POINT ( 'NONE',  ( 0.8561741729129457301, 189.0999999989075206, 9.066987299999999195 ) ) ;
#2883=ORIENTED_EDGE ( 'NONE', *, *, #3113, .T. ) ;
#2895=FACE_OUTER_BOUND ( 'NONE', #7060, .T. ) ;
#2900=CARTESIAN_POINT ( 'NONE',  ( 1.035533905932738197, 187.8199999975965682, 9.500000000000003553 ) ) ;
#2901=CARTESIAN_POINT ( 'NONE',  ( 1.625192428541204714, 228.1012562471100011, 9.715842694323066908 ) ) ;
#2902=CARTESIAN_POINT ( 'NONE',  ( -0.9651034952757481244, 226.3762748196293728, 4.637298184581183591 ) ) ;
#2918=CARTESIAN_POINT ( 'NONE',  ( 1.035533905932737975, 185.7500000000000568, 4.500000000000000888 ) ) ;
#2920=CARTESIAN_POINT ( 'NONE',  ( -1.864073305829632599, 228.0308260764439297, 6.328418323741104246 ) ) ;
#2921=DIRECTION ( 'NONE',  ( -1.000000000000000000, 0.000000000000000000, 0.000000000000000000 ) ) ;
#2925=EDGE_CURVE ( 'NONE', #3329, #5268, #5890, .T. ) ;
#2926=CARTESIAN_POINT ( 'NONE',  ( 1.461580736456473240, 188.3499999989074922, 5.538419263543526760 ) ) ;
#2928=CARTESIAN_POINT ( 'NONE',  ( -1.461580736456473462, 187.3499999989075206, 8.461580736456472351 ) ) ;
#2929=VERTEX_POINT ( 'NONE', #1026 ) ;
#2931=( GEOMETRIC_REPRESENTATION_CONTEXT ( 3 ) GLOBAL_UNCERTAINTY_ASSIGNED_CONTEXT ( ( #13315 ) ) GLOBAL_UNIT_ASSIGNED_CONTEXT ( ( #7998, #8752, #2695 ) ) REPRESENTATION_CONTEXT ( 'NONE', 'WORKASPACE' ) );
#2933=CARTESIAN_POINT ( 'NONE',  ( -0.001074311305641557088, 226.3251817249170017, 4.486671161788877704 ) ) ;
#2936=CARTESIAN_POINT ( 'NONE',  ( 2.927574602831448658, 189.9114408209157148, 6.589606913355709139 ) ) ;
#2939=CARTESIAN_POINT ( 'NONE',  ( 2.917903144078069833, 189.9135866353617814, 6.547191606018472498 ) ) ;
#2944=CARTESIAN_POINT ( 'NONE',  ( -4.946672411965113980E-16, 185.8499999989075206, 9.066987300000000971 ) ) ;
#2951=( BOUNDED_CURVE ( )  B_SPLINE_CURVE ( 2, ( #813, #4638, #12904, #9411, #9332, #14174, #5756, #11636, #8063 ),
 .UNSPECIFIED., .F., .F. ) 
 B_SPLINE_CURVE_WITH_KNOTS ( ( 3, 2, 2, 2, 3 ),
 ( 0.1428571428571428492, 0.1607142857142857262, 0.1785714285714285754, 0.1964285714285714246, 0.2142857142857142738 ),
 .UNSPECIFIED. ) 
 CURVE ( )  GEOMETRIC_REPRESENTATION_ITEM ( )  RATIONAL_B_SPLINE_CURVE ( ( 1.000000000000000000, 0.9238795325112867385, 1.000000000000000000, 0.9238795325112867385, 1.000000000000000000, 0.9238795325112867385, 1.000000000000000000, 0.9238795325112867385, 1.000000000000000000 ) ) 
 REPRESENTATION_ITEM ( '' )  );
#2972=CARTESIAN_POINT ( 'NONE',  ( -1.035533905932739529, 185.2499999978150811, 9.500000000000003553 ) ) ;
#2976=CARTESIAN_POINT ( 'NONE',  ( -1.767766952966369098, 185.0699999975965397, 5.232233047033630235 ) ) ;
#2977=CARTESIAN_POINT ( 'NONE',  ( -1.619108980504621043, 228.6400225536183655, 8.087812496111112637 ) ) ;
#2978=CARTESIAN_POINT ( 'NONE',  ( -2.439580969806472321, 226.7272467340407331, 5.671663139905907869 ) ) ;
#2979=( BOUNDED_CURVE ( )  B_SPLINE_CURVE ( 2, ( #8358, #9308, #14146, #6929, #4376, #11762, #10652, #1023, #864 ),
 .UNSPECIFIED., .F., .F. ) 
 B_SPLINE_CURVE_WITH_KNOTS ( ( 3, 2, 2, 2, 3 ),
 ( 0.3571428571428571508, 0.3750000000000000000, 0.3928571428571428492, 0.4107142857142856984, 0.4285714285714285476 ),
 .UNSPECIFIED. ) 
 CURVE ( )  GEOMETRIC_REPRESENTATION_ITEM ( )  RATIONAL_B_SPLINE_CURVE ( ( 1.000000000000000000, 0.9238795325112867385, 1.000000000000000000, 0.9238795325112867385, 1.000000000000000000, 0.9238795325112867385, 1.000000000000000000, 0.9238795325112867385, 1.000000000000000000 ) ) 
 REPRESENTATION_ITEM ( '' )  );
#2993=DIRECTION ( 'NONE',  ( -6.123233995736766036E-17, 1.000000000000000000, 0.000000000000000000 ) ) ;
#2996=CARTESIAN_POINT ( 'NONE',  ( 2.500000000000000444, 187.1499999999999773, 8.035533905932739529 ) ) ;
#2997=CARTESIAN_POINT ( 'NONE',  ( -0.1316767729515891938, 227.6100531710845587, 5.113202173749356483 ) ) ;
#3002=CARTESIAN_POINT ( 'NONE',  ( 1.035533905932738419, 185.4499999999999886, 9.500000000000003553 ) ) ;
#3003=CARTESIAN_POINT ( 'NONE',  ( -1.035533905932737975, 187.3499999978151038, 4.500000000000001776 ) ) ;
#3005=CARTESIAN_POINT ( 'NONE',  ( -2.066987300000000083, 187.2499999989075263, 7.000000000000000000 ) ) ;
#3009=CARTESIAN_POINT ( 'NONE',  ( 3.659182332138073087E-16, 190.0875178197511275, 4.201689379953569947 ) ) ;
#3011=CARTESIAN_POINT ( 'NONE',  ( 2.763434297034058407, 189.2181571714553741, 8.347543543386905185 ) ) ;
#3014=CARTESIAN_POINT ( 'NONE',  ( 0.2786071629746884604, 190.0868662572826793, 4.208169715142605405 ) ) ;
#3020=CARTESIAN_POINT ( 'NONE',  ( -2.066987300000000527, 186.2499999989074979, 7.000000000000000000 ) ) ;
#3049=CARTESIAN_POINT ( 'NONE',  ( 1.035533905932738197, 187.7499999978150527, 9.500000000000000000 ) ) ;
#3050=CARTESIAN_POINT ( 'NONE',  ( 1.767766952966369098, 187.9999999978150527, 5.232233047033630235 ) ) ;
#3051=CARTESIAN_POINT ( 'NONE',  ( 2.500000000000000444, 184.6999999978150697, 7.000000000000000000 ) ) ;
#3054=CARTESIAN_POINT ( 'NONE',  ( 2.500000000000000444, 188.8199999975965682, 5.964466094067262247 ) ) ;
#3055=CARTESIAN_POINT ( 'NONE',  ( -1.691178964804313178, 228.6047289695326583, 7.985882612257780622 ) ) ;
#3063=CARTESIAN_POINT ( 'NONE',  ( 2.066987300000000527, 184.2499999989074979, 7.000000000000000000 ) ) ;
#3069=CARTESIAN_POINT ( 'NONE',  ( 0.000000000000000000, 184.0000000000000000, 7.000000000000000000 ) ) ;
#3071=CARTESIAN_POINT ( 'NONE',  ( 1.767766952966368432, 187.8999999999999773, 8.767766952966368876 ) ) ;
#3073=CARTESIAN_POINT ( 'NONE',  ( 1.052850409966403333, 227.7074407335792614, 5.394463008855642450 ) ) ;
#3079=CARTESIAN_POINT ( 'NONE',  ( 2.500000000000000000, 188.7500000000000000, 8.035533905932739529 ) ) ;
#3086=PLANE ( 'NONE',  #12655 ) ;
#3087=ADVANCED_FACE ( 'NONE', ( #13355 ), #5220, .T. ) ;
#3088=CARTESIAN_POINT ( 'NONE',  ( 2.757857370799680297, 189.3567818799732549, 5.841158458801078979 ) ) ;
#3089=CARTESIAN_POINT ( 'NONE',  ( -9.825582188149883933E-17, 188.0999999978150754, 4.500000000000000000 ) ) ;
#3090=CARTESIAN_POINT ( 'NONE',  ( -0.2612047379802446279, 227.6089814726536531, 5.110107047554619975 ) ) ;
#3091=CARTESIAN_POINT ( 'NONE',  ( 1.965304387191771029, 228.1545866171788930, 6.685845824222668377 ) ) ;
#3097=CARTESIAN_POINT ( 'NONE',  ( -0.8561741729129469514, 184.7999999989075093, 9.066987300000000971 ) ) ;
#3110=CARTESIAN_POINT ( 'NONE',  ( 0.000000000000000000, 222.7460571280668091, 12.08513476933103625 ) ) ;
#3113=EDGE_CURVE ( 'NONE', #5590, #13467, #11017, .T. ) ;
#3114=CARTESIAN_POINT ( 'NONE',  ( -2.710505431213761085E-17, 228.2551366889530016, 10.16828399152529983 ) ) ;
#3126=CARTESIAN_POINT ( 'NONE',  ( -7.826584432629735133E-16, 189.2999999978150356, 9.500000000000001776 ) ) ;
#3132=CARTESIAN_POINT ( 'NONE',  ( -1.767766952966369765, 188.4699999975965738, 8.767766952966368876 ) ) ;
#3133=CARTESIAN_POINT ( 'NONE',  ( 2.189302528786933877, 227.9503441805575505, 9.272039875547573473 ) ) ;
#3134=CARTESIAN_POINT ( 'NONE',  ( -1.586193948774629714, 228.1096603596491832, 9.740555404025270647 ) ) ;
#3135=EDGE_CURVE ( 'NONE', #8762, #10770, #8481, .T. ) ;
#3141=CARTESIAN_POINT ( 'NONE',  ( -2.500000000000001776, 189.1499999978151152, 8.035533905932737753 ) ) ;
#3151=CARTESIAN_POINT ( 'NONE',  ( 1.767766952966368432, 188.7000000000000171, 8.767766952966368876 ) ) ;
#3152=CARTESIAN_POINT ( 'NONE',  ( 1.826454486347603767, 228.0556294925947896, 9.581672574142119814 ) ) ;
#3156=CARTESIAN_POINT ( 'NONE',  ( -1.767766952966369765, 186.9000000000000057, 8.767766952966368876 ) ) ;
#3159=ORIENTED_EDGE ( 'NONE', *, *, #10911, .T. ) ;
#3162=CARTESIAN_POINT ( 'NONE',  ( -0.1882270327582609148, 228.2551366869376182, 10.16828399218531587 ) ) ;
#3164=CARTESIAN_POINT ( 'NONE',  ( -2.500000000000000444, 184.3300000002185186, 7.000000000000000000 ) ) ;
#3165=CARTESIAN_POINT ( 'NONE',  ( -1.214607412227127980, 227.7425047733634642, 5.495729955674467426 ) ) ;
#3166=CARTESIAN_POINT ( 'NONE',  ( 0.3231974900581740529, 228.9035839249116009, 8.848992768962338218 ) ) ;
#3172=CARTESIAN_POINT ( 'NONE',  ( -2.066987300000001415, 185.4999999989075548, 7.856174172912944620 ) ) ;
#3174=ADVANCED_FACE ( 'NONE', ( #4359 ), #3086, .F. ) ;
#3179=CARTESIAN_POINT ( 'NONE',  ( -2.066987300000000971, 184.8999999989075320, 7.856174172912944620 ) ) ;
#3180=EDGE_CURVE ( 'NONE', #10913, #9483, #1348, .T. ) ;
#3181=DIRECTION ( 'NONE',  ( -6.123233995736766036E-17, 1.000000000000000000, 0.000000000000000000 ) ) ;
#3186=CARTESIAN_POINT ( 'NONE',  ( 5.999999999999999112, 189.3270225533669020, 3.938484906660877805 ) ) ;
#3190=CARTESIAN_POINT ( 'NONE',  ( -0.05145228733558462192, 189.6978048838913651, 10.38925534086671654 ) ) ;
#3202=CARTESIAN_POINT ( 'NONE',  ( -2.066987300000000083, 185.6499999989075320, 7.000000000000000000 ) ) ;
#3206=CARTESIAN_POINT ( 'NONE',  ( 1.767766952966369098, 189.6699999975965341, 5.232233047033630235 ) ) ;
#3207=CARTESIAN_POINT ( 'NONE',  ( 2.600554376340839635, 226.8075635770346139, 5.908288162427849599 ) ) ;
#3218=CARTESIAN_POINT ( 'NONE',  ( 2.283493650000000041, 184.5749999983613066, 7.000000000000000000 ) ) ;
#3223=CARTESIAN_POINT ( 'NONE',  ( 2.500000000000000444, 185.4999999978150527, 7.000000000000000000 ) ) ;
#3224=B_SPLINE_CURVE_WITH_KNOTS ( 'NONE', 3,
 ( #8127, #4706, #3190, #3501, #15605, #4623 ),
 .UNSPECIFIED., .F., .F.,
 ( 4, 2, 4 ),
 ( 0.01906023950618289733, 0.01909837383777384864, 0.01913650816936479995 ),
 .UNSPECIFIED. ) ;
#3225=CARTESIAN_POINT ( 'NONE',  ( -1.498122667687309173, 228.6899413643594983, 8.231980868713440813 ) ) ;
#3229=CARTESIAN_POINT ( 'NONE',  ( -1.035533905932739751, 187.7500000000000284, 9.500000000000003553 ) ) ;
#3237=CARTESIAN_POINT ( 'NONE',  ( -2.966128040510949582, 227.4385277522438287, 7.766262359440736951 ) ) ;
#3238=CARTESIAN_POINT ( 'NONE',  ( 0.5294602902338498840, 189.4400223437018553, 4.020063421733246933 ) ) ;
#3239=CARTESIAN_POINT ( 'NONE',  ( 1.767766952966369320, 184.0300000002184788, 5.232233047033630235 ) ) ;
#3241=CARTESIAN_POINT ( 'NONE',  ( 1.984332343511774788, 228.2073501340537973, 6.838229870390527765 ) ) ;
#3246=CARTESIAN_POINT ( 'NONE',  ( -2.066987300000000527, 184.6499999989075320, 7.000000000000000000 ) ) ;
#3251=CARTESIAN_POINT ( 'NONE',  ( 2.066987299999999639, 185.1999999989075150, 7.856174172912946396 ) ) ;
#3253=CARTESIAN_POINT ( 'NONE',  ( -0.8561741729129469514, 185.5999999989074922, 9.066987300000000971 ) ) ;
#3258=CARTESIAN_POINT ( 'NONE',  ( -5.999999999999999112, 221.4150671951173592, 6.196499129422101682 ) ) ;
#3277=CARTESIAN_POINT ( 'NONE',  ( 2.500000000000000000, 189.4499999978150697, 8.035533905932739529 ) ) ;
#3285=CARTESIAN_POINT ( 'NONE',  ( 2.843216347914732101, 226.9801049014886587, 6.416521247196312672 ) ) ;
#3302=CARTESIAN_POINT ( 'NONE',  ( -5.861467994999758346E-16, 186.0999999978150754, 9.500000000000001776 ) ) ;
#3304=CARTESIAN_POINT ( 'NONE',  ( -2.913793338554793166E-15, 228.9118723800512782, 8.872930300147347182 ) ) ;
#3311=CARTESIAN_POINT ( 'NONE',  ( -2.500000000000000444, 186.8499999999999943, 8.035533905932737753 ) ) ;
#3322=CARTESIAN_POINT ( 'NONE',  ( 1.895314869936763680, 228.4599366835234093, 7.567714231851713436 ) ) ;
#3327=CARTESIAN_POINT ( 'NONE',  ( 2.066987300000000527, 185.0499999989075093, 7.000000000000000000 ) ) ;
#3329=VERTEX_POINT ( 'NONE', #7129 ) ;
#3331=CARTESIAN_POINT ( 'NONE',  ( -4.438452643612533777E-16, 185.0499999989075093, 9.066987300000000971 ) ) ;
#3333=CARTESIAN_POINT ( 'NONE',  ( 1.461580736456472573, 187.3499999989074922, 8.461580736456474128 ) ) ;
#3337=CARTESIAN_POINT ( 'NONE',  ( -5.999999999999999112, 186.5669965222008670, 9.317226423031115701 ) ) ;
#3353=CARTESIAN_POINT ( 'NONE',  ( 1.035533905932737753, 188.0499999978150640, 4.500000000000000888 ) ) ;
#3358=CARTESIAN_POINT ( 'NONE',  ( -1.035533905932737975, 188.2199999975965738, 4.500000000000000888 ) ) ;
#3359=CARTESIAN_POINT ( 'NONE',  ( 2.923766376317260551, 227.0711491207812855, 6.684645050985161596 ) ) ;
#3363=VERTEX_POINT ( 'NONE', #8492 ) ;
#3378=CARTESIAN_POINT ( 'NONE',  ( 2.500000000000000000, 188.7999999999999829, 7.000000000000000000 ) ) ;
#3379=CARTESIAN_POINT ( 'NONE',  ( -1.724643626337419855, 228.5864753960848077, 7.933165251024266063 ) ) ;
#3383=CARTESIAN_POINT ( 'NONE',  ( 2.500000000000000000, 187.9500000000000455, 8.035533905932739529 ) ) ;
#3390=DIRECTION ( 'NONE',  ( 0.000000000000000000, 0.000000000000000000, 1.000000000000000000 ) ) ;
#3391=CARTESIAN_POINT ( 'NONE',  ( -2.829488734775190473, 226.9686955073827619, 6.382877614595673599 ) ) ;
#3393=CARTESIAN_POINT ( 'NONE',  ( -1.035533905932739751, 186.0800000002184902, 9.500000000000003553 ) ) ;
#3395=CARTESIAN_POINT ( 'NONE',  ( -0.2610185499608090876, 227.6142484773064325, 5.125318457402467942 ) ) ;
#3401=CARTESIAN_POINT ( 'NONE',  ( 2.066987299999999639, 188.9999999989074979, 7.856174172912946396 ) ) ;
#3404=ORIENTED_EDGE ( 'NONE', *, *, #8079, .T. ) ;
#3409=CARTESIAN_POINT ( 'NONE',  ( -1.461580736456473240, 186.1499999989075320, 5.538419263543526760 ) ) ;
#3413=CARTESIAN_POINT ( 'NONE',  ( 3.659182332138577465E-16, 221.4150671951173308, 6.196499129422101682 ) ) ;
#3414=CARTESIAN_POINT ( 'NONE',  ( -1.456896669277396583E-16, 188.8999999978150584, 4.500000000000000000 ) ) ;
#3415=CARTESIAN_POINT ( 'NONE',  ( -2.500000000000001332, 185.1499999978150584, 8.035533905932735976 ) ) ;
#3428=CARTESIAN_POINT ( 'NONE',  ( -1.084202172485504434E-16, 187.8499999989074922, 4.933012699999999029 ) ) ;
#3435=CARTESIAN_POINT ( 'NONE',  ( 2.994032664863047533, 227.2266946368854690, 7.142638454998203379 ) ) ;
#3456=B_SPLINE_SURFACE_WITH_KNOTS ( 'NONE', 1, 3, ( 
 ( #10179, #1888, #14137, #14058, #3166, #10492, #6683, #12784, #14214, #15423, #9225, #8024, #15505, #13985, #4603, #931, #4521, #9454, #4443, #4285, #14289, #5723, #5641, #9376, #9150, #7871, #618, #5797, #6842, #6763, #12712, #5490, #1811, #694, #12862, #10643, #3322, #1966, #6919, #11517, #10565, #9297, #10334, #11824, #11595, #5568, #10414, #15264, #3241, #15188, #3091, #7944, #8107, #8186, #4365, #11680, #13023, #779, #11753, #12946, #15346, #2046, #2122, #856, #6995, #11989, #8347, #4762, #15660, #10724, #5878, #1544, #9618, #7152, #5058, #9990, #8802, #13101, #12444, #3925, #11174, #274, #13265, #1094, #13185, #3395, #9535, #14458, #12071, #5957, #3560, #3849, #8428, #14765, #15582, #11906, #6419, #13555, #6259, #8264, #8722, #10801, #5137, #2283, #9911, #2364, #7232, #11097, #2202, #1384, #14839, #13631, #195, #2664, #11252, #14372, #353, #5218, #2745, #10068, #7517, #4684, #7071, #1460, #12363, #7596, #3476, #1015, #6338, #7986, #13865, #13792, #5607, #12521, #12826, #9115, #1930, #4247, #14917, #13946, #7906, #5376, #3055, #2977, #6649, #7674, #11406, #4007, #6804, #1620, #8886, #9040, #10223, #15152, #15226, #13718, #1852, #12748, #7828, #2825, #6496, #11639, #4329, #6726 ),
 ( #11331, #741, #12678, #5453, #507, #428, #11559, #5299, #10147, #4091, #1695, #12595, #15000, #6571, #656, #9187, #2901, #5528, #8961, #7750, #15074, #4168, #14027, #3133, #1776, #11481, #584, #10300, #10376, #9416, #12982, #13141, #10605, #10531, #4410, #5839, #2242, #15386, #11716, #2160, #7033, #9495, #11864, #892, #7113, #819, #14177, #3435, #4482, #9336, #14251, #3359, #7193, #3285, #2009, #6883, #13062, #3207, #11949, #8066, #8303, #974, #1054, #14328, #10685, #8227, #15545, #9264, #6958, #13228, #12032, #4642, #8391, #5918, #8148, #2085, #5684, #11791, #15307, #1131, #14099, #10765, #5762, #15620, #15464, #3520, #14415, #9573, #4724, #2320, #4566, #10454, #12908, #15702, #13540, #3833, #1441, #14501, #2648, #13613, #6241, #11002, #4885, #8475, #8555, #23, #9744, #14581, #13465, #8630, #258, #7347, #5118, #13379, #12424, #100, #2567, #8705, #12189, #3677, #10922, #5996, #12107, #2489, #14666, #1288, #6162, #11078, #4967, #1368, #13305, #3597, #3908, #177, #7424, #10839, #5041, #9818, #7501, #3755, #12268, #9894, #14747, #12346, #4804, #6319, #11156, #9972, #14823, #8783, #2725, #1208, #7577, #9660, #2404, #7272, #6079, #13695, #14005, #15133, #15055, #9096, #2805, #3114 ) ),
 .UNSPECIFIED., .F., .T., .F.,
 ( 2, 2 ),
 ( 4, 2, 2, 2, 2, 2, 2, 2, 2, 2, 2, 2, 2, 2, 2, 2, 2, 2, 2, 2, 2, 2, 2, 2, 2, 2, 2, 2, 2, 2, 2, 2, 2, 2, 2, 2, 2, 2, 2, 2, 2, 2, 2, 2, 2, 2, 2, 2, 2, 2, 2, 2, 2, 2, 2, 2, 2, 2, 2, 2, 2, 2, 2, 2, 2, 2, 2, 2, 2, 2, 2, 2, 2, 2, 2, 2, 2, 2, 2, 2, 2, 4 ),
 ( 0.000000000000000000, 1.000000000000000000 ),
 ( 0.0002080168337970193793, 0.0004025046291346534252, 0.0005969924244722874711, 0.0006942363221411045754, 0.0007914802198099215712, 0.0009859680151475555630, 0.001180455810485189772, 0.001277699708154006767, 0.001374943605822823763, 0.001472187503491640759, 0.001569431401160457755, 0.001763919196498091747, 0.001958406991835725738, 0.002055650889504542951, 0.002152894787173360164, 0.002347382582510994155, 0.002541870377848628147, 0.002639114275517445360, 0.002736358173186262139, 0.002930845968523896131, 0.003125333763861530122, 0.003222577661530346901, 0.003319821559199164114, 0.003417065456867981327, 0.003514309354536798539, 0.003708797149874432531, 0.003903284945212066523, 0.004097772740549700948, 0.004292260535887335374, 0.004486748331224968932, 0.004681236126562602490, 0.004875723921900236915, 0.005070211717237871341, 0.005264699512575504899, 0.005361943410244322111, 0.005459187307913138457, 0.005653675103250772882, 0.005848162898588407307, 0.005945406796257223653, 0.006042650693926040865, 0.006237138489263674423, 0.006431626284601308849, 0.006626114079938943274, 0.006820601875276577700, 0.007015089670614212125, 0.007112333568283028470, 0.007209577465951845683, 0.007404065261289479241, 0.007598553056627113667, 0.007695796954295930879, 0.007793040851964748092, 0.007890284749633564437, 0.007987528647302382517, 0.008182016442640016943, 0.008376504237977651368, 0.008473748135646467713, 0.008570992033315284059, 0.008765479828652918484, 0.008959967623990552910, 0.009057211521659369255, 0.009154455419328185600, 0.009348943214665820026, 0.009543431010003454451, 0.009640674907672272531, 0.009737918805341088876, 0.009835162703009905222, 0.009932406600678723302, 0.01012689439601635599, 0.01032138219135399042, 0.01041862608902280676, 0.01051586998669162484, 0.01071035778202925753, 0.01090484557736689196, 0.01109933337270452638, 0.01129382116804216081, 0.01148830896337979524, 0.01168279675871742793, 0.01187728455405506235, 0.01207177234939269678, 0.01226626014473032947, 0.01246074794006796389, 0.01265523573540559832 ),
 .UNSPECIFIED. ) ;
#3457=CARTESIAN_POINT ( 'NONE',  ( -6.369687763352338550E-16, 186.8999999978150584, 9.500000000000001776 ) ) ;
#3459=CARTESIAN_POINT ( 'NONE',  ( -0.8817132232236292166, 228.8448810635624682, 8.679455557192847337 ) ) ;
#3462=CARTESIAN_POINT ( 'NONE',  ( -0.7316483636516097899, 190.0789992933224255, 4.287069741549627722 ) ) ;
#3472=CARTESIAN_POINT ( 'NONE',  ( -2.129935357778863558, 226.6102832534906213, 5.327017555938296844 ) ) ;
#3474=CARTESIAN_POINT ( 'NONE',  ( -2.500000000000000888, 187.5800000002184902, 8.035533905932737753 ) ) ;
#3476=CARTESIAN_POINT ( 'NONE',  ( -1.989902382949138460, 228.2815652486739282, 7.052567354366601649 ) ) ;
#3480=FACE_OUTER_BOUND ( 'NONE', #11846, .T. ) ;
#3482=CARTESIAN_POINT ( 'NONE',  ( -4.743384504624081899E-17, 186.8499999989074922, 4.933012699999999029 ) ) ;
#3484=CARTESIAN_POINT ( 'NONE',  ( -1.461580736456473240, 186.1499999989075320, 5.538419263543526760 ) ) ;
#3493=CARTESIAN_POINT ( 'NONE',  ( -1.461580736456473240, 186.9499999989075150, 5.538419263543526760 ) ) ;
#3501=CARTESIAN_POINT ( 'NONE',  ( -0.02572782006998338561, 189.6977761910882805, 10.38959324765381709 ) ) ;
#3514=CARTESIAN_POINT ( 'NONE',  ( 2.066987300000000083, 187.6499999989075320, 7.000000000000000000 ) ) ;
#3520=CARTESIAN_POINT ( 'NONE',  ( -0.3933619333212962643, 226.3329841201265253, 4.509674143907711041 ) ) ;
#3540=CARTESIAN_POINT ( 'NONE',  ( -1.035533905932739751, 186.8499999978150470, 9.500000000000003553 ) ) ;
#3541=CARTESIAN_POINT ( 'NONE',  ( 0.6843230633849453071, 226.3504559366005537, 4.561183366923295068 ) ) ;
#3553=EDGE_CURVE ( 'NONE', #6574, #9005, #6937, .T. ) ;
#3555=CARTESIAN_POINT ( 'NONE',  ( -2.718436142382103071, 227.6979080801118300, 8.529473091820765518 ) ) ;
#3558=CARTESIAN_POINT ( 'NONE',  ( -2.500000000000000444, 187.4800000002184959, 5.964466094067261359 ) ) ;
#3560=CARTESIAN_POINT ( 'NONE',  ( -0.6404026449181154934, 227.6435107573390724, 5.209829591148105621 ) ) ;
#3561=CARTESIAN_POINT ( 'NONE',  ( 0.4515139163396761357, 228.8949857255690290, 8.824160678851793449 ) ) ;
#3563=CYLINDRICAL_SURFACE ( 'NONE', #5189, 2.500000000000000444 ) ;
#3565=CARTESIAN_POINT ( 'NONE',  ( -2.066987300000000527, 187.0499999989075093, 7.000000000000000000 ) ) ;
#3566=CARTESIAN_POINT ( 'NONE',  ( 2.066987300000000971, 186.6999999989075150, 6.143825827087054492 ) ) ;
#3569=( BOUNDED_SURFACE ( )  B_SPLINE_SURFACE ( 3, 2, ( 
 ( #233, #10976, #3883 ),
 ( #8756, #4941, #14642 ),
 ( #14478, #197, #13588 ),
 ( #3730, #8608, #7550 ),
 ( #10818, #15679, #7248 ),
 ( #12086, #1185, #6057 ),
 ( #10902, #1729, #12709 ),
 ( #1652, #7868, #383 ),
 ( #7784, #4282, #6374 ),
 ( #4044, #6526, #14952 ),
 ( #7705, #2856, #13665 ),
 ( #13749, #8915, #5334 ),
 ( #11514, #309, #15185 ),
 ( #13900, #3011, #461 ),
 ( #11286, #11208, #12475 ),
 ( #15030, #12554, #11361 ),
 ( #10177, #6604, #8835 ),
 ( #9147, #539, #8996 ),
 ( #11438, #4124, #1807 ),
 ( #12630, #13823, #2936 ),
 ( #5170, #5253, #6681 ),
 ( #5408, #13982, #2778 ),
 ( #10100, #3088, #12781 ),
 ( #10023, #10255, #9074 ),
 ( #7631, #15107, #4205 ),
 ( #615, #5487, #10331 ),
 ( #3961, #7941, #14871 ),
 ( #1576, #6454, #927 ),
 ( #8104, #6991, #5719 ),
 ( #10411, #14133, #8343 ),
 ( #15260, #11591, #11750 ),
 ( #691, #3238, #4681 ),
 ( #11820, #15579, #13098 ),
 ( #1963, #9222, #12942 ) ),
 .UNSPECIFIED., .F., .F., .F. ) 
 B_SPLINE_SURFACE_WITH_KNOTS ( ( 4, 2, 2, 2, 2, 2, 2, 2, 2, 2, 2, 2, 2, 2, 2, 2, 4 ),
 ( 3, 3 ),
 ( 0.000000000000000000, 0.0004059453939305676402, 0.0008118907878611352803, 0.001217836181791702920, 0.001623781575722270561, 0.002029726969652837984, 0.002435672363583405841, 0.002841617757513973698, 0.003247563151444541121, 0.003653508545375108545, 0.004059453939305675968, 0.004465399333236244259, 0.004871344727166811682, 0.005277290121097379105, 0.005683235515027947396, 0.006089180908958514819, 0.006495126302889082243 ),
 ( 0.000000000000000000, 1.000000000000000000 ),
 .UNSPECIFIED. ) 
 GEOMETRIC_REPRESENTATION_ITEM ( )  RATIONAL_B_SPLINE_SURFACE ( (
 ( 1.000000000000000000, 0.8248771365966364177, 1.000000000000000000),
 ( 1.000000000000000000, 0.8247993752883225893, 1.000000000000000000),
 ( 1.000000000000000000, 0.8250334644212878876, 1.000000000000000000),
 ( 1.000000000000000000, 0.8260937318508657645, 1.000000000000000000),
 ( 1.000000000000000000, 0.8269351727486546899, 1.000000000000000000),
 ( 1.000000000000000000, 0.8291161194214680119, 1.000000000000000000),
 ( 1.000000000000000000, 0.8304526363639401776, 1.000000000000000000),
 ( 1.000000000000000000, 0.8335574816758006822, 1.000000000000000000),
 ( 1.000000000000000000, 0.8353047682308820665, 1.000000000000000000),
 ( 1.000000000000000000, 0.8389997731991114538, 1.000000000000000000),
 ( 1.000000000000000000, 0.8409810165338121868, 1.000000000000000000),
 ( 1.000000000000000000, 0.8449567606309243972, 1.000000000000000000),
 ( 1.000000000000000000, 0.8469382525847787280, 1.000000000000000000),
 ( 1.000000000000000000, 0.8507236134161916263, 1.000000000000000000),
 ( 1.000000000000000000, 0.8525331645253796387, 1.000000000000000000),
 ( 1.000000000000000000, 0.8556292709850843448, 1.000000000000000000),
 ( 1.000000000000000000, 0.8569340980096278315, 1.000000000000000000),
 ( 1.000000000000000000, 0.8588235378423549893, 1.000000000000000000),
 ( 1.000000000000000000, 0.8593913334868529263, 1.000000000000000000),
 ( 1.000000000000000000, 0.8595838334664910318, 1.000000000000000000),
 ( 1.000000000000000000, 0.8592170625035302489, 1.000000000000000000),
 ( 1.000000000000000000, 0.8574834265527571109, 1.000000000000000000),
 ( 1.000000000000000000, 0.8561196021166810333, 1.000000000000000000),
 ( 1.000000000000000000, 0.8526284468138234374, 1.000000000000000000),
 ( 1.000000000000000000, 0.8504944293460048321, 1.000000000000000000),
 ( 1.000000000000000000, 0.8457235101200186733, 1.000000000000000000),
 ( 1.000000000000000000, 0.8431479293774302164, 1.000000000000000000),
 ( 1.000000000000000000, 0.8381225573515114213, 1.000000000000000000),
 ( 1.000000000000000000, 0.8356411947703757948, 1.000000000000000000),
 ( 1.000000000000000000, 0.8312972710846878721, 1.000000000000000000),
 ( 1.000000000000000000, 0.8294811344191250768, 1.000000000000000000),
 ( 1.000000000000000000, 0.8268651351247819914, 1.000000000000000000),
 ( 1.000000000000000000, 0.8260641663560207570, 1.000000000000000000),
 ( 1.000000000000000000, 0.8259116551296904474, 1.000000000000000000) ) ) 
 REPRESENTATION_ITEM ( '' )  SURFACE ( )  );
#3571=LINE ( 'NONE', #10971, #4513 ) ;
#3573=CARTESIAN_POINT ( 'NONE',  ( 1.461580736456473240, 186.7499999989075263, 5.538419263543526760 ) ) ;
#3581=CARTESIAN_POINT ( 'NONE',  ( -1.767766952966369320, 187.5000000000000000, 5.232233047033630235 ) ) ;
#3584=ORIENTED_EDGE ( 'NONE', *, *, #1627, .F. ) ;
#3591=CARTESIAN_POINT ( 'NONE',  ( -2.066987300000000527, 188.8499999989074922, 7.000000000000000000 ) ) ;
#3596=CYLINDRICAL_SURFACE ( 'NONE', #15727, 2.500000000000000444 ) ;
#3597=CARTESIAN_POINT ( 'NONE',  ( -2.960186505457850892, 227.4470585832885661, 7.791309201570119747 ) ) ;
#3618=CARTESIAN_POINT ( 'NONE',  ( 1.767766952966368432, 188.5999999978150470, 8.767766952966368876 ) ) ;
#3619=CARTESIAN_POINT ( 'NONE',  ( 1.751153496549405775, 226.5057898163625794, 5.019064844972819017 ) ) ;
#3623=ORIENTED_EDGE ( 'NONE', *, *, #9073, .F. ) ;
#3627=ORIENTED_EDGE ( 'NONE', *, *, #7831, .T. ) ;
#3635=CARTESIAN_POINT ( 'NONE',  ( 2.500000000000000000, 187.8800000002185016, 8.035533905932739529 ) ) ;
#3637=CARTESIAN_POINT ( 'NONE',  ( 1.724621985266778568, 228.5864789591000488, 7.933175541215780946 ) ) ;
#3641=CARTESIAN_POINT ( 'NONE',  ( -2.066987300000001859, 188.6999999989075150, 7.856174172912944620 ) ) ;
#3642=CARTESIAN_POINT ( 'NONE',  ( -1.461580736456473684, 185.5499999989075093, 8.461580736456474128 ) ) ;
#3650=CARTESIAN_POINT ( 'NONE',  ( -1.649561345686224145, 189.0000000000000000, 8.881879043882671354 ) ) ;
#3653=DIRECTION ( 'NONE',  ( -6.123233995736766036E-17, 1.000000000000000000, 0.000000000000000000 ) ) ;
#3670=CARTESIAN_POINT ( 'NONE',  ( -1.461580736456473462, 187.3499999989075206, 8.461580736456472351 ) ) ;
#3677=CARTESIAN_POINT ( 'NONE',  ( -2.922039326512111401, 227.0704416020563201, 6.682560001249291837 ) ) ;
#3686=CARTESIAN_POINT ( 'NONE',  ( 2.500000000000000444, 185.5999999999999943, 7.000000000000000000 ) ) ;
#3688=DIRECTION ( 'NONE',  ( 1.000000000000000000, 6.123233995736603333E-17, 6.123233995738439900E-17 ) ) ;
#3694=ADVANCED_FACE ( 'NONE', ( #9720 ), #13590, .T. ) ;
#3695=CARTESIAN_POINT ( 'NONE',  ( 2.500000000000000444, 187.0499999978150640, 8.035533905932739529 ) ) ;
#3696=CARTESIAN_POINT ( 'NONE',  ( 2.961265621965179395, 227.4473031124620377, 7.792030372366526514 ) ) ;
#3703=CARTESIAN_POINT ( 'NONE',  ( -1.767766952966369765, 187.7000000000000171, 8.767766952966368876 ) ) ;
#3705=CARTESIAN_POINT ( 'NONE',  ( 0.9161293052571292117, 226.3710829030681566, 4.621973948928255638 ) ) ;
#3712=CARTESIAN_POINT ( 'NONE',  ( -1.035533905932739751, 188.4800000002184959, 9.500000000000003553 ) ) ;
#3714=CARTESIAN_POINT ( 'NONE',  ( 1.886647494277889692, 228.0514830721454871, 6.388076905524764371 ) ) ;
#3719=CARTESIAN_POINT ( 'NONE',  ( -6.776263578034402713E-16, 188.8499999989074922, 9.066987300000000971 ) ) ;
#3720=CARTESIAN_POINT ( 'NONE',  ( 2.066987300000000083, 184.9999999989074979, 7.856174172912946396 ) ) ;
#3722=CARTESIAN_POINT ( 'NONE',  ( -2.066987300000000083, 185.6499999989075320, 7.000000000000000000 ) ) ;
#3723=VERTEX_POINT ( 'NONE', #15729 ) ;
#3728=CARTESIAN_POINT ( 'NONE',  ( 2.066987300000000083, 188.2999999989075093, 6.143825827087054492 ) ) ;
#3730=CARTESIAN_POINT ( 'NONE',  ( 0.5022380393797636344, 188.9999999999267004, 9.452991704445535603 ) ) ;
#3747=CARTESIAN_POINT ( 'NONE',  ( -1.461580736456473240, 185.7499999989074979, 8.461580736456472351 ) ) ;
#3755=CARTESIAN_POINT ( 'NONE',  ( -2.691043998642291157, 227.7164964219492163, 8.584158233643494285 ) ) ;
#3757=EDGE_LOOP ( 'NONE', ( #6304, #1136, #14751, #12410 ) ) ;
#3761=CARTESIAN_POINT ( 'NONE',  ( 2.079732659162522257, 189.0000000000000284, 5.600772967838274496 ) ) ;
#3766=CARTESIAN_POINT ( 'NONE',  ( -1.626303258728256651E-16, 189.0624999997268390, 4.608253174999999757 ) ) ;
#3770=CARTESIAN_POINT ( 'NONE',  ( 2.500000000000000000, 188.0000000000000000, 7.000000000000000000 ) ) ;
#3773=CARTESIAN_POINT ( 'NONE',  ( 1.767766952966368432, 189.3999999978150584, 8.767766952966368876 ) ) ;
#3774=CARTESIAN_POINT ( 'NONE',  ( 1.586671692599169736, 226.4708623422775418, 4.916117818249839289 ) ) ;
#3775=CARTESIAN_POINT ( 'NONE',  ( -1.507559010347591544, 189.0898762284225825, 9.781293306605691740 ) ) ;
#3782=CARTESIAN_POINT ( 'NONE',  ( 1.318933956306606925, 226.4213524663575754, 4.770181869611323400 ) ) ;
#3788=CARTESIAN_POINT ( 'NONE',  ( -1.035533905932737975, 187.3800000002185016, 4.500000000000000888 ) ) ;
#3791=CARTESIAN_POINT ( 'NONE',  ( 0.1297182620452491941, 228.9108343529357228, 8.869932418632497928 ) ) ;
#3797=ADVANCED_FACE ( 'NONE', ( #6292 ), #13444, .T. ) ;
#3798=CARTESIAN_POINT ( 'NONE',  ( -5.793705359219414319E-16, 187.2499999989075263, 9.066987300000000971 ) ) ;
#3800=CARTESIAN_POINT ( 'NONE',  ( -1.461580736456472795, 184.7499999989074979, 5.538419263543527649 ) ) ;
#3807=CARTESIAN_POINT ( 'NONE',  ( 5.999999999999999112, 227.2817795252328210, 4.165129161027028459 ) ) ;
#3808=CARTESIAN_POINT ( 'NONE',  ( 2.066987300000000083, 189.0499999989075093, 7.000000000000000000 ) ) ;
#3818=CARTESIAN_POINT ( 'NONE',  ( 1.461580736456472351, 186.7499999989075263, 8.461580736456474128 ) ) ;
#3833=CARTESIAN_POINT ( 'NONE',  ( -1.501309217710235622, 226.4539600517547910, 4.866297710963618073 ) ) ;
#3835=ORIENTED_EDGE ( 'NONE', *, *, #13288, .T. ) ;
#3843=CARTESIAN_POINT ( 'NONE',  ( -1.767766952966369542, 185.1999999978150697, 8.767766952966368876 ) ) ;
#3848=CARTESIAN_POINT ( 'NONE',  ( 1.767766952966368654, 186.2699999975965568, 8.767766952966368876 ) ) ;
#3849=CARTESIAN_POINT ( 'NONE',  ( -0.7022813136239680620, 227.6507649362739585, 5.230780073663146013 ) ) ;
#3850=CARTESIAN_POINT ( 'NONE',  ( 2.599042177021809508, 227.7726851971488315, 8.749463102108622437 ) ) ;
#3860=CARTESIAN_POINT ( 'NONE',  ( 2.878492383785107744, 227.5628096391837971, 8.132007509143102553 ) ) ;
#3865=CARTESIAN_POINT ( 'NONE',  ( 2.500000000000000444, 185.5999999999999943, 7.000000000000000000 ) ) ;
#3867=CARTESIAN_POINT ( 'NONE',  ( 1.923823996436629047, 228.4292023995385250, 7.478951866735841669 ) ) ;
#3872=CARTESIAN_POINT ( 'NONE',  ( 0.8561741729129458411, 188.8999999989074752, 9.066987300000000971 ) ) ;
#3874=CARTESIAN_POINT ( 'NONE',  ( 0.8561741729129455081, 185.3999999989075889, 4.933012699999999029 ) ) ;
#3877=CYLINDRICAL_SURFACE ( 'NONE', #12628, 2.500000000000000444 ) ;
#3880=CARTESIAN_POINT ( 'NONE',  ( -5.999999999999999112, 215.7452399395091618, 13.29567785264566027 ) ) ;
#3883=CARTESIAN_POINT ( 'NONE',  ( -0.07717340183324516989, 189.6978550888158850, 10.38866401756453328 ) ) ;
#3885=CARTESIAN_POINT ( 'NONE',  ( 2.843793502989464983, 189.8324628781118690, 8.306572263327813843 ) ) ;
#3888=CARTESIAN_POINT ( 'NONE',  ( -0.3303979037561528553, 189.0000000000000284, 4.516547480436640782 ) ) ;
#3890=CARTESIAN_POINT ( 'NONE',  ( 2.066987299999999639, 188.4999999989074979, 6.143825827087054492 ) ) ;
#3893=ORIENTED_EDGE ( 'NONE', *, *, #8071, .F. ) ;
#3895=FACE_OUTER_BOUND ( 'NONE', #6208, .T. ) ;
#3899=CARTESIAN_POINT ( 'NONE',  ( -2.696515973634777907, 189.9486803746651162, 5.919686589971288271 ) ) ;
#3908=CARTESIAN_POINT ( 'NONE',  ( -2.951760543192366804, 227.4626507460308744, 7.837199003427246069 ) ) ;
#3913=CARTESIAN_POINT ( 'NONE',  ( 0.4407554183254575597, 188.9999999999999716, 4.532388849764692473 ) ) ;
#3918=CARTESIAN_POINT ( 'NONE',  ( 2.500000000000000444, 187.8999999978150584, 7.000000000000000000 ) ) ;
#3919=CARTESIAN_POINT ( 'NONE',  ( 0.000000000000000000, 186.4999999978150527, 4.500000000000000000 ) ) ;
#3920=CARTESIAN_POINT ( 'NONE',  ( -2.500000000000000444, 185.2000000000000171, 7.000000000000000000 ) ) ;
#3924=CARTESIAN_POINT ( 'NONE',  ( 2.500000000000000444, 186.3199999975965966, 8.035533905932739529 ) ) ;
#3925=CARTESIAN_POINT ( 'NONE',  ( 0.3253281796544252868, 227.6173729869818771, 5.134342219554626219 ) ) ;
#3926=CARTESIAN_POINT ( 'NONE',  ( -2.191791664054325572, 227.9495085101182781, 9.269582106420829248 ) ) ;
#3928=CARTESIAN_POINT ( 'NONE',  ( -2.815864604846499919, 189.2275809052524664, 8.215757671725111067 ) ) ;
#3935=CARTESIAN_POINT ( 'NONE',  ( 0.7710626327916485501, 228.2248363320221642, 10.07924096547705872 ) ) ;
#3941=CARTESIAN_POINT ( 'NONE',  ( 2.500000000000000444, 184.8499999999999943, 5.964466094067262247 ) ) ;
#3944=CARTESIAN_POINT ( 'NONE',  ( -1.288813234857717038, 227.7638191499166851, 5.557287090853593625 ) ) ;
#3949=CARTESIAN_POINT ( 'NONE',  ( 1.423015351387224570E-16, 184.1999999999999886, 4.500000000000000000 ) ) ;
#3952=CARTESIAN_POINT ( 'NONE',  ( -0.8561741729129469514, 188.9999999989075263, 9.066987299999999195 ) ) ;
#3956=DIRECTION ( 'NONE',  ( -1.000000000000000000, 0.000000000000000000, 0.000000000000000000 ) ) ;
#3957=CARTESIAN_POINT ( 'NONE',  ( 3.659182332138577465E-16, 227.2817795252328210, 4.165129161027028459 ) ) ;
#3959=CARTESIAN_POINT ( 'NONE',  ( -1.968030457003884015, 189.0000000000000000, 8.558443299018994921 ) ) ;
#3961=CARTESIAN_POINT ( 'NONE',  ( 1.727510648855079767, 189.0000000003634000, 5.183832296574240495 ) ) ;
#3963=CARTESIAN_POINT ( 'NONE',  ( 2.046795664782080415, 190.0128272625842953, 5.019430763338620594 ) ) ;
#3968=CARTESIAN_POINT ( 'NONE',  ( 0.8561741729129458411, 188.2999999989075093, 9.066987299999999195 ) ) ;
#3973=CYLINDRICAL_SURFACE ( 'NONE', #15468, 2.500000000000000444 ) ;
#3977=CARTESIAN_POINT ( 'NONE',  ( -0.7858668154420391794, 190.0775333035548158, 4.301934987860914106 ) ) ;
#4001=CARTESIAN_POINT ( 'NONE',  ( 2.500000000000000444, 185.4499999978150981, 8.035533905932739529 ) ) ;
#4006=CARTESIAN_POINT ( 'NONE',  ( -3.388131789017201356E-18, 186.5699999975965397, 4.500000000000000000 ) ) ;
#4007=CARTESIAN_POINT ( 'NONE',  ( -1.361424426418679889, 228.7361946629245892, 8.365563033085530620 ) ) ;
#4008=CARTESIAN_POINT ( 'NONE',  ( -1.942272232823049061, 226.5542875158922129, 5.161998670295230518 ) ) ;
#4011=CARTESIAN_POINT ( 'NONE',  ( -2.665324589450957848, 189.8106497419773291, 8.736655013898124267 ) ) ;
#4017=CARTESIAN_POINT ( 'NONE',  ( 2.273809214555841951, 227.9194763741126906, 9.181262328259517602 ) ) ;
#4024=CARTESIAN_POINT ( 'NONE',  ( 1.767766952966369098, 187.2999999999999829, 5.232233047033630235 ) ) ;
#4026=CARTESIAN_POINT ( 'NONE',  ( -1.238081232355301875, 227.7501834494555055, 5.517906410191214306 ) ) ;
#4027=CYLINDRICAL_SURFACE ( 'NONE', #6528, 2.500000000000000444 ) ;
#4031=CARTESIAN_POINT ( 'NONE',  ( -0.8561741729129472844, 188.7999999989075093, 9.066987300000000971 ) ) ;
#4034=CARTESIAN_POINT ( 'NONE',  ( -2.066987300000000083, 186.3999999989075320, 6.143825827087054492 ) ) ;
#4044=CARTESIAN_POINT ( 'NONE',  ( 1.644293605570781969, 188.9999999996334168, 8.888752494527455639 ) ) ;
#4051=CARTESIAN_POINT ( 'NONE',  ( 2.066987300000000083, 186.8999999989075036, 6.143825827087054492 ) ) ;
#4062=CARTESIAN_POINT ( 'NONE',  ( -1.032108583833363236, 228.1961951329309954, 9.994999926284295455 ) ) ;
#4063=CARTESIAN_POINT ( 'NONE',  ( 1.461580736456472795, 189.3499999989074922, 5.538419263543527649 ) ) ;
#4068=CARTESIAN_POINT ( 'NONE',  ( 2.500000000000000444, 187.2000000000000171, 7.000000000000000000 ) ) ;
#4077=CARTESIAN_POINT ( 'NONE',  ( 1.955037903476808836, 189.0000000000000000, 8.565347030709547838 ) ) ;
#4080=EDGE_CURVE ( 'NONE', #3329, #14887, #1826, .T. ) ;
#4084=CARTESIAN_POINT ( 'NONE',  ( 1.767766952966368654, 186.1999999978150697, 8.767766952966368876 ) ) ;
#4090=CARTESIAN_POINT ( 'NONE',  ( -1.035533905932739529, 186.1199999975965511, 9.500000000000003553 ) ) ;
#4091=CARTESIAN_POINT ( 'NONE',  ( 0.9648499430152943646, 228.2043505555869274, 10.01897217821435859 ) ) ;
#4092=CARTESIAN_POINT ( 'NONE',  ( -2.257095642740105212, 226.6533546677793538, 5.453940291146690988 ) ) ;
#4093=( BOUNDED_CURVE ( )  B_SPLINE_CURVE ( 2, ( #627, #11300, #5500, #13680, #10343, #12646, #12796, #15121, #11451 ),
 .UNSPECIFIED., .F., .F. ) 
 B_SPLINE_CURVE_WITH_KNOTS ( ( 3, 2, 2, 2, 3 ),
 ( 0.2857142857142856984, 0.3035714285714285476, 0.3214285714285714524, 0.3392857142857143016, 0.3571428571428571508 ),
 .UNSPECIFIED. ) 
 CURVE ( )  GEOMETRIC_REPRESENTATION_ITEM ( )  RATIONAL_B_SPLINE_CURVE ( ( 1.000000000000000000, 0.9238795325112867385, 1.000000000000000000, 0.9238795325112867385, 1.000000000000000000, 0.9238795325112867385, 1.000000000000000000, 0.9238795325112867385, 1.000000000000000000 ) ) 
 REPRESENTATION_ITEM ( '' )  );
#4096=EDGE_LOOP ( 'NONE', ( #2726, #14804, #12967, #2473 ) ) ;
#4100=CARTESIAN_POINT ( 'NONE',  ( -2.066760391300492827E-16, 189.4499999989075150, 4.933012699999999029 ) ) ;
#4102=CARTESIAN_POINT ( 'NONE',  ( 2.135537325812093989, 227.9676068176768524, 9.322809720636362485 ) ) ;
#4109=CARTESIAN_POINT ( 'NONE',  ( -1.767766952966369320, 185.9000000000000057, 5.232233047033630235 ) ) ;
#4110=CARTESIAN_POINT ( 'NONE',  ( 0.9965032137571403492, 227.6963699622695287, 5.362489989878645780 ) ) ;
#4111=DIRECTION ( 'NONE',  ( -6.123233995736766036E-17, 1.000000000000000000, 0.000000000000000000 ) ) ;
#4114=VECTOR ( 'NONE', #11652, 1000.000000000000114 ) ;
#4115=CARTESIAN_POINT ( 'NONE',  ( 2.066987300000000083, 188.2499999989075263, 7.000000000000000000 ) ) ;
#4117=CARTESIAN_POINT ( 'NONE',  ( -1.461580736456473018, 188.7499999989075263, 5.538419263543527649 ) ) ;
#4118=ORIENTED_EDGE ( 'NONE', *, *, #9073, .T. ) ;
#4120=CARTESIAN_POINT ( 'NONE',  ( 1.035533905932738197, 186.9499999978150413, 9.500000000000000000 ) ) ;
#4124=CARTESIAN_POINT ( 'NONE',  ( 3.013685100799304184, 189.2999267616114878, 7.018152099054431048 ) ) ;
#4131=CARTESIAN_POINT ( 'NONE',  ( -2.066987300000001415, 188.0999999989074922, 7.856174172912944620 ) ) ;
#4135=AXIS2_PLACEMENT_3D ( 'NONE', #14602, #13398, #12282 ) ;
#4152=ADVANCED_FACE ( 'NONE', ( #10563 ), #14974, .T. ) ;
#4163=CARTESIAN_POINT ( 'NONE',  ( -1.767766952966369765, 187.5999999978150754, 8.767766952966368876 ) ) ;
#4164=CARTESIAN_POINT ( 'NONE',  ( -6.369687763352338550E-16, 186.8999999978150584, 9.500000000000001776 ) ) ;
#4167=CARTESIAN_POINT ( 'NONE',  ( -2.500000000000000444, 186.7199999975965454, 5.964466094067261359 ) ) ;
#4168=CARTESIAN_POINT ( 'NONE',  ( 1.978507955918972439, 228.0159604248740663, 9.465015589616863068 ) ) ;
#4169=CARTESIAN_POINT ( 'NONE',  ( -2.548643141829932901, 227.7997363639018147, 8.829041127271985090 ) ) ;
#4173=ORIENTED_EDGE ( 'NONE', *, *, #11196, .T. ) ;
#4176=CARTESIAN_POINT ( 'NONE',  ( 1.767766952966369098, 189.5999999978150470, 5.232233047033630235 ) ) ;
#4179=CARTESIAN_POINT ( 'NONE',  ( 1.485919012929320271, 228.1288645930629286, 9.797042361818872891 ) ) ;
#4186=CARTESIAN_POINT ( 'NONE',  ( 2.500000000000000444, 187.2000000000000171, 7.000000000000000000 ) ) ;
#4188=CARTESIAN_POINT ( 'NONE',  ( -1.724657202313207849, 227.9349080091615178, 6.051401474621576071 ) ) ;
#4189=PRODUCT_DEFINITION_CONTEXT ( 'detailed design', #4761, 'design' ) ;
#4194=CARTESIAN_POINT ( 'NONE',  ( -1.767766952966369542, 185.2999999999999829, 8.767766952966368876 ) ) ;
#4197=CARTESIAN_POINT ( 'NONE',  ( -5.895349312889930360E-16, 187.4499999989075150, 9.066987300000000971 ) ) ;
#4203=CARTESIAN_POINT ( 'NONE',  ( 0.01327486276323468564, 190.0875178197512696, 4.201689379953597481 ) ) ;
#4205=CARTESIAN_POINT ( 'NONE',  ( 2.348212394088349253, 189.9869324597729587, 5.353485886314879316 ) ) ;
#4208=CARTESIAN_POINT ( 'NONE',  ( 0.07962197837297851910, 190.0874091994478761, 4.202769589527710181 ) ) ;
#4213=CARTESIAN_POINT ( 'NONE',  ( 0.8561741729129461742, 184.8999999989075320, 9.066987300000000971 ) ) ;
#4241=CARTESIAN_POINT ( 'NONE',  ( -2.500000000000000888, 189.0999999978150470, 7.000000000000000000 ) ) ;
#4245=ADVANCED_FACE ( 'NONE', ( #9743 ), #3596, .T. ) ;
#4247=CARTESIAN_POINT ( 'NONE',  ( -1.826974499845722466, 228.5193582813216153, 7.739327195479140720 ) ) ;
#4248=CARTESIAN_POINT ( 'NONE',  ( -2.998822209637060254, 227.3208645008386668, 7.419865387590665939 ) ) ;
#4256=CARTESIAN_POINT ( 'NONE',  ( 1.767766952966368432, 189.3999999978150584, 8.767766952966368876 ) ) ;
#4257=CARTESIAN_POINT ( 'NONE',  ( 2.066987300000000971, 184.2999999989074809, 6.143825827087054492 ) ) ;
#4263=FACE_OUTER_BOUND ( 'NONE', #5596, .T. ) ;
#4267=CARTESIAN_POINT ( 'NONE',  ( 1.035533905932737753, 188.1499999999999773, 4.500000000000000888 ) ) ;
#4268=CARTESIAN_POINT ( 'NONE',  ( 1.454231928715901123, 227.8150477629479269, 5.705238247175231869 ) ) ;
#4272=CARTESIAN_POINT ( 'NONE',  ( 1.767766952966368432, 186.2999999999999829, 8.767766952966368876 ) ) ;
#4282=CARTESIAN_POINT ( 'NONE',  ( 1.857821011765909747, 189.1149986214457783, 9.541363111238132078 ) ) ;
#4283=CARTESIAN_POINT ( 'NONE',  ( 1.035533905932737753, 188.0499999978150356, 4.500000000000001776 ) ) ;
#4284=CARTESIAN_POINT ( 'NONE',  ( -0.0007128680628333008105, 227.6089742637946642, 5.110086227958842819 ) ) ;
#4285=CARTESIAN_POINT ( 'NONE',  ( 1.211961328308884367, 228.7773363860045492, 8.484382675910040916 ) ) ;
#4291=CARTESIAN_POINT ( 'NONE',  ( -2.066987300000001415, 186.2999999989075093, 7.856174172912944620 ) ) ;
#4292=CARTESIAN_POINT ( 'NONE',  ( 1.767766952966368654, 184.7000000000000171, 8.767766952966368876 ) ) ;
#4293=ORIENTED_EDGE ( 'NONE', *, *, #8957, .T. ) ;
#4300=CARTESIAN_POINT ( 'NONE',  ( 2.066987300000000527, 184.2999999989075093, 6.143825827087054492 ) ) ;
#4305=CARTESIAN_POINT ( 'NONE',  ( -5.999999999999999112, 185.8606548077538321, 9.048340948986950849 ) ) ;
#4310=( GEOMETRIC_REPRESENTATION_CONTEXT ( 3 ) GLOBAL_UNCERTAINTY_ASSIGNED_CONTEXT ( ( #2502 ) ) GLOBAL_UNIT_ASSIGNED_CONTEXT ( ( #2041, #14210, #4679 ) ) REPRESENTATION_CONTEXT ( 'NONE', 'WORKASPACE' ) );
#4321=CARTESIAN_POINT ( 'NONE',  ( 2.500000000000000444, 189.5499999978150640, 5.964466094067262247 ) ) ;
#4328=CARTESIAN_POINT ( 'NONE',  ( 2.500000000000000444, 189.6199999975965795, 5.964466094067262247 ) ) ;
#4329=CARTESIAN_POINT ( 'NONE',  ( -0.06495987523897406302, 228.9118723585069120, 8.872930237925691799 ) ) ;
#4331=CARTESIAN_POINT ( 'NONE',  ( -2.710505431213761085E-17, 228.2551366889530016, 10.16828399152529983 ) ) ;
#4341=SURFACE_STYLE_FILL_AREA ( #9198 ) ;
#4345=CARTESIAN_POINT ( 'NONE',  ( 1.035533905932737975, 186.4499999978150697, 4.500000000000000888 ) ) ;
#4347=CARTESIAN_POINT ( 'NONE',  ( -1.923824245924939058, 228.4291822535419954, 7.478893683947804405 ) ) ;
#4353=CARTESIAN_POINT ( 'NONE',  ( -2.500000000000000444, 186.0500000000000114, 8.035533905932737753 ) ) ;
#4359=FACE_OUTER_BOUND ( 'NONE', #2389, .T. ) ;
#4360=CARTESIAN_POINT ( 'NONE',  ( -0.3990466364818540668, 190.0854366310740318, 4.222250755151196522 ) ) ;
#4362=CARTESIAN_POINT ( 'NONE',  ( 0.000000000000000000, 184.0000000000000000, 7.000000000000000000 ) ) ;
#4363=CARTESIAN_POINT ( 'NONE',  ( 1.035533905932738419, 184.5800000002185186, 9.500000000000003553 ) ) ;
#4365=CARTESIAN_POINT ( 'NONE',  ( 1.864425960470169619, 228.0311117417621745, 6.329243341474429130 ) ) ;
#4371=CARTESIAN_POINT ( 'NONE',  ( -0.8561741729129456191, 184.4999999989074979, 4.933012699999999029 ) ) ;
#4374=EDGE_LOOP ( 'NONE', ( #2327, #4118, #1098, #589 ) ) ;
#4376=CARTESIAN_POINT ( 'NONE',  ( -5.929230630780102373E-16, 186.2000000000000171, 9.500000000000001776 ) ) ;
#4382=CARTESIAN_POINT ( 'NONE',  ( -1.461580736456473684, 184.7499999989074979, 8.461580736456474128 ) ) ;
#4387=CARTESIAN_POINT ( 'NONE',  ( 0.000000000000000000, 187.2933328889893687, 9.583808270834989429 ) ) ;
#4398=ORIENTED_EDGE ( 'NONE', *, *, #5480, .F. ) ;
#4399=CARTESIAN_POINT ( 'NONE',  ( 2.500000000000000444, 184.8499999999999943, 5.964466094067262247 ) ) ;
#4403=CARTESIAN_POINT ( 'NONE',  ( -1.461580736456472795, 185.5499999989075093, 5.538419263543527649 ) ) ;
#4409=CARTESIAN_POINT ( 'NONE',  ( 1.767766952966369098, 188.0699999975965397, 5.232233047033630235 ) ) ;
#4410=CARTESIAN_POINT ( 'NONE',  ( 2.807343268925317492, 227.6302376672054208, 8.330365510804844220 ) ) ;
#4411=CARTESIAN_POINT ( 'NONE',  ( -0.1960076320828026963, 228.2536001344089982, 10.16376666290868336 ) ) ;
#4417=CARTESIAN_POINT ( 'NONE',  ( -1.965116437629976787E-16, 189.6999999978150697, 4.500000000000000000 ) ) ;
#4425=CARTESIAN_POINT ( 'NONE',  ( -1.050320854595332420E-16, 188.2000000000000171, 4.500000000000000000 ) ) ;
#4426=CARTESIAN_POINT ( 'NONE',  ( -0.8219475227482178070, 228.8541360017199224, 8.706184346459185264 ) ) ;
#4430=CARTESIAN_POINT ( 'NONE',  ( 2.500000000000000444, 187.2000000000000171, 7.000000000000000000 ) ) ;
#4433=ORIENTED_EDGE ( 'NONE', *, *, #5650, .T. ) ;
#4438=CARTESIAN_POINT ( 'NONE',  ( -0.7711655121432159365, 228.2232134260211183, 10.07446308542475499 ) ) ;
#4439=( NAMED_UNIT ( * ) SI_UNIT ( $, .STERADIAN. ) SOLID_ANGLE_UNIT ( ) );
#4441=CARTESIAN_POINT ( 'NONE',  ( -2.500000000000000444, 185.1800000002184561, 8.035533905932737753 ) ) ;
#4442=CARTESIAN_POINT ( 'NONE',  ( -1.592078987458502848, 227.8601693307692813, 5.835551908609170724 ) ) ;
#4443=CARTESIAN_POINT ( 'NONE',  ( 1.159630251547017377, 228.7900363578050928, 8.521060918829135744 ) ) ;
#4448=CARTESIAN_POINT ( 'NONE',  ( 2.066987299999999639, 189.2999999989075377, 6.143825827087054492 ) ) ;
#4454=CARTESIAN_POINT ( 'NONE',  ( 0.8561741729129461742, 185.0999999989074922, 9.066987299999999195 ) ) ;
#4456=CARTESIAN_POINT ( 'NONE',  ( 1.461580736456472795, 185.7499999989074979, 8.461580736456474128 ) ) ;
#4460=CARTESIAN_POINT ( 'NONE',  ( -5.999999999999999112, 189.3270225533669020, 3.938484906660875584 ) ) ;
#4467=ORIENTED_EDGE ( 'NONE', *, *, #14690, .F. ) ;
#4471=ORIENTED_EDGE ( 'NONE', *, *, #8071, .T. ) ;
#4475=CARTESIAN_POINT ( 'NONE',  ( -2.500000000000000888, 188.2999999978150356, 7.000000000000000000 ) ) ;
#4482=CARTESIAN_POINT ( 'NONE',  ( 2.990428124265142706, 227.2109326449624120, 7.096232946303270950 ) ) ;
#4483=( BOUNDED_SURFACE ( )  B_SPLINE_SURFACE ( 1, 2, ( 
 ( #3063, #4257, #592, #5462, #12756, #6658, #4852, #2608, #9627, #8436, #12307, #1332, #5964, #2536, #14379, #3720, #2453, #8597, #4929, #7316, #14545, #13348, #4691, #2370, #8672, #5884, #3642, #64, #1176, #8518, #2288, #11042, #12077, #10731, #7465, #15589, #12156, #6044, #3484, #6205, #4531, #8355, #140, #5005, #9541, #14467, #4769, #13192, #7160, #3566, #7238, #10808, #9858, #14710, #13503, #10966, #11997, #9784, #7389, #10891, #3798, #13272, #1254, #1101, #9708, #15668, #6130, #14630, #13432, #12231, #7621, #1643, #1719, #224, #2849, #12546, #13577, #7539, #5083, #10089, #4115, #1567, #2926, #2768, #451, #10247, #12465, #6363, #12385, #9934, #15022, #4031, #2686, #3872, #7697, #7860, #14786, #1484, #11199, #5160, #299 ),
 ( #8986, #8824, #10014, #8745, #3949, #14861, #13652, #6443, #6519, #11276, #375, #5243, #14939, #13814, #5323, #8906, #13741, #11353, #10167, #7775, #6594, #12622, #11429, #5399, #529, #15098, #4194, #9064, #13890, #3002, #1405, #6280, #11120, #1797, #6907, #9138, #14273, #1875, #15252, #10401, #10322, #4353, #9212, #10553, #14123, #11742, #4272, #5554, #8171, #4591, #11812, #916, #5632, #9287, #6672, #14047, #1954, #3311, #3156, #15409, #12851, #12771, #9362, #681, #4430, #9442, #766, #8011, #2032, #6750, #6829, #7928, #11665, #13011, #10479, #3229, #11505, #15333, #15495, #3383, #8095, #844, #12933, #5709, #13973, #2111, #4507, #606, #12701, #5478, #14203, #6983, #15173, #5786, #10632, #3079, #11583, #8064, #2082, #7111, #14024 ) ),
 .UNSPECIFIED., .F., .F., .F. ) 
 B_SPLINE_SURFACE_WITH_KNOTS ( ( 2, 2 ),
 ( 3, 2, 2, 2, 2, 2, 2, 2, 2, 2, 2, 2, 2, 2, 2, 2, 2, 2, 2, 2, 2, 2, 2, 2, 2, 2, 2, 2, 2, 2, 2, 2, 2, 2, 2, 2, 2, 2, 2, 2, 2, 2, 2, 2, 2, 2, 2, 2, 2, 2, 3 ),
 ( 0.000000000000000000, 1.000000000000000000 ),
 ( 0.000000000000000000, 0.01785714285714285615, 0.03571428571428571230, 0.05357142857142856845, 0.07142857142857142461, 0.08928571428571428770, 0.1071428571428571369, 0.1250000000000000000, 0.1428571428571428492, 0.1607142857142857262, 0.1785714285714285754, 0.1964285714285714246, 0.2142857142857142738, 0.2321428571428571508, 0.2500000000000000000, 0.2678571428571428492, 0.2857142857142856984, 0.3035714285714285476, 0.3214285714285714524, 0.3392857142857143016, 0.3571428571428571508, 0.3750000000000000000, 0.3928571428571428492, 0.4107142857142856984, 0.4285714285714285476, 0.4464285714285714524, 0.4642857142857143016, 0.4821428571428571508, 0.5000000000000000000, 0.5178571428571429047, 0.5357142857142856984, 0.5535714285714286031, 0.5714285714285713969, 0.5892857142857143016, 0.6071428571428570953, 0.6250000000000000000, 0.6428571428571429047, 0.6607142857142856984, 0.6785714285714286031, 0.6964285714285713969, 0.7142857142857143016, 0.7321428571428570953, 0.7500000000000000000, 0.7678571428571429047, 0.7857142857142856984, 0.8035714285714286031, 0.8214285714285713969, 0.8392857142857143016, 0.8571428571428570953, 0.8750000000000000000, 0.8928571428571429047 ),
 .UNSPECIFIED. ) 
 GEOMETRIC_REPRESENTATION_ITEM ( )  RATIONAL_B_SPLINE_SURFACE ( (
 ( 1.000000000000000000, 0.9238795325112867385, 1.000000000000000000, 0.9238795325112867385, 1.000000000000000000, 0.9238795325112867385, 1.000000000000000000, 0.9238795325112867385, 1.000000000000000000, 0.9238795325112867385, 1.000000000000000000, 0.9238795325112867385, 1.000000000000000000, 0.9238795325112867385, 1.000000000000000000, 0.9238795325112867385, 1.000000000000000000, 0.9238795325112867385, 1.000000000000000000, 0.9238795325112867385, 1.000000000000000000, 0.9238795325112867385, 1.000000000000000000, 0.9238795325112867385, 1.000000000000000000, 0.9238795325112867385, 1.000000000000000000, 0.9238795325112867385, 1.000000000000000000, 0.9238795325112867385, 1.000000000000000000, 0.9238795325112867385, 1.000000000000000000, 0.9238795325112867385, 1.000000000000000000, 0.9238795325112867385, 1.000000000000000000, 0.9238795325112867385, 1.000000000000000000, 0.9238795325112867385, 1.000000000000000000, 0.9238795325112867385, 1.000000000000000000, 0.9238795325112867385, 1.000000000000000000, 0.9238795325112867385, 1.000000000000000000, 0.9238795325112867385, 1.000000000000000000, 0.9238795325112867385, 1.000000000000000000, 0.9238795325112867385, 1.000000000000000000, 0.9238795325112867385, 1.000000000000000000, 0.9238795325112867385, 1.000000000000000000, 0.9238795325112867385, 1.000000000000000000, 0.9238795325112867385, 1.000000000000000000, 0.9238795325112867385, 1.000000000000000000, 0.9238795325112867385, 1.000000000000000000, 0.9238795325112867385, 1.000000000000000000, 0.9238795325112867385, 1.000000000000000000, 0.9238795325112867385, 1.000000000000000000, 0.9238795325112867385, 1.000000000000000000, 0.9238795325112867385, 1.000000000000000000, 0.9238795325112867385, 1.000000000000000000, 0.9238795325112867385, 1.000000000000000000, 0.9238795325112867385, 1.000000000000000000, 0.9238795325112867385, 1.000000000000000000, 0.9238795325112867385, 1.000000000000000000, 0.9238795325112867385, 1.000000000000000000, 0.9238795325112867385, 1.000000000000000000, 0.9238795325112867385, 1.000000000000000000, 0.9238795325112867385, 1.000000000000000000, 0.9238795325112867385, 1.000000000000000000, 0.9238795325112867385, 1.000000000000000000, 0.9238795325112867385, 1.000000000000000000, 0.9238795325112867385, 1.000000000000000000),
 ( 1.000000000000000000, 0.9238795325112867385, 1.000000000000000000, 0.9238795325112867385, 1.000000000000000000, 0.9238795325112867385, 1.000000000000000000, 0.9238795325112867385, 1.000000000000000000, 0.9238795325112867385, 1.000000000000000000, 0.9238795325112867385, 1.000000000000000000, 0.9238795325112867385, 1.000000000000000000, 0.9238795325112867385, 1.000000000000000000, 0.9238795325112867385, 1.000000000000000000, 0.9238795325112867385, 1.000000000000000000, 0.9238795325112867385, 1.000000000000000000, 0.9238795325112867385, 1.000000000000000000, 0.9238795325112867385, 1.000000000000000000, 0.9238795325112867385, 1.000000000000000000, 0.9238795325112867385, 1.000000000000000000, 0.9238795325112867385, 1.000000000000000000, 0.9238795325112867385, 1.000000000000000000, 0.9238795325112867385, 1.000000000000000000, 0.9238795325112867385, 1.000000000000000000, 0.9238795325112867385, 1.000000000000000000, 0.9238795325112867385, 1.000000000000000000, 0.9238795325112867385, 1.000000000000000000, 0.9238795325112867385, 1.000000000000000000, 0.9238795325112867385, 1.000000000000000000, 0.9238795325112867385, 1.000000000000000000, 0.9238795325112867385, 1.000000000000000000, 0.9238795325112867385, 1.000000000000000000, 0.9238795325112867385, 1.000000000000000000, 0.9238795325112867385, 1.000000000000000000, 0.9238795325112867385, 1.000000000000000000, 0.9238795325112867385, 1.000000000000000000, 0.9238795325112867385, 1.000000000000000000, 0.9238795325112867385, 1.000000000000000000, 0.9238795325112867385, 1.000000000000000000, 0.9238795325112867385, 1.000000000000000000, 0.9238795325112867385, 1.000000000000000000, 0.9238795325112867385, 1.000000000000000000, 0.9238795325112867385, 1.000000000000000000, 0.9238795325112867385, 1.000000000000000000, 0.9238795325112867385, 1.000000000000000000, 0.9238795325112867385, 1.000000000000000000, 0.9238795325112867385, 1.000000000000000000, 0.9238795325112867385, 1.000000000000000000, 0.9238795325112867385, 1.000000000000000000, 0.9238795325112867385, 1.000000000000000000, 0.9238795325112867385, 1.000000000000000000, 0.9238795325112867385, 1.000000000000000000, 0.9238795325112867385, 1.000000000000000000, 0.9238795325112867385, 1.000000000000000000, 0.9238795325112867385, 1.000000000000000000) ) ) 
 REPRESENTATION_ITEM ( '' )  SURFACE ( )  );
#4490=CARTESIAN_POINT ( 'NONE',  ( -2.500000000000000888, 189.0999999978150470, 7.000000000000000000 ) ) ;
#4501=CARTESIAN_POINT ( 'NONE',  ( -2.500000000000000444, 185.9499999978150413, 8.035533905932737753 ) ) ;
#4502=CARTESIAN_POINT ( 'NONE',  ( -1.986723294250032357, 228.3028615258686500, 7.114072217564876510 ) ) ;
#4507=CARTESIAN_POINT ( 'NONE',  ( -1.767766952966369320, 188.2999999999999829, 5.232233047033630235 ) ) ;
#4508=CARTESIAN_POINT ( 'NONE',  ( -2.500000000000000444, 187.4999999978150527, 7.000000000000000000 ) ) ;
#4513=VECTOR ( 'NONE', #6134, 1000.000000000000000 ) ;
#4515=CARTESIAN_POINT ( 'NONE',  ( -2.418857398188632324, 226.7180838673660332, 5.644635841926620934 ) ) ;
#4518=CARTESIAN_POINT ( 'NONE',  ( -1.767766952966369542, 185.2300000002184959, 8.767766952966368876 ) ) ;
#4521=CARTESIAN_POINT ( 'NONE',  ( 1.078411626687468594, 228.8081072869749732, 8.573250792970148026 ) ) ;
#4526=CARTESIAN_POINT ( 'NONE',  ( -6.877907531704918753E-16, 189.0499999989075093, 9.066987300000000971 ) ) ;
#4531=CARTESIAN_POINT ( 'NONE',  ( -2.066987300000000527, 186.2499999989074979, 7.000000000000000000 ) ) ;
#4537=CARTESIAN_POINT ( 'NONE',  ( 0.8561741729129457301, 185.1999999989075434, 4.933012699999999029 ) ) ;
#4542=CARTESIAN_POINT ( 'NONE',  ( 3.659182332138577465E-16, 227.2817795252328210, 4.165129161027028459 ) ) ;
#4553=CARTESIAN_POINT ( 'NONE',  ( 2.066987300000000083, 185.2999999989075661, 6.143825827087054492 ) ) ;
#4554=CARTESIAN_POINT ( 'NONE',  ( 1.990438725498679062, 228.3461478020684865, 7.239085452117288710 ) ) ;
#4560=CARTESIAN_POINT ( 'NONE',  ( 2.066987300000000083, 185.2999999989075377, 6.143825827087054492 ) ) ;
#4565=CARTESIAN_POINT ( 'NONE',  ( -1.767766952966369320, 188.2699999975965568, 5.232233047033630235 ) ) ;
#4566=CARTESIAN_POINT ( 'NONE',  ( -0.9651034952757481244, 226.3762748196293728, 4.637298184581183591 ) ) ;
#4586=CARTESIAN_POINT ( 'NONE',  ( -1.767766952966369542, 185.9999999978150527, 8.767766952966368876 ) ) ;
#4587=CARTESIAN_POINT ( 'NONE',  ( 0.9648499430152943646, 228.2043505555869274, 10.01897217821435859 ) ) ;
#4589=CARTESIAN_POINT ( 'NONE',  ( -2.251711471503315298, 189.9958096512905286, 5.235413736675446295 ) ) ;
#4591=CARTESIAN_POINT ( 'NONE',  ( 2.500000000000000444, 186.4500000000000171, 5.964466094067262247 ) ) ;
#4597=CARTESIAN_POINT ( 'NONE',  ( -6.776263578034402713E-18, 186.5999999999999943, 4.500000000000000000 ) ) ;
#4598=CARTESIAN_POINT ( 'NONE',  ( -2.791088703906231760, 226.9357700049156108, 6.285935106528314442 ) ) ;
#4599=SHAPE_REPRESENTATION_RELATIONSHIP ( 'NONE' , 'NONE' ,  #11283, #8222 ) ;
#4601=CARTESIAN_POINT ( 'NONE',  ( 1.035533905932737975, 184.8800000002185016, 4.500000000000000888 ) ) ;
#4603=CARTESIAN_POINT ( 'NONE',  ( 0.9944270131901197241, 228.8248696211178981, 8.621661370035813121 ) ) ;
#4616=CARTESIAN_POINT ( 'NONE',  ( -2.066987300000000527, 185.4499999989075150, 7.000000000000000000 ) ) ;
#4620=CARTESIAN_POINT ( 'NONE',  ( -5.999999999999999112, 215.7452399395091618, 13.29567785264566027 ) ) ;
#4623=CARTESIAN_POINT ( 'NONE',  ( 0.000000000000000000, 189.6977690162252657, 10.38967773564543862 ) ) ;
#4635=CARTESIAN_POINT ( 'NONE',  ( -5.895349312889930360E-16, 187.4499999989075150, 9.066987300000000971 ) ) ;
#4638=CARTESIAN_POINT ( 'NONE',  ( 2.500000000000000444, 185.5499999978150356, 5.964466094067262247 ) ) ;
#4642=CARTESIAN_POINT ( 'NONE',  ( 1.328920255623610380, 226.4243263863947391, 4.778947530392284371 ) ) ;
#4644=CARTESIAN_POINT ( 'NONE',  ( -1.748661130334981051, 228.0746845563984095, 9.637707355516731411 ) ) ;
#4664=CARTESIAN_POINT ( 'NONE',  ( 2.500000000000000444, 189.5499999978150640, 5.964466094067262247 ) ) ;
#4665=CARTESIAN_POINT ( 'NONE',  ( 1.707343418157801551, 228.0835877007203294, 9.663887492166837845 ) ) ;
#4674=CARTESIAN_POINT ( 'NONE',  ( 2.244217608389459162, 226.6470584425424306, 5.435389493528692384 ) ) ;
#4678=CARTESIAN_POINT ( 'NONE',  ( -2.882630993546674070, 227.5642217159421818, 8.136181965847606889 ) ) ;
#4679=( NAMED_UNIT ( * ) SI_UNIT ( $, .STERADIAN. ) SOLID_ANGLE_UNIT ( ) );
#4681=CARTESIAN_POINT ( 'NONE',  ( 0.4899822127396957772, 190.0840757508179593, 4.235790927168524789 ) ) ;
#4682=CARTESIAN_POINT ( 'NONE',  ( -1.767766952966369320, 185.8300000002185186, 5.232233047033630235 ) ) ;
#4684=CARTESIAN_POINT ( 'NONE',  ( -1.965306002007385144, 228.1545512627131131, 6.685743718507844768 ) ) ;
#4690=CARTESIAN_POINT ( 'NONE',  ( 2.066987300000000971, 187.4999999989075548, 6.143825827087054492 ) ) ;
#4691=CARTESIAN_POINT ( 'NONE',  ( -1.461580736456473018, 185.3499999989074922, 5.538419263543526760 ) ) ;
#4694=( BOUNDED_CURVE ( )  B_SPLINE_CURVE ( 2, ( #13313, #31, #7122, #2253, #2170, #11874, #9752, #14590, #3686 ),
 .UNSPECIFIED., .F., .F. ) 
 B_SPLINE_CURVE_WITH_KNOTS ( ( 3, 2, 2, 2, 3 ),
 ( 0.2142857142857143293, 0.2321428571428572063, 0.2500000000000000000, 0.2678571428571428492, 0.2857142857142856984 ),
 .UNSPECIFIED. ) 
 CURVE ( )  GEOMETRIC_REPRESENTATION_ITEM ( )  RATIONAL_B_SPLINE_CURVE ( ( 0.9999999999999997780, 0.9238795325112869605, 1.000000000000000000, 0.9238795325112867385, 1.000000000000000000, 0.9238795325112867385, 1.000000000000000000, 0.9238795325112867385, 1.000000000000000000 ) ) 
 REPRESENTATION_ITEM ( '' )  );
#4699=CARTESIAN_POINT ( 'NONE',  ( -5.793705359219414319E-16, 187.2499999989075263, 9.066987300000000971 ) ) ;
#4703=CARTESIAN_POINT ( 'NONE',  ( 1.035533905932737975, 184.1499999999999773, 4.500000000000001776 ) ) ;
#4704=CARTESIAN_POINT ( 'NONE',  ( 1.035533905932737753, 188.8499999978150186, 4.500000000000001776 ) ) ;
#4706=CARTESIAN_POINT ( 'NONE',  ( -0.06431340346706571065, 189.6978264018315770, 10.38900192207087336 ) ) ;
#4711=CARTESIAN_POINT ( 'NONE',  ( 1.728762592943754006, 227.9346299510661140, 6.050598426982102040 ) ) ;
#4717=CARTESIAN_POINT ( 'NONE',  ( -0.8561741729129469514, 188.1999999989075150, 9.066987299999999195 ) ) ;
#4719=LINE ( 'NONE', #2005, #15317 ) ;
#4724=CARTESIAN_POINT ( 'NONE',  ( -0.7768053109583262783, 226.3575155338836282, 4.581995736916623763 ) ) ;
#4732=EDGE_CURVE ( 'NONE', #7444, #6574, #2468, .T. ) ;
#4743=CARTESIAN_POINT ( 'NONE',  ( -1.035533905932737975, 188.1499999978150868, 4.500000000000000888 ) ) ;
#4744=CARTESIAN_POINT ( 'NONE',  ( 2.990428124265142706, 227.2109326449624120, 7.096232946303270950 ) ) ;
#4754=CARTESIAN_POINT ( 'NONE',  ( 0.6751155222935361078, 226.3493740387523587, 4.557952239717714349 ) ) ;
#4757=CARTESIAN_POINT ( 'NONE',  ( -2.773170890423259483, 226.9215440165780535, 6.244038878397168091 ) ) ;
#4759=CARTESIAN_POINT ( 'NONE',  ( -2.500000000000000444, 188.2800000002184788, 5.964466094067261359 ) ) ;
#4761=APPLICATION_CONTEXT ( 'automotive_design' ) ;
#4762=CARTESIAN_POINT ( 'NONE',  ( 1.080575604060385553, 227.7131986584202821, 5.411092224208442936 ) ) ;
#4763=FACE_OUTER_BOUND ( 'NONE', #6887, .T. ) ;
#4767=CARTESIAN_POINT ( 'NONE',  ( 1.461580736456473240, 187.5499999989075093, 5.538419263543526760 ) ) ;
#4769=CARTESIAN_POINT ( 'NONE',  ( 1.461580736456472573, 186.5499999989075093, 8.461580736456474128 ) ) ;
#4778=CARTESIAN_POINT ( 'NONE',  ( 2.066987300000000527, 186.6999999989075150, 6.143825827087054492 ) ) ;
#4790=VERTEX_POINT ( 'NONE', #14258 ) ;
#4791=CARTESIAN_POINT ( 'NONE',  ( 1.789766218952369536, 227.9720476933883049, 6.158663000976825508 ) ) ;
#4799=CARTESIAN_POINT ( 'NONE',  ( 2.066987300000000083, 186.0999999989075206, 6.143825827087054492 ) ) ;
#4804=CARTESIAN_POINT ( 'NONE',  ( -2.381852405317018029, 227.8773184320497478, 9.057252860304588538 ) ) ;
#4809=CARTESIAN_POINT ( 'NONE',  ( -5.861467994999758346E-16, 186.0999999978150754, 9.500000000000001776 ) ) ;
#4824=CARTESIAN_POINT ( 'NONE',  ( 2.500000000000000000, 188.6999999978150697, 7.000000000000000000 ) ) ;
#4825=CARTESIAN_POINT ( 'NONE',  ( 2.257611286988003396, 226.6535225833466427, 5.454435118953909978 ) ) ;
#4827=CARTESIAN_POINT ( 'NONE',  ( -1.329739968339264777, 189.0000000001359979, 4.875166081584925593 ) ) ;
#4831=CARTESIAN_POINT ( 'NONE',  ( -2.066760391300492827E-16, 189.4499999989075150, 4.933012699999999029 ) ) ;
#4838=CARTESIAN_POINT ( 'NONE',  ( -2.586818446948293104, 227.7795406139177032, 8.769651989551642046 ) ) ;
#4843=CARTESIAN_POINT ( 'NONE',  ( -9.825582188149883933E-17, 188.1300000002185016, 4.500000000000000000 ) ) ;
#4846=CARTESIAN_POINT ( 'NONE',  ( 0.9944270131901197241, 228.8248696211178981, 8.621661370035813121 ) ) ;
#4850=ORIENTED_EDGE ( 'NONE', *, *, #968, .F. ) ;
#4851=CARTESIAN_POINT ( 'NONE',  ( 1.461580736456472573, 188.9499999989075150, 8.461580736456474128 ) ) ;
#4852=CARTESIAN_POINT ( 'NONE',  ( -1.461580736456473018, 184.5499999989075093, 5.538419263543526760 ) ) ;
#4855=CARTESIAN_POINT ( 'NONE',  ( 0.05308131560460233739, 189.7622414119611847, 5.148053411033613358 ) ) ;
#4863=CARTESIAN_POINT ( 'NONE',  ( 0.000000000000000000, 184.0000000000000000, 7.000000000000000000 ) ) ;
#4864=CARTESIAN_POINT ( 'NONE',  ( 2.066987300000000527, 184.3499999989074922, 7.000000000000000000 ) ) ;
#4878=CARTESIAN_POINT ( 'NONE',  ( 2.066987300000000083, 186.0499999989075093, 7.000000000000000000 ) ) ;
#4885=CARTESIAN_POINT ( 'NONE',  ( -1.979540121751099724, 226.5646310999674427, 5.192482286045976281 ) ) ;
#4905=CARTESIAN_POINT ( 'NONE',  ( 2.500000000000000444, 187.1499999978150868, 5.964466094067262247 ) ) ;
#4906=CARTESIAN_POINT ( 'NONE',  ( -0.1001789588503840533, 226.3251931448050698, 4.486704830075608719 ) ) ;
#4908=CARTESIAN_POINT ( 'NONE',  ( -2.488587570294162443, 189.3796024022271922, 5.337940027815102795 ) ) ;
#4915=CARTESIAN_POINT ( 'NONE',  ( 0.3831815474498145857, 226.3309662840062515, 4.503685043354857420 ) ) ;
#4922=CARTESIAN_POINT ( 'NONE',  ( 2.500000000000000444, 187.1300000002185016, 7.000000000000000000 ) ) ;
#4924=CARTESIAN_POINT ( 'NONE',  ( 1.965304387191771029, 228.1545866171788930, 6.685845824222668377 ) ) ;
#4929=CARTESIAN_POINT ( 'NONE',  ( 1.461580736456473462, 185.1499999989075320, 5.538419263543526760 ) ) ;
#4938=CARTESIAN_POINT ( 'NONE',  ( 5.999999999999999112, 186.5669965222008670, 9.317226423031115701 ) ) ;
#4941=CARTESIAN_POINT ( 'NONE',  ( 0.1189749320691910750, 189.0435645138963139, 10.18765630333474626 ) ) ;
#4952=ADVANCED_FACE ( 'NONE', ( #9009 ), #3973, .T. ) ;
#4957=EDGE_CURVE ( 'NONE', #7973, #12251, #4093, .T. ) ;
#4959=CARTESIAN_POINT ( 'NONE',  ( 0.8561741729129458411, 187.4999999989075548, 9.066987299999999195 ) ) ;
#4967=CARTESIAN_POINT ( 'NONE',  ( -2.990426535912302786, 227.3682058476787233, 7.559219386994686651 ) ) ;
#4973=CARTESIAN_POINT ( 'NONE',  ( 2.388242816781450006, 189.0000000000000000, 6.240296789758633444 ) ) ;
#4981=DIRECTION ( 'NONE',  ( -1.000000000000000000, 0.000000000000000000, 0.000000000000000000 ) ) ;
#4983=CARTESIAN_POINT ( 'NONE',  ( -1.767766952966369320, 187.3999999978150584, 5.232233047033630235 ) ) ;
#4984=CARTESIAN_POINT ( 'NONE',  ( 2.923059718105053051, 227.5089953743221258, 7.973592892444406388 ) ) ;
#4986=CARTESIAN_POINT ( 'NONE',  ( -1.135771517436445111, 189.0000000004517631, 9.231728281961022020 ) ) ;
#4990=CARTESIAN_POINT ( 'NONE',  ( 2.500000000000000000, 188.0000000000000000, 7.000000000000000000 ) ) ;
#4992=CARTESIAN_POINT ( 'NONE',  ( 1.815011834558647452, 226.5209060679430308, 5.063596875652942586 ) ) ;
#4998=CARTESIAN_POINT ( 'NONE',  ( 1.767766952966368432, 187.8300000002184902, 8.767766952966368876 ) ) ;
#5000=CARTESIAN_POINT ( 'NONE',  ( 1.558909820229182230, 228.6656996696739554, 8.161969471806774123 ) ) ;
#5005=CARTESIAN_POINT ( 'NONE',  ( -0.8561741729129470624, 186.3999999989075320, 9.066987300000000971 ) ) ;
#5007=CARTESIAN_POINT ( 'NONE',  ( -0.8561741729129467293, 185.7999999989075093, 9.066987299999999195 ) ) ;
#5013=CARTESIAN_POINT ( 'NONE',  ( 5.999999999999999112, 215.0542865858234336, 7.296348638370669271 ) ) ;
#5014=CARTESIAN_POINT ( 'NONE',  ( -2.434916734102785085, 189.0000000000000000, 7.580643601937843812 ) ) ;
#5021=EDGE_CURVE ( 'NONE', #2326, #10913, #15043, .T. ) ;
#5030=CARTESIAN_POINT ( 'NONE',  ( -1.461580736456473906, 188.7499999989075263, 8.461580736456474128 ) ) ;
#5041=CARTESIAN_POINT ( 'NONE',  ( -2.809592974547592714, 227.6294044507834542, 8.327915135215583575 ) ) ;
#5057=CARTESIAN_POINT ( 'NONE',  ( -1.035533905932737975, 186.6199999975965511, 4.500000000000000888 ) ) ;
#5058=CARTESIAN_POINT ( 'NONE',  ( 0.6422548253168780530, 227.6434438162357878, 5.209636261422765813 ) ) ;
#5060=CARTESIAN_POINT ( 'NONE',  ( 2.550395957922052759, 226.7806086135062458, 5.828878098564913124 ) ) ;
#5061=CARTESIAN_POINT ( 'NONE',  ( -2.662230360837048337, 189.2020403679304366, 8.562491460291731471 ) ) ;
#5069=CARTESIAN_POINT ( 'NONE',  ( 2.228329245637216793, 227.9362088727311857, 9.230470988095557772 ) ) ;
#5071=EDGE_CURVE ( 'NONE', #12251, #10913, #2979, .T. ) ;
#5076=CARTESIAN_POINT ( 'NONE',  ( -6.369687763352338550E-16, 186.9300000002185129, 9.500000000000001776 ) ) ;
#5077=CARTESIAN_POINT ( 'NONE',  ( 1.862843374206504254, 228.4903663355887318, 7.655596802610238782 ) ) ;
#5083=CARTESIAN_POINT ( 'NONE',  ( 1.461580736456472573, 188.1499999989075036, 8.461580736456474128 ) ) ;
#5092=CARTESIAN_POINT ( 'NONE',  ( 0.07962197837297851910, 190.0874091994478761, 4.202769589527710181 ) ) ;
#5102=CARTESIAN_POINT ( 'NONE',  ( 2.066987300000000083, 187.6499999989075320, 7.000000000000000000 ) ) ;
#5110=CARTESIAN_POINT ( 'NONE',  ( -2.246716568442826745, 227.9318189537954993, 9.217556643805876249 ) ) ;
#5118=CARTESIAN_POINT ( 'NONE',  ( -2.623350778723538834, 226.8212935938476278, 5.948734516926445615 ) ) ;
#5124=CARTESIAN_POINT ( 'NONE',  ( 1.458225638478870767, 188.9999999999999716, 4.936243315740555637 ) ) ;
#5131=CARTESIAN_POINT ( 'NONE',  ( 2.500000000000000444, 187.8499999978150470, 8.035533905932739529 ) ) ;
#5132=CARTESIAN_POINT ( 'NONE',  ( 1.035533905932737975, 185.6499999978150868, 4.500000000000000888 ) ) ;
#5136=CARTESIAN_POINT ( 'NONE',  ( 1.035533905932738419, 186.2199999975965738, 9.500000000000003553 ) ) ;
#5137=CARTESIAN_POINT ( 'NONE',  ( -1.313542798833678749, 227.7708088449086290, 5.577473728656160645 ) ) ;
#5138=CARTESIAN_POINT ( 'NONE',  ( -1.240485740468941556, 226.4108687305035232, 4.739277288743133809 ) ) ;
#5140=CARTESIAN_POINT ( 'NONE',  ( -2.778918535561691439, 189.3544729152338846, 5.892260229556007367 ) ) ;
#5147=CARTESIAN_POINT ( 'NONE',  ( 2.999875809771047397, 227.2791568961600319, 7.297085794927967939 ) ) ;
#5153=CARTESIAN_POINT ( 'NONE',  ( 1.035533905932737975, 184.9499999999999886, 4.500000000000000888 ) ) ;
#5155=CARTESIAN_POINT ( 'NONE',  ( 0.8230742150784297051, 227.6668866512619047, 5.277340506070477666 ) ) ;
#5160=CARTESIAN_POINT ( 'NONE',  ( 0.8561741729129455081, 189.1999999989075434, 4.933012699999999029 ) ) ;
#5162=CARTESIAN_POINT ( 'NONE',  ( -5.421010862427522170E-16, 186.6499999989075320, 9.066987300000000971 ) ) ;
#5168=CARTESIAN_POINT ( 'NONE',  ( -1.456896669277396583E-16, 188.4499999989075150, 4.933012699999999029 ) ) ;
#5170=CARTESIAN_POINT ( 'NONE',  ( 2.471008584805455488, 189.0000000025389397, 6.581706668861207810 ) ) ;
#5173=CARTESIAN_POINT ( 'NONE',  ( 2.266383616481251195, 189.7755269081602876, 9.339276568968184478 ) ) ;
#5178=CARTESIAN_POINT ( 'NONE',  ( 0.8561741729129460632, 185.8999999989075036, 9.066987299999999195 ) ) ;
#5181=B_SPLINE_CURVE_WITH_KNOTS ( 'NONE', 3,
 ( #14719, #6289, #8681, #2544, #14795, #7324, #7398, #5014, #12240, #12084, #11051, #6216, #3959, #73, #3650, #1262, #9868, #952, #13511, #7475, #12319, #6138 ),
 .UNSPECIFIED., .F., .F.,
 ( 4, 2, 2, 2, 2, 2, 2, 2, 2, 2, 4 ),
 ( 0.8845854629958906923, 0.9326205154887873272, 0.9806555679816839621, 1.028690620474580708, 1.052708146721028859, 1.076725672967477232, 1.124760725460373534, 1.148778251706821907, 1.172795777953270280, 1.220830830446166804, 1.268865882939063106 ),
 .UNSPECIFIED. ) ;
#5187=CARTESIAN_POINT ( 'NONE',  ( -0.9748673250649166899, 190.0717113996746264, 4.361044512588190258 ) ) ;
#5189=AXIS2_PLACEMENT_3D ( 'NONE', #9623, #13189, #7155 ) ;
#5191=CARTESIAN_POINT ( 'NONE',  ( 0.000000000000000000, 202.2378330312726291, 13.30884679668974258 ) ) ;
#5205=( BOUNDED_SURFACE ( )  B_SPLINE_SURFACE ( 3, 3, ( 
 ( #12880, #15284, #4387, #9241, #2063, #8124, #15521, #6860 ),
 ( #11696, #14076, #11769, #11841, #10661, #15206, #14304, #5819 ),
 ( #2138, #15364, #3186, #10433, #5507, #11615, #1987, #14155 ),
 ( #796, #5739, #5662, #872, #7964, #14002, #3413, #4542 ),
 ( #10351, #10582, #4460, #13041, #9315, #9392, #3258, #14230 ),
 ( #4305, #3337, #951, #7011, #8205, #4620, #13118, #716 ),
 ( #8284, #9473, #2219, #7090, #1907, #9167, #3110, #12804 ) ),
 .UNSPECIFIED., .T., .F., .F. ) 
 B_SPLINE_SURFACE_WITH_KNOTS ( ( 4, 3, 4 ),
 ( 4, 2, 2, 4 ),
 ( 0.000000000000000000, 0.5000000000000000000, 1.000000000000000000 ),
 ( 0.000000000000000000, 0.05225677727458622607, 0.5261283886372931651, 1.000000000000000000 ),
 .UNSPECIFIED. ) 
 GEOMETRIC_REPRESENTATION_ITEM ( )  RATIONAL_B_SPLINE_SURFACE ( (
 ( 1.000000000000000000, 1.000000000000000000, 1.000000000000000000, 1.000000000000000000, 1.000000000000000000, 1.000000000000000000, 1.000000000000000000, 1.000000000000000000),
 ( 0.3333333333333333703, 0.3333333333333333703, 0.3333333333333333703, 0.3333333333333333703, 0.3333333333333333703, 0.3333333333333333703, 0.3333333333333333703, 0.3333333333333333703),
 ( 0.3333333333333333703, 0.3333333333333333703, 0.3333333333333333703, 0.3333333333333333703, 0.3333333333333333703, 0.3333333333333333703, 0.3333333333333333703, 0.3333333333333333703),
 ( 1.000000000000000000, 1.000000000000000000, 1.000000000000000000, 1.000000000000000000, 1.000000000000000000, 1.000000000000000000, 1.000000000000000000, 1.000000000000000000),
 ( 0.3333333333333333703, 0.3333333333333333703, 0.3333333333333333703, 0.3333333333333333703, 0.3333333333333333703, 0.3333333333333333703, 0.3333333333333333703, 0.3333333333333333703),
 ( 0.3333333333333333703, 0.3333333333333333703, 0.3333333333333333703, 0.3333333333333333703, 0.3333333333333333703, 0.3333333333333333703, 0.3333333333333333703, 0.3333333333333333703),
 ( 1.000000000000000000, 1.000000000000000000, 1.000000000000000000, 1.000000000000000000, 1.000000000000000000, 1.000000000000000000, 1.000000000000000000, 1.000000000000000000) ) ) 
 REPRESENTATION_ITEM ( '' )  SURFACE ( )  );
#5211=CARTESIAN_POINT ( 'NONE',  ( -2.500000000000000444, 185.8499999978150754, 5.964466094067261359 ) ) ;
#5217=CARTESIAN_POINT ( 'NONE',  ( 2.500000000000000444, 187.2199999975966023, 5.964466094067262247 ) ) ;
#5218=CARTESIAN_POINT ( 'NONE',  ( -1.914314807121730633, 228.0813985855225212, 6.474474614426593888 ) ) ;
#5219=CARTESIAN_POINT ( 'NONE',  ( -1.329004440443209090, 226.4243434115648199, 4.778997713384572243 ) ) ;
#5220=( BOUNDED_SURFACE ( )  B_SPLINE_SURFACE ( 3, 3, ( 
 ( #7473, #2460, #11050, #7323, #8605, #2618, #12163, #6137 ),
 ( #7166, #4938, #9790, #14639, #13439, #2543, #14387, #1107 ),
 ( #14718, #1340, #15676, #5971, #6215, #5013, #9632, #3807 ),
 ( #12318, #7782, #5250, #11360, #12472, #12629, #1573, #3957 ),
 ( #7629, #14868, #8832, #13662, #12552, #7704, #8753, #381 ),
 ( #9071, #6601, #14794, #1493, #10253, #3880, #13898, #5405 ),
 ( #1727, #14949, #2775, #11437, #10096, #13822, #15105, #13747 ) ),
 .UNSPECIFIED., .T., .F., .F. ) 
 B_SPLINE_SURFACE_WITH_KNOTS ( ( 4, 3, 4 ),
 ( 4, 2, 2, 4 ),
 ( 0.000000000000000000, 0.5000000000000000000, 1.000000000000000000 ),
 ( 0.000000000000000000, 0.05225677727458622607, 0.5261283886372931651, 1.000000000000000000 ),
 .UNSPECIFIED. ) 
 GEOMETRIC_REPRESENTATION_ITEM ( )  RATIONAL_B_SPLINE_SURFACE ( (
 ( 1.000000000000000000, 1.000000000000000000, 1.000000000000000000, 1.000000000000000000, 1.000000000000000000, 1.000000000000000000, 1.000000000000000000, 1.000000000000000000),
 ( 0.3333333333333333703, 0.3333333333333333703, 0.3333333333333333703, 0.3333333333333333703, 0.3333333333333333703, 0.3333333333333333703, 0.3333333333333333703, 0.3333333333333333703),
 ( 0.3333333333333333703, 0.3333333333333333703, 0.3333333333333333703, 0.3333333333333333703, 0.3333333333333333703, 0.3333333333333333703, 0.3333333333333333703, 0.3333333333333333703),
 ( 1.000000000000000000, 1.000000000000000000, 1.000000000000000000, 1.000000000000000000, 1.000000000000000000, 1.000000000000000000, 1.000000000000000000, 1.000000000000000000),
 ( 0.3333333333333333703, 0.3333333333333333703, 0.3333333333333333703, 0.3333333333333333703, 0.3333333333333333703, 0.3333333333333333703, 0.3333333333333333703, 0.3333333333333333703),
 ( 0.3333333333333333703, 0.3333333333333333703, 0.3333333333333333703, 0.3333333333333333703, 0.3333333333333333703, 0.3333333333333333703, 0.3333333333333333703, 0.3333333333333333703),
 ( 1.000000000000000000, 1.000000000000000000, 1.000000000000000000, 1.000000000000000000, 1.000000000000000000, 1.000000000000000000, 1.000000000000000000, 1.000000000000000000) ) ) 
 REPRESENTATION_ITEM ( '' )  SURFACE ( )  );
#5222=CARTESIAN_POINT ( 'NONE',  ( -1.440803585010799637, 189.7277077271388919, 10.02067490447666920 ) ) ;
#5224=ORIENTED_EDGE ( 'NONE', *, *, #7474, .F. ) ;
#5229=CARTESIAN_POINT ( 'NONE',  ( 2.363458168944469584, 227.8848776677811827, 9.079507460819527864 ) ) ;
#5236=CARTESIAN_POINT ( 'NONE',  ( -2.500000000000000444, 185.2499999999999716, 8.035533905932737753 ) ) ;
#5238=EDGE_CURVE ( 'NONE', #8865, #5590, #1771, .T. ) ;
#5239=CARTESIAN_POINT ( 'NONE',  ( 0.5174937098143853609, 227.6312805367891201, 5.174508016632918483 ) ) ;
#5243=CARTESIAN_POINT ( 'NONE',  ( -1.035533905932739529, 184.5499999999999829, 9.500000000000003553 ) ) ;
#5246=CARTESIAN_POINT ( 'NONE',  ( -1.084202172485504434E-16, 187.8499999989074922, 4.933012699999999029 ) ) ;
#5250=CARTESIAN_POINT ( 'NONE',  ( 3.659182332138577465E-16, 189.3270225533669020, 3.938484906660876472 ) ) ;
#5253=CARTESIAN_POINT ( 'NONE',  ( 2.943069445653888838, 189.3294980521935997, 6.426540498107687682 ) ) ;
#5258=CARTESIAN_POINT ( 'NONE',  ( -1.768703179866833342, 189.0000639513403939, 5.233169770031948609 ) ) ;
#5259=VERTEX_POINT ( 'NONE', #8676 ) ;
#5260=CARTESIAN_POINT ( 'NONE',  ( 1.461580736456473018, 186.1499999989075320, 5.538419263543527649 ) ) ;
#5268=VERTEX_POINT ( 'NONE', #11280 ) ;
#5271=CARTESIAN_POINT ( 'NONE',  ( -0.6743670111594756156, 228.2309373833427344, 10.09717849966832226 ) ) ;
#5272=CARTESIAN_POINT ( 'NONE',  ( -2.066987300000001415, 188.8999999989075320, 7.856174172912944620 ) ) ;
#5281=ORIENTED_EDGE ( 'NONE', *, *, #7474, .T. ) ;
#5294=CARTESIAN_POINT ( 'NONE',  ( -1.767766952966369542, 185.9999999978150527, 8.767766952966368876 ) ) ;
#5298=CARTESIAN_POINT ( 'NONE',  ( -1.035533905932739751, 187.7199999975965738, 9.500000000000003553 ) ) ;
#5299=CARTESIAN_POINT ( 'NONE',  ( 0.7764192831524953098, 228.2223555856212442, 10.07190823357606213 ) ) ;
#5300=CARTESIAN_POINT ( 'NONE',  ( -2.960186505457850892, 227.4470585832885661, 7.791309201570119747 ) ) ;
#5304=CARTESIAN_POINT ( 'NONE',  ( -2.994879556239296026, 189.2754426180449343, 7.463391921200928536 ) ) ;
#5311=CARTESIAN_POINT ( 'NONE',  ( 2.805029955784917206, 227.6318923565098942, 8.335241701881683341 ) ) ;
#5312=VECTOR ( 'NONE', #8096, 1000.000000000000000 ) ;
#5317=CARTESIAN_POINT ( 'NONE',  ( -1.035533905932737975, 187.4499999999999886, 4.500000000000000888 ) ) ;
#5318=CARTESIAN_POINT ( 'NONE',  ( 1.362382138968808887, 227.7849605967929847, 5.618344795260735935 ) ) ;
#5323=CARTESIAN_POINT ( 'NONE',  ( 1.767766952966368654, 184.7000000000000171, 8.767766952966368876 ) ) ;
#5325=CARTESIAN_POINT ( 'NONE',  ( 2.066987299999999639, 188.4499999989075150, 7.000000000000000000 ) ) ;
#5330=DIRECTION ( 'NONE',  ( -6.123233995736766036E-17, 1.000000000000000000, 0.000000000000000000 ) ) ;
#5334=CARTESIAN_POINT ( 'NONE',  ( 2.596699584268322258, 189.8036601807143313, 8.865069138243688585 ) ) ;
#5336=FACE_OUTER_BOUND ( 'NONE', #12809, .T. ) ;
#5338=DIRECTION ( 'NONE',  ( 0.000000000000000000, 1.000000000000000000, 0.000000000000000000 ) ) ;
#5341=CARTESIAN_POINT ( 'NONE',  ( -2.066987300000000527, 188.0499999989075093, 7.000000000000000000 ) ) ;
#5351=CARTESIAN_POINT ( 'NONE',  ( 2.066987299999999639, 189.2499999989075263, 7.000000000000000000 ) ) ;
#5371=CARTESIAN_POINT ( 'NONE',  ( -1.035533905932739751, 186.8499999978150470, 9.500000000000003553 ) ) ;
#5375=CARTESIAN_POINT ( 'NONE',  ( 1.035533905932738419, 185.4199999975965909, 9.500000000000003553 ) ) ;
#5376=CARTESIAN_POINT ( 'NONE',  ( -1.724643626337419855, 228.5864753960848077, 7.933165251024266063 ) ) ;
#5378=CARTESIAN_POINT ( 'NONE',  ( -2.842542329930219491, 227.5997332721124451, 8.240608773874100734 ) ) ;
#5387=CARTESIAN_POINT ( 'NONE',  ( 2.794738844873451811, 227.6405336420577896, 8.360663504027472825 ) ) ;
#5393=CARTESIAN_POINT ( 'NONE',  ( -1.035533905932739751, 186.1500000000000057, 9.500000000000003553 ) ) ;
#5394=CARTESIAN_POINT ( 'NONE',  ( -1.580027211161896261, 227.8635840621947182, 5.845413847729996171 ) ) ;
#5399=CARTESIAN_POINT ( 'NONE',  ( -2.500000000000000444, 185.1500000000000057, 5.964466094067261359 ) ) ;
#5401=CARTESIAN_POINT ( 'NONE',  ( 1.461580736456472795, 186.9499999989075150, 5.538419263543527649 ) ) ;
#5405=CARTESIAN_POINT ( 'NONE',  ( -5.999999999999999112, 229.2449477060184222, 9.834870838912449287 ) ) ;
#5408=CARTESIAN_POINT ( 'NONE',  ( 2.388242814291142047, 188.9999999974610603, 6.240296794481074549 ) ) ;
#5414=CARTESIAN_POINT ( 'NONE',  ( -2.500000000000000444, 186.7999999999999829, 7.000000000000000000 ) ) ;
#5415=ORIENTED_EDGE ( 'NONE', *, *, #2836, .F. ) ;
#5416=CARTESIAN_POINT ( 'NONE',  ( -1.461580736456473018, 187.1499999989075320, 5.538419263543527649 ) ) ;
#5418=VERTEX_POINT ( 'NONE', #12855 ) ;
#5431=CARTESIAN_POINT ( 'NONE',  ( -6.437450399132682577E-16, 187.0000000000000000, 9.500000000000001776 ) ) ;
#5433=CARTESIAN_POINT ( 'NONE',  ( 1.767766952966369320, 186.3999999978150584, 5.232233047033630235 ) ) ;
#5436=ORIENTED_EDGE ( 'NONE', *, *, #8359, .F. ) ;
#5447=CARTESIAN_POINT ( 'NONE',  ( -2.500000000000000444, 188.2499999978150242, 5.964466094067261359 ) ) ;
#5452=CARTESIAN_POINT ( 'NONE',  ( 1.035533905932737753, 188.1199999975965511, 4.500000000000000888 ) ) ;
#5453=CARTESIAN_POINT ( 'NONE',  ( 0.3900692251286368428, 228.2474522196246767, 10.14569219465573546 ) ) ;
#5454=CARTESIAN_POINT ( 'NONE',  ( -2.922039326512111401, 227.0704416020563201, 6.682560001249291837 ) ) ;
#5462=CARTESIAN_POINT ( 'NONE',  ( 0.8561741729129458411, 184.3999999989075036, 4.933012699999999029 ) ) ;
#5472=CARTESIAN_POINT ( 'NONE',  ( 2.500000000000000444, 186.4500000000000171, 5.964466094067262247 ) ) ;
#5474=CARTESIAN_POINT ( 'NONE',  ( -1.946166655054753614, 228.1230067974157691, 6.594641503551242678 ) ) ;
#5478=CARTESIAN_POINT ( 'NONE',  ( -2.500000000000000888, 188.4500000000000171, 8.035533905932737753 ) ) ;
#5480=EDGE_CURVE ( 'NONE', #2929, #9483, #686, .T. ) ;
#5481=CARTESIAN_POINT ( 'NONE',  ( -6.403569081242510563E-16, 188.2499999989075263, 9.066987300000000971 ) ) ;
#5484=MECHANICAL_DESIGN_GEOMETRIC_PRESENTATION_REPRESENTATION('',(#7001),#2931);
#5487=CARTESIAN_POINT ( 'NONE',  ( 2.199649899629913641, 189.3965398499018136, 4.963263318916532718 ) ) ;
#5490=CARTESIAN_POINT ( 'NONE',  ( 1.785787022451674089, 228.5490719641819908, 7.825142006337427070 ) ) ;
#5495=CARTESIAN_POINT ( 'NONE',  ( 1.461580736456472795, 185.7499999989074979, 8.461580736456474128 ) ) ;
#5500=CARTESIAN_POINT ( 'NONE',  ( 1.767766952966369320, 185.7000000000000171, 5.232233047033630235 ) ) ;
#5507=CARTESIAN_POINT ( 'NONE',  ( 5.999999999999999112, 202.3202208672780102, 7.308763624231163547 ) ) ;
#5522=CARTESIAN_POINT ( 'NONE',  ( -4.438452643612533777E-16, 185.0499999989075093, 9.066987300000000971 ) ) ;
#5527=CARTESIAN_POINT ( 'NONE',  ( 1.035533905932737753, 188.9199999975965341, 4.500000000000000888 ) ) ;
#5528=CARTESIAN_POINT ( 'NONE',  ( 1.707343418157801551, 228.0835877007203294, 9.663887492166837845 ) ) ;
#5529=EDGE_CURVE ( 'NONE', #12097, #320, #14529, .T. ) ;
#5539=ORIENTED_EDGE ( 'NONE', *, *, #3553, .T. ) ;
#5548=CARTESIAN_POINT ( 'NONE',  ( 1.035533905932737975, 185.6499999978150868, 4.500000000000000888 ) ) ;
#5550=CARTESIAN_POINT ( 'NONE',  ( 0.8239120926223584274, 228.2181226988968774, 10.05946334177977519 ) ) ;
#5554=CARTESIAN_POINT ( 'NONE',  ( 2.500000000000000444, 186.3499999999999943, 8.035533905932739529 ) ) ;
#5560=DIRECTION ( 'NONE',  ( -6.123233995736766036E-17, 1.000000000000000000, 0.000000000000000000 ) ) ;
#5562=CARTESIAN_POINT ( 'NONE',  ( -1.342063929050375748, 190.0567506639880833, 4.518418250680232617 ) ) ;
#5564=ADVANCED_FACE ( 'NONE', ( #2437 ), #13258, .T. ) ;
#5566=CARTESIAN_POINT ( 'NONE',  ( 2.500000000000000444, 185.5800000002185186, 5.964466094067262247 ) ) ;
#5568=CARTESIAN_POINT ( 'NONE',  ( 1.990705347729657237, 228.2501094229765215, 6.961721135629644230 ) ) ;
#5573=CARTESIAN_POINT ( 'NONE',  ( 0.8561741729129457301, 189.0999999989075206, 9.066987299999999195 ) ) ;
#5590=VERTEX_POINT ( 'NONE', #1392 ) ;
#5596=EDGE_LOOP ( 'NONE', ( #3159, #9665, #5712 ) ) ;
#5601=CARTESIAN_POINT ( 'NONE',  ( 3.726944967918921492E-17, 185.4499999989075150, 4.933012699999999029 ) ) ;
#5604=PRODUCT_CONTEXT ( 'NONE', #8631, 'mechanical' ) ;
#5607=CARTESIAN_POINT ( 'NONE',  ( -1.958673816210946272, 228.3772695101851014, 7.328966720224260101 ) ) ;
#5614=CARTESIAN_POINT ( 'NONE',  ( 2.500000000000000000, 189.4999999978150527, 7.000000000000000000 ) ) ;
#5616=ORIENTED_EDGE ( 'NONE', *, *, #11851, .T. ) ;
#5622=CARTESIAN_POINT ( 'NONE',  ( 2.500000000000000444, 185.5999999999999943, 7.000000000000000000 ) ) ;
#5624=CARTESIAN_POINT ( 'NONE',  ( 2.500000000000000444, 185.4499999978150981, 8.035533905932739529 ) ) ;
#5626=CARTESIAN_POINT ( 'NONE',  ( -1.691178964804313178, 228.6047289695326583, 7.985882612257780622 ) ) ;
#5632=CARTESIAN_POINT ( 'NONE',  ( -6.776263578034402713E-18, 186.5999999999999943, 4.500000000000000000 ) ) ;
#5637=CARTESIAN_POINT ( 'NONE',  ( -2.727823417914460258, 189.8175560065074023, 8.604987984268861467 ) ) ;
#5639=CARTESIAN_POINT ( 'NONE',  ( 2.500000000000000444, 183.9800000002184959, 5.964466094067262247 ) ) ;
#5641=CARTESIAN_POINT ( 'NONE',  ( 1.360905158423219241, 228.7363411735375962, 8.365986164091459898 ) ) ;
#5647=CARTESIAN_POINT ( 'NONE',  ( -0.8561741729129457301, 185.2999999989075377, 4.933012699999999029 ) ) ;
#5650=EDGE_CURVE ( 'NONE', #10770, #8478, #13008, .T. ) ;
#5658=CARTESIAN_POINT ( 'NONE',  ( 2.066987300000000527, 187.4499999989075150, 7.000000000000000000 ) ) ;
#5662=CARTESIAN_POINT ( 'NONE',  ( 3.659182332138577465E-16, 189.3270225533669020, 3.938484906660876472 ) ) ;
#5677=CARTESIAN_POINT ( 'NONE',  ( -1.767766952966369320, 188.9999999978150527, 5.232233047033630235 ) ) ;
#5684=CARTESIAN_POINT ( 'NONE',  ( 0.7798766585422360897, 226.3581810736479270, 4.583957619654694504 ) ) ;
#5685=CARTESIAN_POINT ( 'NONE',  ( -0.7777163206635004933, 228.2226383035325057, 10.07273956871427956 ) ) ;
#5695=ORIENTED_EDGE ( 'NONE', *, *, #534, .F. ) ;
#5702=CARTESIAN_POINT ( 'NONE',  ( -1.767766952966369765, 188.5000000000000000, 8.767766952966368876 ) ) ;
#5704=CARTESIAN_POINT ( 'NONE',  ( -1.965306002007385144, 228.1545512627131131, 6.685743718507844768 ) ) ;
#5708=CARTESIAN_POINT ( 'NONE',  ( 0.01194215579347689300, 189.0000000000000568, 4.500000000000001776 ) ) ;
#5709=CARTESIAN_POINT ( 'NONE',  ( 1.035533905932737753, 188.1499999999999773, 4.500000000000000888 ) ) ;
#5712=ORIENTED_EDGE ( 'NONE', *, *, #8880, .F. ) ;
#5717=CARTESIAN_POINT ( 'NONE',  ( -1.974820130016563091, 226.5603787955025155, 5.179955460749784635 ) ) ;
#5719=CARTESIAN_POINT ( 'NONE',  ( 1.442725981297484195, 190.0517701937062043, 4.572028445994527956 ) ) ;
#5720=CARTESIAN_POINT ( 'NONE',  ( -2.500000000000000444, 184.2800000002184504, 5.964466094067261359 ) ) ;
#5723=CARTESIAN_POINT ( 'NONE',  ( 1.312858199469658427, 228.7505821040874139, 8.407114783769989330 ) ) ;
#5728=CARTESIAN_POINT ( 'NONE',  ( -1.461580736456473684, 185.5499999989075093, 8.461580736456474128 ) ) ;
#5731=CARTESIAN_POINT ( 'NONE',  ( 2.500000000000000444, 184.0000000000000000, 7.000000000000000000 ) ) ;
#5734=CARTESIAN_POINT ( 'NONE',  ( -1.461580736456473240, 187.7499999989075263, 5.538419263543526760 ) ) ;
#5739=CARTESIAN_POINT ( 'NONE',  ( 3.659182332138577465E-16, 188.6555110544239824, 3.692234042172417574 ) ) ;
#5741=CARTESIAN_POINT ( 'NONE',  ( 2.500000000000000000, 188.6999999978150697, 7.000000000000000000 ) ) ;
#5754=CARTESIAN_POINT ( 'NONE',  ( 2.500000000000000444, 187.8999999978150584, 7.000000000000000000 ) ) ;
#5756=CARTESIAN_POINT ( 'NONE',  ( -1.767766952966369098, 185.7999999978150356, 5.232233047033630235 ) ) ;
#5761=CARTESIAN_POINT ( 'NONE',  ( -1.035533905932737975, 189.0199999975965568, 4.500000000000000888 ) ) ;
#5762=CARTESIAN_POINT ( 'NONE',  ( 0.09803033623910094307, 226.3251703050289336, 4.486637493502143137 ) ) ;
#5764=CARTESIAN_POINT ( 'NONE',  ( -0.09789622041826565035, 228.2551366570249343, 10.16828389758070550 ) ) ;
#5780=CARTESIAN_POINT ( 'NONE',  ( -1.767766952966369542, 185.1999999978150697, 8.767766952966368876 ) ) ;
#5781=CARTESIAN_POINT ( 'NONE',  ( -1.864336199031810581, 228.4898043637318779, 7.653973795834509097 ) ) ;
#5784=VECTOR ( 'NONE', #12957, 1000.000000000000000 ) ;
#5786=CARTESIAN_POINT ( 'NONE',  ( 1.035533905932738197, 188.6499999999999773, 9.500000000000003553 ) ) ;
#5793=CARTESIAN_POINT ( 'NONE',  ( -2.961146025923796721, 227.1224618315849852, 6.835633734209157986 ) ) ;
#5795=CARTESIAN_POINT ( 'NONE',  ( -2.500000000000000444, 185.9800000002184674, 8.035533905932737753 ) ) ;
#5797=CARTESIAN_POINT ( 'NONE',  ( 1.618192118698865700, 228.6399984490590214, 8.087742880769061671 ) ) ;
#5802=CARTESIAN_POINT ( 'NONE',  ( -0.8561741729129470624, 185.5999999989075206, 9.066987300000000971 ) ) ;
#5803=CARTESIAN_POINT ( 'NONE',  ( -4.946672411965113980E-16, 184.5999999999999943, 9.500000000000001776 ) ) ;
#5805=ADVANCED_FACE ( 'NONE', ( #12838 ), #15319, .T. ) ;
#5806=ORIENTED_EDGE ( 'NONE', *, *, #9305, .T. ) ;
#5809=DIRECTION ( 'NONE',  ( -6.123233995736766036E-17, 1.000000000000000000, 0.000000000000000000 ) ) ;
#5813=CARTESIAN_POINT ( 'NONE',  ( 2.066987300000000527, 186.6499999989075320, 7.000000000000000000 ) ) ;
#5819=CARTESIAN_POINT ( 'NONE',  ( 5.999999999999999112, 229.2449477060184222, 9.834870838912449287 ) ) ;
#5823=ORIENTED_EDGE ( 'NONE', *, *, #3135, .T. ) ;
#5827=CARTESIAN_POINT ( 'NONE',  ( 3.726944967918921492E-17, 185.4499999989075150, 4.933012699999999029 ) ) ;
#5828=CARTESIAN_POINT ( 'NONE',  ( -2.500000000000000444, 184.0000000000000000, 7.000000000000000000 ) ) ;
#5833=CARTESIAN_POINT ( 'NONE',  ( 0.8561741729129452860, 187.7999999989075093, 4.933012699999999029 ) ) ;
#5839=CARTESIAN_POINT ( 'NONE',  ( 2.840695628781289894, 227.6003006331432346, 8.242276837941533429 ) ) ;
#5840=CARTESIAN_POINT ( 'NONE',  ( -1.827163138824825950, 228.0559401102076151, 9.582586618047248095 ) ) ;
#5858=CARTESIAN_POINT ( 'NONE',  ( 2.500000000000000000, 189.4999999978150527, 7.000000000000000000 ) ) ;
#5859=CARTESIAN_POINT ( 'NONE',  ( 1.498625850689462968, 228.1261123260860018, 9.788931089129667029 ) ) ;
#5873=CARTESIAN_POINT ( 'NONE',  ( -2.735089344010680268, 227.6862984522302611, 8.495314001923839342 ) ) ;
#5875=CARTESIAN_POINT ( 'NONE',  ( 2.500000000000000444, 184.7300000002184959, 7.000000000000000000 ) ) ;
#5878=CARTESIAN_POINT ( 'NONE',  ( 0.9680444063220374762, 227.6910878243089087, 5.347234874174658259 ) ) ;
#5883=CARTESIAN_POINT ( 'NONE',  ( 1.461580736456473240, 188.3499999989074922, 5.538419263543526760 ) ) ;
#5884=CARTESIAN_POINT ( 'NONE',  ( -2.066987300000001415, 185.4999999989075548, 7.856174172912944620 ) ) ;
#5890=LINE ( 'NONE', #9236, #5784 ) ;
#5891=CARTESIAN_POINT ( 'NONE',  ( -0.8561741729129457301, 186.8999999989075320, 4.933012699999999029 ) ) ;
#5897=CARTESIAN_POINT ( 'NONE',  ( 1.035533905932738419, 185.3499999978151038, 9.500000000000000000 ) ) ;
#5904=CARTESIAN_POINT ( 'NONE',  ( 0.8561741729129456191, 184.5999999989075206, 4.933012699999999029 ) ) ;
#5905=CARTESIAN_POINT ( 'NONE',  ( 1.224717432196171130, 227.7398333025587362, 5.488014595619924663 ) ) ;
#5911=CARTESIAN_POINT ( 'NONE',  ( -1.592421940838084637E-16, 188.6499999989075320, 4.933012699999999029 ) ) ;
#5918=CARTESIAN_POINT ( 'NONE',  ( 1.059913075168976260, 226.3867898013274669, 4.668296007112484602 ) ) ;
#5923=CARTESIAN_POINT ( 'NONE',  ( -2.500000000000000888, 188.2999999978150356, 7.000000000000000000 ) ) ;
#5936=CARTESIAN_POINT ( 'NONE',  ( 2.500000000000000444, 187.9499999978150697, 5.964466094067262247 ) ) ;
#5937=CARTESIAN_POINT ( 'NONE',  ( 2.349311747835623354, 227.8901172732836642, 9.094898149752092209 ) ) ;
#5941=CARTESIAN_POINT ( 'NONE',  ( -0.3590199077019145535, 189.4412677667518210, 3.993594655970155838 ) ) ;
#5945=CARTESIAN_POINT ( 'NONE',  ( -1.035533905932739751, 187.7500000000000284, 9.500000000000000000 ) ) ;
#5948=CARTESIAN_POINT ( 'NONE',  ( 1.058049511578855073, 226.3870755470184122, 4.669134239153247101 ) ) ;
#5952=CARTESIAN_POINT ( 'NONE',  ( -1.233820397871397523, 226.4104340690482218, 4.737993341516149925 ) ) ;
#5953=SURFACE_STYLE_USAGE ( .BOTH. , #15342 ) ;
#5955=CARTESIAN_POINT ( 'NONE',  ( -1.035533905932737975, 188.1800000002185129, 4.500000000000000888 ) ) ;
#5957=CARTESIAN_POINT ( 'NONE',  ( -0.6092285535620440839, 227.6401390286306992, 5.200091846327095979 ) ) ;
#5962=CARTESIAN_POINT ( 'NONE',  ( 1.461580736456472573, 188.1499999989075036, 8.461580736456474128 ) ) ;
#5964=CARTESIAN_POINT ( 'NONE',  ( -4.302927372051845722E-16, 184.8499999989074922, 9.066987300000000971 ) ) ;
#5971=CARTESIAN_POINT ( 'NONE',  ( 5.999999999999999112, 195.9172377311516016, 6.220370292208427188 ) ) ;
#5972=CARTESIAN_POINT ( 'NONE',  ( -2.066987300000001415, 187.8999999989075036, 7.856174172912944620 ) ) ;
#5986=ORIENTED_EDGE ( 'NONE', *, *, #2427, .T. ) ;
#5990=CARTESIAN_POINT ( 'NONE',  ( -6.098637220230962441E-17, 187.0499999989075093, 4.933012699999999029 ) ) ;
#5993=CARTESIAN_POINT ( 'NONE',  ( -2.500000000000000444, 185.2000000000000171, 7.000000000000000000 ) ) ;
#5996=CARTESIAN_POINT ( 'NONE',  ( -2.961755302830887615, 227.1327330595862861, 6.865988109554851171 ) ) ;
#6000=CARTESIAN_POINT ( 'NONE',  ( 2.500000000000000444, 186.2999999978150356, 7.000000000000000000 ) ) ;
#6006=CARTESIAN_POINT ( 'NONE',  ( -2.500000000000000444, 185.0999999978150754, 7.000000000000000000 ) ) ;
#6015=CARTESIAN_POINT ( 'NONE',  ( 1.035533905932737753, 188.1499999999999773, 4.500000000000001776 ) ) ;
#6018=CARTESIAN_POINT ( 'NONE',  ( 2.500000000000000444, 187.8999999978150584, 7.000000000000000000 ) ) ;
#6019=CARTESIAN_POINT ( 'NONE',  ( 2.840695628781289894, 227.6003006331432346, 8.242276837941533429 ) ) ;
#6022=CARTESIAN_POINT ( 'NONE',  ( -0.1252076328335900435, 190.0879680885402934, 4.197210855963412257 ) ) ;
#6026=CARTESIAN_POINT ( 'NONE',  ( 1.767766952966368432, 187.8999999999999773, 8.767766952966368876 ) ) ;
#6033=CARTESIAN_POINT ( 'NONE',  ( -0.1892923005757740362, 226.3252034129036474, 4.486734984831129758 ) ) ;
#6036=CARTESIAN_POINT ( 'NONE',  ( 2.500000000000000444, 188.7800000002184788, 5.964466094067262247 ) ) ;
#6037=CARTESIAN_POINT ( 'NONE',  ( -1.592074373690287370, 228.6606520933046340, 8.147391783356672690 ) ) ;
#6039=CARTESIAN_POINT ( 'NONE',  ( 1.984332343511774788, 228.2073501340537973, 6.838229870390527765 ) ) ;
#6043=CARTESIAN_POINT ( 'NONE',  ( -1.461580736456473906, 187.9499999989075150, 8.461580736456474128 ) ) ;
#6044=CARTESIAN_POINT ( 'NONE',  ( -0.8561741729129457301, 186.0999999989074922, 4.933012699999999029 ) ) ;
#6057=CARTESIAN_POINT ( 'NONE',  ( 1.304322108239046818, 189.7221164505237425, 10.09240358076341693 ) ) ;
#6074=CARTESIAN_POINT ( 'NONE',  ( -0.8561741729129467293, 185.7999999989075093, 9.066987299999999195 ) ) ;
#6079=CARTESIAN_POINT ( 'NONE',  ( -0.9647310034392982958, 228.2043607281333379, 10.01900208526334168 ) ) ;
#6091=LINE ( 'NONE', #12200, #7054 ) ;
#6099=CARTESIAN_POINT ( 'NONE',  ( -1.035533905932737975, 188.9499999978150697, 4.500000000000000888 ) ) ;
#6100=CARTESIAN_POINT ( 'NONE',  ( 2.899241599682305992, 227.5396000034540975, 8.063657412308430139 ) ) ;
#6122=CARTESIAN_POINT ( 'NONE',  ( -1.035533905932737753, 184.2500000000000000, 4.500000000000000888 ) ) ;
#6125=CARTESIAN_POINT ( 'NONE',  ( 1.078411626687468594, 228.8081072869749732, 8.573250792970148026 ) ) ;
#6128=ORIENTED_EDGE ( 'NONE', *, *, #9412, .T. ) ;
#6129=CARTESIAN_POINT ( 'NONE',  ( 2.066987300000000083, 189.0999999989075206, 6.143825827087054492 ) ) ;
#6130=CARTESIAN_POINT ( 'NONE',  ( 1.461580736456473240, 187.5499999989075093, 5.538419263543526760 ) ) ;
#6134=DIRECTION ( 'NONE',  ( -6.123233995736766036E-17, 1.000000000000000000, 0.000000000000000000 ) ) ;
#6137=CARTESIAN_POINT ( 'NONE',  ( 0.000000000000000000, 229.2449477060184222, 9.834870838912449287 ) ) ;
#6138=CARTESIAN_POINT ( 'NONE',  ( -0.05280746222630467585, 189.0001365486126303, 9.499442212161147481 ) ) ;
#6144=CARTESIAN_POINT ( 'NONE',  ( -2.500000000000000888, 187.5999999999999943, 7.000000000000000000 ) ) ;
#6153=CYLINDRICAL_SURFACE ( 'NONE', #10864, 2.500000000000000444 ) ;
#6155=CARTESIAN_POINT ( 'NONE',  ( -1.461580736456473018, 187.9499999989075150, 5.538419263543527649 ) ) ;
#6162=CARTESIAN_POINT ( 'NONE',  ( -2.998822209637060254, 227.3208645008386668, 7.419865387590665939 ) ) ;
#6166=ORIENTED_EDGE ( 'NONE', *, *, #11434, .F. ) ;
#6178=CARTESIAN_POINT ( 'NONE',  ( -2.500000000000000444, 188.3499999999999943, 5.964466094067261359 ) ) ;
#6180=CARTESIAN_POINT ( 'NONE',  ( 1.035533905932738197, 188.5499999978150356, 9.500000000000003553 ) ) ;
#6181=CARTESIAN_POINT ( 'NONE',  ( 2.692585213447247661, 226.8629897650803855, 6.071564533969844746 ) ) ;
#6183=CARTESIAN_POINT ( 'NONE',  ( -1.503949710467194167, 189.0000000002120260, 9.002347884774902553 ) ) ;
#6191=CARTESIAN_POINT ( 'NONE',  ( 0.9637716067245765128, 226.3761301684456555, 4.636858967466513270 ) ) ;
#6198=CARTESIAN_POINT ( 'NONE',  ( -1.490777987167568597E-16, 188.9300000002185129, 4.500000000000000000 ) ) ;
#6200=CARTESIAN_POINT ( 'NONE',  ( 0.2588337889006175341, 228.9066910274044346, 8.857966258178848307 ) ) ;
#6205=CARTESIAN_POINT ( 'NONE',  ( -2.066987300000000971, 186.1999999989075150, 6.143825827087054492 ) ) ;
#6208=EDGE_LOOP ( 'NONE', ( #9506, #5695 ) ) ;
#6215=CARTESIAN_POINT ( 'NONE',  ( 5.999999999999999112, 202.3202208672780102, 7.308763624231163547 ) ) ;
#6216=CARTESIAN_POINT ( 'NONE',  ( -2.108001641305449425, 189.0000000000000284, 8.365019857495370914 ) ) ;
#6221=CARTESIAN_POINT ( 'NONE',  ( -2.500000000000000444, 184.3499999999999943, 5.964466094067261359 ) ) ;
#6234=CARTESIAN_POINT ( 'NONE',  ( 2.066987299999999195, 189.1999999989075434, 7.856174172912946396 ) ) ;
#6236=( BOUNDED_CURVE ( )  B_SPLINE_CURVE ( 2, ( #7117, #15391, #10609, #2163, #4809, #10688, #2409, #7197, #6000 ),
 .UNSPECIFIED., .F., .F. ) 
 B_SPLINE_CURVE_WITH_KNOTS ( ( 3, 2, 2, 2, 3 ),
 ( 0.2142857142857142738, 0.2321428571428571508, 0.2500000000000000000, 0.2678571428571428492, 0.2857142857142856984 ),
 .UNSPECIFIED. ) 
 CURVE ( )  GEOMETRIC_REPRESENTATION_ITEM ( )  RATIONAL_B_SPLINE_CURVE ( ( 1.000000000000000000, 0.9238795325112867385, 1.000000000000000000, 0.9238795325112867385, 1.000000000000000000, 0.9238795325112867385, 1.000000000000000000, 0.9238795325112867385, 1.000000000000000000 ) ) 
 REPRESENTATION_ITEM ( '' )  );
#6241=CARTESIAN_POINT ( 'NONE',  ( -1.865818183961493126, 226.5341093703536899, 5.102530190813160615 ) ) ;
#6244=ORIENTED_EDGE ( 'NONE', *, *, #12935, .F. ) ;
#6247=CARTESIAN_POINT ( 'NONE',  ( 2.471008581483269850, 189.0000000000000284, 6.581706670152065008 ) ) ;
#6248=CIRCLE ( 'NONE', #1661, 2.500000000000000444 ) ;
#6258=CARTESIAN_POINT ( 'NONE',  ( -1.035533905932737753, 185.0199999975965284, 4.500000000000000888 ) ) ;
#6259=CARTESIAN_POINT ( 'NONE',  ( -1.159640499634989608, 227.7308148186401979, 5.461968699681960082 ) ) ;
#6260=CARTESIAN_POINT ( 'NONE',  ( 0.7798766585422360897, 226.3581810736479270, 4.583957619654694504 ) ) ;
#6261=CARTESIAN_POINT ( 'NONE',  ( -0.05280792143845292053, 189.0000000000001137, 9.499442202459045248 ) ) ;
#6267=CARTESIAN_POINT ( 'NONE',  ( 2.115286944722794438, 226.6055634003047032, 5.313108787231142216 ) ) ;
#6273=CARTESIAN_POINT ( 'NONE',  ( -2.500000000000000444, 186.6800000002185413, 5.964466094067261359 ) ) ;
#6275=CARTESIAN_POINT ( 'NONE',  ( 1.579185070784824285, 228.6572036374857078, 8.137432446265082220 ) ) ;
#6280=CARTESIAN_POINT ( 'NONE',  ( 2.500000000000000444, 185.5500000000000114, 8.035533905932739529 ) ) ;
#6282=CARTESIAN_POINT ( 'NONE',  ( -2.066987300000000527, 184.8999999989075320, 7.856174172912944620 ) ) ;
#6289=CARTESIAN_POINT ( 'NONE',  ( -1.967615029119349934, 189.0000000000000284, 5.432308397871834060 ) ) ;
#6292=FACE_OUTER_BOUND ( 'NONE', #14066, .T. ) ;
#6299=CARTESIAN_POINT ( 'NONE',  ( 2.066987299999999195, 188.3999999989075036, 7.856174172912946396 ) ) ;
#6304=ORIENTED_EDGE ( 'NONE', *, *, #13392, .F. ) ;
#6311=CARTESIAN_POINT ( 'NONE',  ( -2.103459429923432822, 227.9779199259797622, 9.353140775971661824 ) ) ;
#6319=CARTESIAN_POINT ( 'NONE',  ( -2.257704606524308488, 227.9260547655458140, 9.200601119324863575 ) ) ;
#6323=ORIENTED_EDGE ( 'NONE', *, *, #968, .T. ) ;
#6331=CARTESIAN_POINT ( 'NONE',  ( -1.767766952966369320, 187.3999999978150584, 5.232233047033630235 ) ) ;
#6332=CARTESIAN_POINT ( 'NONE',  ( -1.035533905932737753, 185.0499999999999829, 4.500000000000001776 ) ) ;
#6337=CARTESIAN_POINT ( 'NONE',  ( 2.500000000000000444, 184.8199999975965682, 5.964466094067262247 ) ) ;
#6338=CARTESIAN_POINT ( 'NONE',  ( -1.984331290054332841, 228.3135221411288285, 7.144860682478253011 ) ) ;
#6339=CARTESIAN_POINT ( 'NONE',  ( -2.599074790483714370, 227.7726799100639994, 8.749447567440038043 ) ) ;
#6340=CARTESIAN_POINT ( 'NONE',  ( -2.521737919408184148, 188.9999999974891409, 6.973570937152097748 ) ) ;
#6350=CARTESIAN_POINT ( 'NONE',  ( 2.688173913331684428, 227.7236097417891187, 8.605093950198996922 ) ) ;
#6356=CARTESIAN_POINT ( 'NONE',  ( -6.776263578034402713E-18, 186.5999999999999943, 4.500000000000000000 ) ) ;
#6358=CARTESIAN_POINT ( 'NONE',  ( 1.211961328308884367, 228.7773363860045492, 8.484382675910040916 ) ) ;
#6363=CARTESIAN_POINT ( 'NONE',  ( -2.066987300000001415, 188.5999999989074922, 6.143825827087054492 ) ) ;
#6365=CARTESIAN_POINT ( 'NONE',  ( 0.8561741729129455081, 187.7999999989075093, 4.933012699999999029 ) ) ;
#6370=SURFACE_STYLE_USAGE ( .BOTH. , #11418 ) ;
#6374=CARTESIAN_POINT ( 'NONE',  ( 1.973460340353461850, 189.7555967275478963, 9.640314175604393299 ) ) ;
#6376=CARTESIAN_POINT ( 'NONE',  ( 0.2000180313179936165, 189.6977690162252657, 10.38967773564543684 ) ) ;
#6381=CARTESIAN_POINT ( 'NONE',  ( -2.066987300000000083, 187.2499999989075263, 7.000000000000000000 ) ) ;
#6391=CARTESIAN_POINT ( 'NONE',  ( -2.866007985673219682, 189.8358165770212054, 8.236538289369191190 ) ) ;
#6392=CARTESIAN_POINT ( 'NONE',  ( -2.066760391300492827E-16, 189.4499999989075150, 4.933012699999999029 ) ) ;
#6395=CARTESIAN_POINT ( 'NONE',  ( 0.000000000000000000, 189.6977690162252657, 10.38967773564543862 ) ) ;
#6406=CARTESIAN_POINT ( 'NONE',  ( 2.491866687051035978, 189.0000000000000000, 7.260727728595771424 ) ) ;
#6410=EDGE_CURVE ( 'NONE', #12097, #4790, #1864, .T. ) ;
#6413=CARTESIAN_POINT ( 'NONE',  ( 4.743384504624081899E-17, 185.6999999978150697, 4.500000000000000000 ) ) ;
#6418=CARTESIAN_POINT ( 'NONE',  ( -2.500000000000000444, 185.9699999975965454, 7.000000000000000000 ) ) ;
#6419=CARTESIAN_POINT ( 'NONE',  ( -1.051851325171203388, 227.7069327454752283, 5.392995910236884960 ) ) ;
#6420=CARTESIAN_POINT ( 'NONE',  ( -1.707413668510289861, 226.4963546398602148, 4.991255295473766118 ) ) ;
#6421=CARTESIAN_POINT ( 'NONE',  ( -2.347932364728245513, 189.7818114793913367, 9.238878617153785555 ) ) ;
#6430=CARTESIAN_POINT ( 'NONE',  ( 2.868718875460478657, 227.0003171668635389, 6.475958485551715604 ) ) ;
#6437=CARTESIAN_POINT ( 'NONE',  ( -6.437450399132682577E-16, 187.0000000000000000, 9.500000000000001776 ) ) ;
#6439=CARTESIAN_POINT ( 'NONE',  ( 1.214181464861975757, 227.7437454098885041, 5.499312984720448938 ) ) ;
#6443=CARTESIAN_POINT ( 'NONE',  ( -2.500000000000000444, 184.3499999999999943, 5.964466094067261359 ) ) ;
#6445=CARTESIAN_POINT ( 'NONE',  ( 1.461580736456472795, 187.7499999989075263, 5.538419263543527649 ) ) ;
#6448=CARTESIAN_POINT ( 'NONE',  ( -1.767766952966369765, 186.7999999978150356, 8.767766952966368876 ) ) ;
#6454=CARTESIAN_POINT ( 'NONE',  ( 1.724409861001041877, 189.4160653832104231, 4.535432872984458186 ) ) ;
#6456=CARTESIAN_POINT ( 'NONE',  ( 1.049294306888729489, 190.0690657775611214, 4.388349470883383674 ) ) ;
#6461=CARTESIAN_POINT ( 'NONE',  ( -0.8561741729129469514, 187.3999999989075889, 9.066987299999999195 ) ) ;
#6471=CARTESIAN_POINT ( 'NONE',  ( -1.409930671981111772, 189.7264147913530223, 10.03734922520923867 ) ) ;
#6483=CARTESIAN_POINT ( 'NONE',  ( -2.500000000000000888, 187.5999999999999943, 7.000000000000000000 ) ) ;
#6490=CARTESIAN_POINT ( 'NONE',  ( 1.035533905932738197, 186.9499999978150413, 9.500000000000003553 ) ) ;
#6495=CARTESIAN_POINT ( 'NONE',  ( -2.500000000000000444, 187.5199999975965568, 5.964466094067261359 ) ) ;
#6496=CARTESIAN_POINT ( 'NONE',  ( -0.2609190394019921810, 228.9066108255455276, 8.857734630635405892 ) ) ;
#6497=CARTESIAN_POINT ( 'NONE',  ( -2.599095426179941271, 226.8075136295145171, 5.908139701444540925 ) ) ;
#6499=CARTESIAN_POINT ( 'NONE',  ( -2.568556045599829751, 189.1887412497518142, 8.730119828325975107 ) ) ;
#6507=CARTESIAN_POINT ( 'NONE',  ( 2.777531521503771472, 227.6543197073591216, 8.401223264750537822 ) ) ;
#6512=CARTESIAN_POINT ( 'NONE',  ( -1.524659305057740610E-16, 189.0000000000000000, 4.500000000000000000 ) ) ;
#6513=CARTESIAN_POINT ( 'NONE',  ( 1.035533905932738197, 186.2500000000000000, 9.500000000000003553 ) ) ;
#6515=CARTESIAN_POINT ( 'NONE',  ( 0.2606415164794526063, 227.6142277459897230, 5.125258584176975774 ) ) ;
#6519=CARTESIAN_POINT ( 'NONE',  ( -2.500000000000000444, 184.4000000000000057, 7.000000000000000000 ) ) ;
#6521=CARTESIAN_POINT ( 'NONE',  ( 2.066987299999999639, 189.2999999989075661, 6.143825827087054492 ) ) ;
#6526=CARTESIAN_POINT ( 'NONE',  ( 2.136295798034152149, 189.1395851565150679, 9.290070378363166625 ) ) ;
#6528=AXIS2_PLACEMENT_3D ( 'NONE', #13498, #4111, #2921 ) ;
#6534=CARTESIAN_POINT ( 'NONE',  ( -0.8561741729129456191, 187.8999999989075320, 4.933012699999999029 ) ) ;
#6541=B_SPLINE_CURVE_WITH_KNOTS ( 'NONE', 3,
 ( #12508, #12431, #1606, #9900, #1374, #2496, #12195, #11317, #340, #416, #106, #4077, #8948, #2731, #12352, #1531, #7355, #6406, #11163, #11238, #6247, #4973, #14753, #9824, #3761, #1446, #5124, #9977, #14828, #3913, #8789, #13619 ),
 .UNSPECIFIED., .F., .F.,
 ( 4, 2, 2, 2, 2, 2, 2, 2, 2, 2, 2, 2, 2, 2, 2, 4 ),
 ( 0.2688658829390630500, 0.3001158843412741750, 0.3313658857434852445, 0.3626158871456963695, 0.3938658885479074945, 0.4251158899501185640, 0.4563658913523296889, 0.4876158927545407584, 0.5188658941567521055, 0.5501158955589633415, 0.5813658969611745775, 0.6126158983633858135, 0.6438658997655970495, 0.7063659025700197436, 0.7376159039722309796, 0.7688659053744424376 ),
 .UNSPECIFIED. ) ;
#6566=CARTESIAN_POINT ( 'NONE',  ( 1.767766952966368654, 185.3999999978150584, 8.767766952966368876 ) ) ;
#6567=CARTESIAN_POINT ( 'NONE',  ( 1.767766952966369320, 184.7999999978150356, 5.232233047033630235 ) ) ;
#6570=CARTESIAN_POINT ( 'NONE',  ( -1.035533905932737975, 187.4199999975965909, 4.500000000000000888 ) ) ;
#6571=CARTESIAN_POINT ( 'NONE',  ( 1.455795469679321608, 228.1339131991090596, 9.811868761735363265 ) ) ;
#6572=CARTESIAN_POINT ( 'NONE',  ( -2.951760543192366804, 227.4626507460308744, 7.837199003427246069 ) ) ;
#6574=VERTEX_POINT ( 'NONE', #12123 ) ;
#6587=CARTESIAN_POINT ( 'NONE',  ( 1.035533905932738419, 184.6500000000000057, 9.500000000000003553 ) ) ;
#6589=CARTESIAN_POINT ( 'NONE',  ( 0.9680444063220374762, 227.6910878243089087, 5.347234874174658259 ) ) ;
#6594=CARTESIAN_POINT ( 'NONE',  ( 9.147955830346443662E-17, 185.0000000000000000, 4.500000000000000000 ) ) ;
#6596=CARTESIAN_POINT ( 'NONE',  ( -1.461580736456473018, 187.9499999989075150, 5.538419263543527649 ) ) ;
#6600=CARTESIAN_POINT ( 'NONE',  ( 2.500000000000000444, 187.0999999978150754, 7.000000000000000000 ) ) ;
#6601=CARTESIAN_POINT ( 'NONE',  ( -5.999999999999999112, 186.5669965222008670, 9.317226423031115701 ) ) ;
#6604=CARTESIAN_POINT ( 'NONE',  ( 2.975469271411296024, 189.2669713358625643, 7.607624869344640217 ) ) ;
#6614=CARTESIAN_POINT ( 'NONE',  ( 2.066987299999999639, 186.7999999989074809, 7.856174172912946396 ) ) ;
#6644=CARTESIAN_POINT ( 'NONE',  ( 1.035533905932737753, 187.2499999978151095, 4.500000000000000888 ) ) ;
#6645=CARTESIAN_POINT ( 'NONE',  ( -1.767766952966369098, 184.9999999978150527, 5.232233047033630235 ) ) ;
#6648=CARTESIAN_POINT ( 'NONE',  ( -2.500000000000000888, 188.3699999975965511, 7.000000000000000000 ) ) ;
#6649=CARTESIAN_POINT ( 'NONE',  ( -1.580502612156455822, 228.6570661798589299, 8.137035460797768849 ) ) ;
#6650=CARTESIAN_POINT ( 'NONE',  ( -2.692660167145737304, 226.8630334657495666, 6.071693271619351684 ) ) ;
#6658=CARTESIAN_POINT ( 'NONE',  ( -0.8561741729129456191, 184.4999999989074979, 4.933012699999999029 ) ) ;
#6660=CARTESIAN_POINT ( 'NONE',  ( 2.763116275831466240, 226.9137948392856572, 6.221213813064390585 ) ) ;
#6667=CARTESIAN_POINT ( 'NONE',  ( 2.500000000000000444, 186.3499999999999943, 8.035533905932739529 ) ) ;
#6668=CARTESIAN_POINT ( 'NONE',  ( -1.923034433439944513, 228.0917019039344495, 6.504231185664401949 ) ) ;
#6672=CARTESIAN_POINT ( 'NONE',  ( -1.767766952966369320, 186.7000000000000171, 5.232233047033630235 ) ) ;
#6674=CARTESIAN_POINT ( 'NONE',  ( 0.8561741729129458411, 188.2999999989075093, 9.066987299999999195 ) ) ;
#6680=CARTESIAN_POINT ( 'NONE',  ( 0.000000000000000000, 0.000000000000000000, 0.000000000000000000 ) ) ;
#6681=CARTESIAN_POINT ( 'NONE',  ( 2.879399905582539887, 189.9211542764968215, 6.401088131731365927 ) ) ;
#6683=CARTESIAN_POINT ( 'NONE',  ( 0.4515139163396761357, 228.8949857255690290, 8.824160678851793449 ) ) ;
#6688=CARTESIAN_POINT ( 'NONE',  ( -0.8561741729129456191, 188.6999999989075150, 4.933012699999999029 ) ) ;
#6691=ADVANCED_FACE ( 'NONE', ( #2895 ), #10594, .T. ) ;
#6708=CARTESIAN_POINT ( 'NONE',  ( 2.500000000000000444, 186.2999999978150356, 7.000000000000000000 ) ) ;
#6720=CARTESIAN_POINT ( 'NONE',  ( -1.965116437629976787E-16, 189.6999999978150697, 4.500000000000000000 ) ) ;
#6725=CARTESIAN_POINT ( 'NONE',  ( 2.500000000000000000, 189.5199999975965852, 8.035533905932739529 ) ) ;
#6726=CARTESIAN_POINT ( 'NONE',  ( -2.913793338554793166E-15, 228.9118723800512782, 8.872930300147347182 ) ) ;
#6732=EDGE_LOOP ( 'NONE', ( #179, #14826, #3835, #963, #2308, #8288, #414, #13066, #8943, #5806, #1992, #3404, #3627, #4173, #12582, #11063 ) ) ;
#6744=CARTESIAN_POINT ( 'NONE',  ( -1.035533905932739751, 188.5500000000000114, 9.500000000000003553 ) ) ;
#6746=CARTESIAN_POINT ( 'NONE',  ( 1.080575604060385553, 227.7131986584202821, 5.411092224208442936 ) ) ;
#6750=CARTESIAN_POINT ( 'NONE',  ( -1.035533905932737975, 187.4499999999999886, 4.500000000000000888 ) ) ;
#6758=CARTESIAN_POINT ( 'NONE',  ( -1.050085366295366640, 189.7133272379261086, 10.20285018932750631 ) ) ;
#6763=CARTESIAN_POINT ( 'NONE',  ( 1.691241850060078322, 228.6046986201012601, 7.985794961368397615 ) ) ;
#6768=CARTESIAN_POINT ( 'NONE',  ( 2.066987300000000971, 185.0999999989074922, 6.143825827087054492 ) ) ;
#6776=CARTESIAN_POINT ( 'NONE',  ( -0.8561741729129469514, 184.7999999989075093, 9.066987300000000971 ) ) ;
#6787=ORIENTED_EDGE ( 'NONE', *, *, #5650, .F. ) ;
#6789=ORIENTED_EDGE ( 'NONE', *, *, #15525, .F. ) ;
#6797=CARTESIAN_POINT ( 'NONE',  ( 0.8561741729129455081, 185.3999999989075604, 4.933012699999999029 ) ) ;
#6803=CARTESIAN_POINT ( 'NONE',  ( -2.500000000000000888, 188.4199999975965625, 8.035533905932737753 ) ) ;
#6804=CARTESIAN_POINT ( 'NONE',  ( -1.312946155259101522, 228.7505583286450985, 8.407046118935697976 ) ) ;
#6822=CARTESIAN_POINT ( 'NONE',  ( 2.500000000000000000, 187.9500000000000455, 8.035533905932739529 ) ) ;
#6824=CARTESIAN_POINT ( 'NONE',  ( -1.619108980504621043, 228.6400225536183655, 8.087812496111112637 ) ) ;
#6829=CARTESIAN_POINT ( 'NONE',  ( -1.767766952966369320, 187.5000000000000000, 5.232233047033630235 ) ) ;
#6837=CARTESIAN_POINT ( 'NONE',  ( -2.500000000000000444, 186.7999999999999829, 7.000000000000000000 ) ) ;
#6838=CARTESIAN_POINT ( 'NONE',  ( -2.085029866008053734, 227.9837044594366375, 9.370153471119524013 ) ) ;
#6841=CARTESIAN_POINT ( 'NONE',  ( -1.939157702522992466, 228.0901138467679914, 6.499644785989321605 ) ) ;
#6842=CARTESIAN_POINT ( 'NONE',  ( 1.637003574519428017, 228.6312591184326948, 8.062503195461440342 ) ) ;
#6848=EDGE_LOOP ( 'NONE', ( #6323, #8209, #8615, #9688, #13071 ) ) ;
#6849=CARTESIAN_POINT ( 'NONE',  ( -2.066987300000000527, 188.8499999989074922, 7.000000000000000000 ) ) ;
#6850=CARTESIAN_POINT ( 'NONE',  ( 2.500000000000000444, 184.7999999999999829, 7.000000000000000000 ) ) ;
#6860=CARTESIAN_POINT ( 'NONE',  ( 0.000000000000000000, 229.2449477060184222, 9.834870838912449287 ) ) ;
#6869=CARTESIAN_POINT ( 'NONE',  ( 3.659182332138577465E-16, 220.7266909453316543, 6.312321839438380877 ) ) ;
#6877=CARTESIAN_POINT ( 'NONE',  ( -2.500000000000000888, 189.1499999978150868, 8.035533905932737753 ) ) ;
#6883=CARTESIAN_POINT ( 'NONE',  ( 2.734462269239809729, 226.8914732116195125, 6.155466831691636109 ) ) ;
#6887=EDGE_LOOP ( 'NONE', ( #6166, #7198, #10988, #6787, #8708 ) ) ;
#6902=CARTESIAN_POINT ( 'NONE',  ( -1.035533905932737753, 185.7499999978150527, 4.500000000000000888 ) ) ;
#6903=CARTESIAN_POINT ( 'NONE',  ( -1.052533753945321227, 228.8137749680355455, 8.589619379135912780 ) ) ;
#6907=CARTESIAN_POINT ( 'NONE',  ( 1.767766952966369320, 185.7000000000000171, 5.232233047033630235 ) ) ;
#6908=CARTESIAN_POINT ( 'NONE',  ( -2.500000000000000444, 187.4499999978150981, 5.964466094067261359 ) ) ;
#6915=CARTESIAN_POINT ( 'NONE',  ( -1.815463298294986760, 226.5191110010208035, 5.058303205087121945 ) ) ;
#6917=CARTESIAN_POINT ( 'NONE',  ( -5.421010862427522170E-16, 185.3300000002185186, 9.500000000000001776 ) ) ;
#6919=CARTESIAN_POINT ( 'NONE',  ( 1.939628903789791359, 228.4085481513286311, 7.419301219863100982 ) ) ;
#6926=CARTESIAN_POINT ( 'NONE',  ( 1.461580736456472795, 189.3499999989074922, 5.538419263543527649 ) ) ;
#6929=CARTESIAN_POINT ( 'NONE',  ( -1.035533905932739751, 186.1500000000000057, 9.500000000000000000 ) ) ;
#6934=CARTESIAN_POINT ( 'NONE',  ( 1.461580736456473240, 187.5499999989075093, 5.538419263543526760 ) ) ;
#6937=LINE ( 'NONE', #14229, #9612 ) ;
#6938=CARTESIAN_POINT ( 'NONE',  ( -1.768235190473915752, 189.0000319710720191, 5.232701284541176001 ) ) ;
#6942=AXIS2_PLACEMENT_3D ( 'NONE', #1301, #116, #4981 ) ;
#6946=CARTESIAN_POINT ( 'NONE',  ( -0.8561741729129455081, 185.4999999989075263, 4.933012699999999029 ) ) ;
#6952=CARTESIAN_POINT ( 'NONE',  ( -2.066987300000000083, 184.8499999989075206, 7.000000000000000000 ) ) ;
#6958=CARTESIAN_POINT ( 'NONE',  ( 1.586671692599169736, 226.4708623422775418, 4.916117818249839289 ) ) ;
#6968=DIRECTION ( 'NONE',  ( -1.000000000000000000, 0.000000000000000000, 0.000000000000000000 ) ) ;
#6975=CARTESIAN_POINT ( 'NONE',  ( -2.500000000000000444, 185.1499999978150584, 8.035533905932737753 ) ) ;
#6977=CARTESIAN_POINT ( 'NONE',  ( -1.958673816210946272, 228.3772695101851014, 7.328966720224260101 ) ) ;
#6982=CARTESIAN_POINT ( 'NONE',  ( -1.623479154671611857, 188.9999999998642295, 5.090171998070187165 ) ) ;
#6983=CARTESIAN_POINT ( 'NONE',  ( -1.035533905932739751, 188.5500000000000114, 9.500000000000003553 ) ) ;
#6990=CARTESIAN_POINT ( 'NONE',  ( -2.998365736231170420, 227.3239176724307811, 7.428857950662880683 ) ) ;
#6991=CARTESIAN_POINT ( 'NONE',  ( 1.543908090016931078, 189.4216793162960357, 4.413729295337608605 ) ) ;
#6992=CARTESIAN_POINT ( 'NONE',  ( 4.743384504624081899E-17, 185.7300000002184959, 4.500000000000000000 ) ) ;
#6995=CARTESIAN_POINT ( 'NONE',  ( 1.314367061980813878, 227.7707019980692564, 5.577165148888615143 ) ) ;
#7000=CARTESIAN_POINT ( 'NONE',  ( 0.8561741729129458411, 184.3999999989075036, 4.933012699999999029 ) ) ;
#7001=STYLED_ITEM ( 'NONE', ( #832 ), #10455 ) ;
#7002=ORIENTED_EDGE ( 'NONE', *, *, #923, .T. ) ;
#7006=CARTESIAN_POINT ( 'NONE',  ( -2.066987300000000971, 187.8499999989074922, 7.000000000000000000 ) ) ;
#7011=CARTESIAN_POINT ( 'NONE',  ( -5.999999999999999112, 194.5935680195190116, 12.11154058223188379 ) ) ;
#7015=CARTESIAN_POINT ( 'NONE',  ( 2.500000000000000444, 184.0000000000000000, 7.000000000000000000 ) ) ;
#7028=CARTESIAN_POINT ( 'NONE',  ( -2.066987300000000971, 184.8999999989075320, 7.856174172912944620 ) ) ;
#7033=CARTESIAN_POINT ( 'NONE',  ( 2.975657739721877970, 227.4162173224905530, 7.700537803285528504 ) ) ;
#7051=CARTESIAN_POINT ( 'NONE',  ( 1.035533905932738197, 188.6499999999999773, 9.500000000000003553 ) ) ;
#7052=CARTESIAN_POINT ( 'NONE',  ( -0.4531526159469659309, 228.8951261137066524, 8.824566127799945647 ) ) ;
#7054=VECTOR ( 'NONE', #14596, 1000.000000000000000 ) ;
#7060=EDGE_LOOP ( 'NONE', ( #13678, #11045, #12505, #12269, #2349, #13673, #9191, #8601, #625, #2143, #3623, #6244, #5436, #10825, #14156 ) ) ;
#7067=CARTESIAN_POINT ( 'NONE',  ( -2.228027794420240681, 226.6433447131122989, 5.424436590844790018 ) ) ;
#7070=CARTESIAN_POINT ( 'NONE',  ( -1.739661649193494419, 228.5884852582535700, 7.938969847602396435 ) ) ;
#7071=CARTESIAN_POINT ( 'NONE',  ( -1.974809306405319154, 228.1756194782155944, 6.746589926531873616 ) ) ;
#7078=CARTESIAN_POINT ( 'NONE',  ( 3.659182332138073087E-16, 190.0875178197511275, 4.201689379953569947 ) ) ;
#7083=CARTESIAN_POINT ( 'NONE',  ( 2.066987300000000083, 184.4499999989075150, 7.000000000000000000 ) ) ;
#7085=CARTESIAN_POINT ( 'NONE',  ( -2.066987300000000527, 186.1999999989075150, 6.143825827087054492 ) ) ;
#7090=CARTESIAN_POINT ( 'NONE',  ( 0.000000000000000000, 194.5935680195190116, 12.11154058223188201 ) ) ;
#7095=ORIENTED_EDGE ( 'NONE', *, *, #8766, .F. ) ;
#7098=CARTESIAN_POINT ( 'NONE',  ( -1.461580736456473240, 184.9499999989075150, 8.461580736456472351 ) ) ;
#7100=ORIENTED_EDGE ( 'NONE', *, *, #9159, .T. ) ;
#7105=CARTESIAN_POINT ( 'NONE',  ( 2.066987300000000083, 186.8999999989075036, 6.143825827087054492 ) ) ;
#7111=CARTESIAN_POINT ( 'NONE',  ( 1.035533905932737753, 188.9499999999999886, 4.500000000000000888 ) ) ;
#7113=CARTESIAN_POINT ( 'NONE',  ( 2.999966428792078865, 227.3061007205240571, 7.376404775963534277 ) ) ;
#7117=CARTESIAN_POINT ( 'NONE',  ( -2.500000000000000444, 185.8999999978150584, 7.000000000000000000 ) ) ;
#7122=CARTESIAN_POINT ( 'NONE',  ( -1.767766952966369542, 185.2999999999999829, 8.767766952966368876 ) ) ;
#7125=UNCERTAINTY_MEASURE_WITH_UNIT (LENGTH_MEASURE( 1.000000000000000082E-05 ), #9372, 'distance_accuracy_value', 'NONE');
#7129=CARTESIAN_POINT ( 'NONE',  ( 2.500000000000000444, 187.8999999978150584, 7.000000000000000000 ) ) ;
#7133=CARTESIAN_POINT ( 'NONE',  ( -1.965116437629976787E-16, 189.6999999978150697, 4.500000000000000000 ) ) ;
#7134=CARTESIAN_POINT ( 'NONE',  ( 2.856278104602718138, 227.5851434513726019, 8.197675965640897289 ) ) ;
#7137=CARTESIAN_POINT ( 'NONE',  ( -1.999225930651338912, 189.0000000014894113, 5.488052162623582753 ) ) ;
#7144=CARTESIAN_POINT ( 'NONE',  ( 2.530388970177701147, 226.7703937237002663, 5.798752065564563907 ) ) ;
#7145=ORIENTED_EDGE ( 'NONE', *, *, #14457, .F. ) ;
#7148=CARTESIAN_POINT ( 'NONE',  ( -1.359954704877545772, 226.4297670701539005, 4.794973935041616286 ) ) ;
#7150=CARTESIAN_POINT ( 'NONE',  ( 2.500000000000000000, 187.9300000002185129, 7.000000000000000000 ) ) ;
#7151=CARTESIAN_POINT ( 'NONE',  ( -0.2624983655900470780, 228.9118722929915748, 8.872930048714067652 ) ) ;
#7152=CARTESIAN_POINT ( 'NONE',  ( 0.7033144145436343031, 227.6506181221223244, 5.230356066017792571 ) ) ;
#7153=CARTESIAN_POINT ( 'NONE',  ( 2.500000000000000444, 184.6999999978150697, 7.000000000000000000 ) ) ;
#7155=DIRECTION ( 'NONE',  ( -1.000000000000000000, 0.000000000000000000, 0.000000000000000000 ) ) ;
#7156=EDGE_LOOP ( 'NONE', ( #13755, #5539, #454, #9821, #10586 ) ) ;
#7158=CARTESIAN_POINT ( 'NONE',  ( 0.8561741729129455081, 189.1999999989075434, 4.933012699999999029 ) ) ;
#7160=CARTESIAN_POINT ( 'NONE',  ( 2.066987300000000527, 186.6499999989075320, 7.000000000000000000 ) ) ;
#7166=CARTESIAN_POINT ( 'NONE',  ( 5.999999999999999112, 185.8606548077538321, 9.048340948986950849 ) ) ;
#7167=CARTESIAN_POINT ( 'NONE',  ( -6.268043809681822509E-16, 188.0499999989075093, 9.066987300000000971 ) ) ;
#7187=CARTESIAN_POINT ( 'NONE',  ( 2.066987299999999639, 185.9999999989074979, 7.856174172912946396 ) ) ;
#7192=DIRECTION ( 'NONE',  ( -1.000000000000000000, 0.000000000000000000, 0.000000000000000000 ) ) ;
#7193=CARTESIAN_POINT ( 'NONE',  ( 2.900052503084635358, 227.0405808247315917, 6.594625917879634258 ) ) ;
#7197=CARTESIAN_POINT ( 'NONE',  ( 2.500000000000000444, 186.2499999978150527, 8.035533905932739529 ) ) ;
#7198=ORIENTED_EDGE ( 'NONE', *, *, #14464, .F. ) ;
#7212=CARTESIAN_POINT ( 'NONE',  ( 1.767766952966368432, 187.7999999978150356, 8.767766952966368876 ) ) ;
#7214=CARTESIAN_POINT ( 'NONE',  ( 1.328920255623610380, 226.4243263863947391, 4.778947530392284371 ) ) ;
#7217=CARTESIAN_POINT ( 'NONE',  ( -0.7894119942751186558, 189.4371793396122996, 4.080690743408665000 ) ) ;
#7222=CARTESIAN_POINT ( 'NONE',  ( -2.500000000000000888, 187.5999999999999943, 7.000000000000000000 ) ) ;
#7223=ORIENTED_EDGE ( 'NONE', *, *, #8957, .F. ) ;
#7228=CARTESIAN_POINT ( 'NONE',  ( -0.3835139150651865059, 226.3309889762633134, 4.503752476338783062 ) ) ;
#7229=CARTESIAN_POINT ( 'NONE',  ( 0.000000000000000000, 184.0000000000000000, 7.000000000000000000 ) ) ;
#7230=CARTESIAN_POINT ( 'NONE',  ( 1.035533905932737753, 187.2800000002184788, 4.500000000000000888 ) ) ;
#7232=CARTESIAN_POINT ( 'NONE',  ( -1.497718339830098611, 227.8307599607422844, 5.750615970570851943 ) ) ;
#7233=CARTESIAN_POINT ( 'NONE',  ( 1.939628903789791359, 228.4085481513286311, 7.419301219863100982 ) ) ;
#7237=CARTESIAN_POINT ( 'NONE',  ( -0.8561741729129457301, 186.8999999989075036, 4.933012699999999029 ) ) ;
#7238=CARTESIAN_POINT ( 'NONE',  ( 1.461580736456473240, 186.7499999989075263, 5.538419263543526760 ) ) ;
#7239=CARTESIAN_POINT ( 'NONE',  ( -1.524659305057740610E-16, 189.0000000000000000, 4.500000000000000000 ) ) ;
#7246=CARTESIAN_POINT ( 'NONE',  ( 1.461580736456473240, 189.1499999989075036, 5.538419263543526760 ) ) ;
#7248=CARTESIAN_POINT ( 'NONE',  ( 0.9292488878324430823, 189.7097868069985509, 10.24626543057368799 ) ) ;
#7250=CARTESIAN_POINT ( 'NONE',  ( -2.500000000000000444, 184.4000000000000057, 7.000000000000000000 ) ) ;
#7253=CARTESIAN_POINT ( 'NONE',  ( 1.767766952966369098, 187.2999999999999829, 5.232233047033630235 ) ) ;
#7259=CARTESIAN_POINT ( 'NONE',  ( 1.499313473695500498, 228.6911157451824579, 8.235372547512890051 ) ) ;
#7264=CARTESIAN_POINT ( 'NONE',  ( 1.461580736456472795, 187.7499999989075263, 5.538419263543527649 ) ) ;
#7272=CARTESIAN_POINT ( 'NONE',  ( -1.057007967372188606, 228.1937333886401120, 9.987756413537558942 ) ) ;
#7276=CARTESIAN_POINT ( 'NONE',  ( 1.035533905932738197, 188.5499999978150356, 9.500000000000000000 ) ) ;
#7290=CARTESIAN_POINT ( 'NONE',  ( 2.500000000000000444, 188.0500000000000114, 5.964466094067262247 ) ) ;
#7292=CARTESIAN_POINT ( 'NONE',  ( 2.500000000000000444, 187.0999999978150754, 7.000000000000000000 ) ) ;
#7293=CARTESIAN_POINT ( 'NONE',  ( 0.9678947859540896204, 226.3761757439112898, 4.637006245081842337 ) ) ;
#7308=CARTESIAN_POINT ( 'NONE',  ( 1.035533905932737975, 184.1500000000000341, 4.500000000000000888 ) ) ;
#7310=CARTESIAN_POINT ( 'NONE',  ( 1.989829716803914739, 228.2822890550965553, 7.054657748597916722 ) ) ;
#7315=CARTESIAN_POINT ( 'NONE',  ( -0.8561741729129472844, 188.7999999989075093, 9.066987300000000971 ) ) ;
#7316=CARTESIAN_POINT ( 'NONE',  ( 0.8561741729129457301, 185.1999999989075150, 4.933012699999999029 ) ) ;
#7318=CARTESIAN_POINT ( 'NONE',  ( 1.237586355860756271, 228.7707919832083689, 8.465482067366952634 ) ) ;
#7323=CARTESIAN_POINT ( 'NONE',  ( 0.000000000000000000, 194.5935680195190116, 12.11154058223188201 ) ) ;
#7324=CARTESIAN_POINT ( 'NONE',  ( -2.513578226966119988, 189.0000000000000568, 6.945885617963185155 ) ) ;
#7328=CARTESIAN_POINT ( 'NONE',  ( -1.035533905932737753, 184.2500000000000000, 4.500000000000001776 ) ) ;
#7341=CARTESIAN_POINT ( 'NONE',  ( -1.461580736456473462, 188.1499999989075320, 8.461580736456472351 ) ) ;
#7347=CARTESIAN_POINT ( 'NONE',  ( -2.599095426179941271, 226.8075136295145171, 5.908139701444540925 ) ) ;
#7355=CARTESIAN_POINT ( 'NONE',  ( 2.435767893059086031, 189.0000000000000284, 7.586867366306830007 ) ) ;
#7365=CARTESIAN_POINT ( 'NONE',  ( -9.825582188149883933E-17, 188.0999999978150754, 4.500000000000000000 ) ) ;
#7366=CARTESIAN_POINT ( 'NONE',  ( 2.189302528786933877, 227.9503441805575505, 9.272039875547573473 ) ) ;
#7369=CARTESIAN_POINT ( 'NONE',  ( -2.110350344527927469, 189.0000000007702852, 8.349190812944474516 ) ) ;
#7382=CARTESIAN_POINT ( 'NONE',  ( -2.500000000000000444, 184.4000000000000057, 7.000000000000000000 ) ) ;
#7384=CARTESIAN_POINT ( 'NONE',  ( 1.786693786749917301, 227.9723819745098865, 6.159628423921897244 ) ) ;
#7388=CARTESIAN_POINT ( 'NONE',  ( -0.8561741729129458411, 188.4999999989074979, 4.933012699999999029 ) ) ;
#7389=CARTESIAN_POINT ( 'NONE',  ( -1.461580736456473906, 187.1499999989075320, 8.461580736456474128 ) ) ;
#7391=CARTESIAN_POINT ( 'NONE',  ( -1.461580736456473240, 185.7499999989074979, 8.461580736456472351 ) ) ;
#7398=CARTESIAN_POINT ( 'NONE',  ( -2.504122110289527026, 189.0000000000000568, 7.207938535869628183 ) ) ;
#7408=ORIENTED_EDGE ( 'NONE', *, *, #8973, .F. ) ;
#7416=DIRECTION ( 'NONE',  ( -6.123233995736766036E-17, 1.000000000000000000, 0.000000000000000000 ) ) ;
#7418=CARTESIAN_POINT ( 'NONE',  ( -4.946672411965113980E-16, 185.8499999989075206, 9.066987300000000971 ) ) ;
#7424=CARTESIAN_POINT ( 'NONE',  ( -2.899241975612990352, 227.5395701600909888, 8.063569561630318461 ) ) ;
#7440=CARTESIAN_POINT ( 'NONE',  ( -2.500000000000000444, 186.6999999978150697, 7.000000000000000000 ) ) ;
#7441=CARTESIAN_POINT ( 'NONE',  ( 2.255245247391631569, 227.9269692368775395, 9.203290779546277278 ) ) ;
#7442=CARTESIAN_POINT ( 'NONE',  ( -0.1937970382946692660, 188.9999999996763904, 9.496463395928850915 ) ) ;
#7444=VERTEX_POINT ( 'NONE', #10993 ) ;
#7449=CARTESIAN_POINT ( 'NONE',  ( 2.085888082922780828, 226.5962934794760031, 5.285790551658203995 ) ) ;
#7455=CARTESIAN_POINT ( 'NONE',  ( -5.082197683525802034E-17, 187.3300000002185186, 4.500000000000000000 ) ) ;
#7458=B_SPLINE_CURVE_WITH_KNOTS ( 'NONE', 1,
 ( #4100, #13800 ),
 .UNSPECIFIED., .F., .F.,
 ( 2, 2 ),
 ( 0.000000000000000000, 1.000000000000000000 ),
 .UNSPECIFIED. ) ;
#7459=CARTESIAN_POINT ( 'NONE',  ( 1.132923824227977772, 228.7961917368426157, 8.538838004569329954 ) ) ;
#7465=CARTESIAN_POINT ( 'NONE',  ( 1.461580736456473462, 185.9499999989075150, 5.538419263543526760 ) ) ;
#7467=CARTESIAN_POINT ( 'NONE',  ( 0.8561741729129460632, 185.8999999989075320, 9.066987299999999195 ) ) ;
#7470=DIRECTION ( 'NONE',  ( 0.9996022823964011428, 0.0003845365441984911130, 0.02819803467534520366 ) ) ;
#7473=CARTESIAN_POINT ( 'NONE',  ( 0.000000000000000000, 185.8606548077538321, 9.048340948986950849 ) ) ;
#7474=EDGE_CURVE ( 'NONE', #13467, #15176, #13199, .T. ) ;
#7475=CARTESIAN_POINT ( 'NONE',  ( -0.4796817918372051071, 189.0000000000000000, 9.463196806509678538 ) ) ;
#7484=CARTESIAN_POINT ( 'NONE',  ( -1.461580736456473018, 187.9499999989075150, 5.538419263543527649 ) ) ;
#7490=DIRECTION ( 'NONE',  ( -1.000000000000000000, 0.000000000000000000, 0.000000000000000000 ) ) ;
#7491=CARTESIAN_POINT ( 'NONE',  ( -1.488442273571260133, 228.1302346159642696, 9.801076297958973171 ) ) ;
#7499=EDGE_CURVE ( 'NONE', #8478, #8762, #14148, .T. ) ;
#7501=CARTESIAN_POINT ( 'NONE',  ( -2.733336431741188566, 227.6877042401139022, 8.499448515046434949 ) ) ;
#7504=VERTEX_POINT ( 'NONE', #10352 ) ;
#7505=VERTEX_POINT ( 'NONE', #10561 ) ;
#7512=CARTESIAN_POINT ( 'NONE',  ( -1.035533905932739751, 187.6499999978150584, 9.500000000000003553 ) ) ;
#7516=CARTESIAN_POINT ( 'NONE',  ( -5.421010862427522170E-17, 187.3699999975965511, 4.500000000000000000 ) ) ;
#7517=CARTESIAN_POINT ( 'NONE',  ( -1.946166655054753614, 228.1230067974157691, 6.594641503551242678 ) ) ;
#7518=CARTESIAN_POINT ( 'NONE',  ( -1.826734563482391938, 226.5243062390148623, 5.073637952221710101 ) ) ;
#7520=CARTESIAN_POINT ( 'NONE',  ( -2.461562117910376823, 189.0000000012555859, 7.467094330940653002 ) ) ;
#7526=CARTESIAN_POINT ( 'NONE',  ( 2.999777127831125600, 227.3703607088935712, 7.565575523838102612 ) ) ;
#7531=CARTESIAN_POINT ( 'NONE',  ( 2.500000000000000444, 188.8500000000000227, 5.964466094067262247 ) ) ;
#7532=CARTESIAN_POINT ( 'NONE',  ( -5.454892180317694184E-16, 185.4000000000000057, 9.500000000000001776 ) ) ;
#7534=CARTESIAN_POINT ( 'NONE',  ( 0.5467140873060455375, 228.8869147685435053, 8.800851294624202126 ) ) ;
#7537=VECTOR ( 'NONE', #5338, 1000.000000000000000 ) ;
#7539=CARTESIAN_POINT ( 'NONE',  ( 0.8561741729129460632, 188.0999999989074922, 9.066987300000000971 ) ) ;
#7541=CARTESIAN_POINT ( 'NONE',  ( 1.461580736456472351, 186.7499999989075263, 8.461580736456474128 ) ) ;
#7550=CARTESIAN_POINT ( 'NONE',  ( 0.7305957235815243589, 189.7049259502624921, 10.30464020416732573 ) ) ;
#7551=DIRECTION ( 'NONE',  ( -1.000000000000000000, 0.000000000000000000, 0.000000000000000000 ) ) ;
#7557=CARTESIAN_POINT ( 'NONE',  ( -2.066987300000000971, 185.6999999989075434, 7.856174172912944620 ) ) ;
#7577=CARTESIAN_POINT ( 'NONE',  ( -1.502165409303774624, 228.1258990818537598, 9.788304365642131799 ) ) ;
#7590=CARTESIAN_POINT ( 'NONE',  ( 1.767766952966369320, 186.3999999978150584, 5.232233047033630235 ) ) ;
#7595=CARTESIAN_POINT ( 'NONE',  ( 1.767766952966369320, 186.4699999975965454, 5.232233047033630235 ) ) ;
#7596=CARTESIAN_POINT ( 'NONE',  ( -1.990689658724532629, 228.2709309767465697, 7.021854970500988280 ) ) ;
#7597=CARTESIAN_POINT ( 'NONE',  ( -2.994031302066835654, 227.3524127508109132, 7.512731884239616242 ) ) ;
#7598=CARTESIAN_POINT ( 'NONE',  ( -2.686130926226363513, 189.9500051332105670, 5.898299179268767567 ) ) ;
#7602=( GEOMETRIC_REPRESENTATION_CONTEXT ( 3 ) GLOBAL_UNCERTAINTY_ASSIGNED_CONTEXT ( ( #7125 ) ) GLOBAL_UNIT_ASSIGNED_CONTEXT ( ( #9372, #1011, #4439 ) ) REPRESENTATION_CONTEXT ( 'NONE', 'WORKASPACE' ) );
#7613=CARTESIAN_POINT ( 'NONE',  ( -1.767766952966369765, 186.9000000000000057, 8.767766952966368876 ) ) ;
#7616=CARTESIAN_POINT ( 'NONE',  ( -1.618809023786734747, 227.8806835185142461, 5.894798052868548410 ) ) ;
#7621=CARTESIAN_POINT ( 'NONE',  ( -1.461580736456473240, 187.7499999989075263, 5.538419263543526760 ) ) ;
#7623=CARTESIAN_POINT ( 'NONE',  ( -1.592421940838084637E-16, 188.6499999989075320, 4.933012699999999029 ) ) ;
#7628=CARTESIAN_POINT ( 'NONE',  ( -1.035533905932739751, 186.8499999978150754, 9.500000000000000000 ) ) ;
#7629=CARTESIAN_POINT ( 'NONE',  ( -5.999999999999999112, 187.9952603975225429, 3.440894205938198613 ) ) ;
#7631=CARTESIAN_POINT ( 'NONE',  ( 2.079732661467729837, 189.0000000025126781, 5.600772965815071558 ) ) ;
#7632=CARTESIAN_POINT ( 'NONE',  ( -1.767766952966369320, 188.1999999978150697, 5.232233047033630235 ) ) ;
#7633=CARTESIAN_POINT ( 'NONE',  ( 1.992407597290263954, 189.7567858285134719, 9.623042625840206199 ) ) ;
#7636=CARTESIAN_POINT ( 'NONE',  ( -1.524659305057740610E-16, 189.0000000000000000, 4.500000000000000000 ) ) ;
#7638=CARTESIAN_POINT ( 'NONE',  ( -2.066987300000000083, 186.3999999989075320, 6.143825827087054492 ) ) ;
#7646=CARTESIAN_POINT ( 'NONE',  ( 3.659182332138073087E-16, 190.0875178197511275, 4.201689379953569947 ) ) ;
#7657=ORIENTED_EDGE ( 'NONE', *, *, #14425, .F. ) ;
#7667=CARTESIAN_POINT ( 'NONE',  ( 1.767766952966369320, 184.7999999978150356, 5.232233047033630235 ) ) ;
#7673=CARTESIAN_POINT ( 'NONE',  ( -2.500000000000000444, 185.1699999975965625, 7.000000000000000000 ) ) ;
#7674=CARTESIAN_POINT ( 'NONE',  ( -1.498122667687309173, 228.6899413643594983, 8.231980868713440813 ) ) ;
#7675=CARTESIAN_POINT ( 'NONE',  ( -1.058356156152139738, 226.3870070917984094, 4.668936284651906909 ) ) ;
#7676=CARTESIAN_POINT ( 'NONE',  ( -1.074555296234348978, 189.7140709984146270, 10.19372410532584894 ) ) ;
#7683=CARTESIAN_POINT ( 'NONE',  ( 2.717538370304318551, 226.8807925037416453, 6.123999117906609335 ) ) ;
#7689=CARTESIAN_POINT ( 'NONE',  ( -1.035533905932737753, 185.0499999999999829, 4.500000000000000888 ) ) ;
#7691=CARTESIAN_POINT ( 'NONE',  ( 1.161994134746590523, 227.7310455073454136, 5.462634941821782775 ) ) ;
#7697=CARTESIAN_POINT ( 'NONE',  ( 1.461580736456472573, 188.9499999989075150, 8.461580736456474128 ) ) ;
#7699=CARTESIAN_POINT ( 'NONE',  ( 1.461580736456472351, 189.1499999989075320, 8.461580736456474128 ) ) ;
#7704=CARTESIAN_POINT ( 'NONE',  ( -5.999999999999999112, 215.0542865858234336, 7.296348638347391891 ) ) ;
#7705=CARTESIAN_POINT ( 'NONE',  ( 1.753917781081038241, 189.0000000001399485, 8.787807861841729462 ) ) ;
#7712=CARTESIAN_POINT ( 'NONE',  ( 2.066987300000000083, 187.6999999989075150, 6.143825827087054492 ) ) ;
#7745=CARTESIAN_POINT ( 'NONE',  ( 9.825582188149883933E-17, 184.8999999978150584, 4.500000000000000000 ) ) ;
#7746=CARTESIAN_POINT ( 'NONE',  ( -2.500000000000000444, 185.0999999978150754, 7.000000000000000000 ) ) ;
#7749=CARTESIAN_POINT ( 'NONE',  ( 1.767766952966368432, 187.8699999975965511, 8.767766952966368876 ) ) ;
#7750=CARTESIAN_POINT ( 'NONE',  ( 1.826454486347603767, 228.0556294925947896, 9.581672574142119814 ) ) ;
#7751=CARTESIAN_POINT ( 'NONE',  ( -2.961755302830887615, 227.1327330595862861, 6.865988109554851171 ) ) ;
#7753=ADVANCED_FACE ( 'NONE', ( #4263 ), #1944, .T. ) ;
#7763=AXIS2_PLACEMENT_3D ( 'NONE', #9841, #10870, #14357 ) ;
#7769=CARTESIAN_POINT ( 'NONE',  ( -2.500000000000000444, 187.5500000000000114, 5.964466094067261359 ) ) ;
#7770=CARTESIAN_POINT ( 'NONE',  ( -1.497718339830098611, 227.8307599607422844, 5.750615970570851943 ) ) ;
#7775=CARTESIAN_POINT ( 'NONE',  ( 1.035533905932737975, 184.9499999999999886, 4.500000000000000888 ) ) ;
#7777=CARTESIAN_POINT ( 'NONE',  ( 0.8561741729129458411, 187.4999999989075263, 9.066987299999999195 ) ) ;
#7780=CARTESIAN_POINT ( 'NONE',  ( -2.499999999999998224, 186.7499999978150811, 8.035533905932741305 ) ) ;
#7782=CARTESIAN_POINT ( 'NONE',  ( 3.659182332138577465E-16, 188.6555110544239824, 3.692234042172417574 ) ) ;
#7784=CARTESIAN_POINT ( 'NONE',  ( 1.414552616161247167, 189.0000000003665832, 9.066428890920718686 ) ) ;
#7787=CARTESIAN_POINT ( 'NONE',  ( 1.899761157012515467, 190.0238153260214062, 4.888075663000788218 ) ) ;
#7792=CARTESIAN_POINT ( 'NONE',  ( 1.461580736456472573, 185.9499999989075150, 8.461580736456474128 ) ) ;
#7809=CARTESIAN_POINT ( 'NONE',  ( 1.035533905932737975, 186.4499999978150697, 4.500000000000001776 ) ) ;
#7823=CARTESIAN_POINT ( 'NONE',  ( 1.035533905932738419, 186.1499999978150584, 9.500000000000003553 ) ) ;
#7827=CARTESIAN_POINT ( 'NONE',  ( -6.403569081242510563E-16, 186.9699999975965454, 9.500000000000001776 ) ) ;
#7828=CARTESIAN_POINT ( 'NONE',  ( -0.4531526159469659309, 228.8951261137066524, 8.824566127799945647 ) ) ;
#7829=CARTESIAN_POINT ( 'NONE',  ( -2.381852405317018029, 227.8773184320497478, 9.057252860304588538 ) ) ;
#7831=EDGE_CURVE ( 'NONE', #13744, #15449, #9484, .T. ) ;
#7837=CARTESIAN_POINT ( 'NONE',  ( 2.500000000000000444, 189.5499999978150356, 5.964466094067262247 ) ) ;
#7841=CARTESIAN_POINT ( 'NONE',  ( 2.767106495899620988, 226.9168529135898780, 6.230221390918345037 ) ) ;
#7847=CARTESIAN_POINT ( 'NONE',  ( -1.035533905932739751, 188.5499999999999829, 9.500000000000000000 ) ) ;
#7849=( BOUNDED_CURVE ( )  B_SPLINE_CURVE ( 2, ( #8369, #2383, #15602, #4703, #14393, #7328, #14480, #6221, #7250 ),
 .UNSPECIFIED., .F., .F. ) 
 B_SPLINE_CURVE_WITH_KNOTS ( ( 3, 2, 2, 2, 3 ),
 ( 0.000000000000000000, 0.01785714285714285615, 0.03571428571428571230, 0.05357142857142856845, 0.07142857142857142461 ),
 .UNSPECIFIED. ) 
 CURVE ( )  GEOMETRIC_REPRESENTATION_ITEM ( )  RATIONAL_B_SPLINE_CURVE ( ( 1.000000000000000000, 0.9238795325112867385, 1.000000000000000000, 0.9238795325112867385, 1.000000000000000000, 0.9238795325112867385, 1.000000000000000000, 0.9238795325112867385, 1.000000000000000000 ) ) 
 REPRESENTATION_ITEM ( '' )  );
#7850=CARTESIAN_POINT ( 'NONE',  ( -1.035533905932739529, 184.5499999999999829, 9.500000000000003553 ) ) ;
#7852=CARTESIAN_POINT ( 'NONE',  ( -1.361823383409473953, 227.7851450847494448, 5.618877607002349173 ) ) ;
#7860=CARTESIAN_POINT ( 'NONE',  ( 2.066987299999999639, 188.9999999989074979, 7.856174172912946396 ) ) ;
#7863=CARTESIAN_POINT ( 'NONE',  ( -0.8561741729129469514, 188.1999999989075150, 9.066987299999999195 ) ) ;
#7868=CARTESIAN_POINT ( 'NONE',  ( 1.705890586619502214, 189.1032960091229143, 9.654523998859355416 ) ) ;
#7871=CARTESIAN_POINT ( 'NONE',  ( 1.558909820229182230, 228.6656996696739554, 8.161969471806774123 ) ) ;
#7876=CARTESIAN_POINT ( 'NONE',  ( 2.066987300000000971, 184.2999999989074809, 6.143825827087054492 ) ) ;
#7880=DIRECTION ( 'NONE',  ( -6.123233995736766036E-17, 1.000000000000000000, 0.000000000000000000 ) ) ;
#7901=CARTESIAN_POINT ( 'NONE',  ( 1.767766952966369098, 188.7999999978150356, 5.232233047033630235 ) ) ;
#7905=CARTESIAN_POINT ( 'NONE',  ( -7.894347068410079160E-16, 189.3699999975965511, 9.500000000000001776 ) ) ;
#7906=CARTESIAN_POINT ( 'NONE',  ( -1.770887355114397321, 228.5581793045761287, 7.851444524843710582 ) ) ;
#7907=CARTESIAN_POINT ( 'NONE',  ( -1.502165409303774624, 228.1258990818537598, 9.788304365642131799 ) ) ;
#7913=FACE_OUTER_BOUND ( 'NONE', #6732, .T. ) ;
#7918=FILL_AREA_STYLE_COLOUR ( '', #8016 ) ;
#7922=CARTESIAN_POINT ( 'NONE',  ( 1.767766952966369098, 188.0999999999999943, 5.232233047033630235 ) ) ;
#7923=CARTESIAN_POINT ( 'NONE',  ( -0.8818726034074957365, 227.6760006002180319, 5.303662110480990677 ) ) ;
#7928=CARTESIAN_POINT ( 'NONE',  ( -2.500000000000000444, 187.5500000000000114, 5.964466094067261359 ) ) ;
#7938=CARTESIAN_POINT ( 'NONE',  ( -2.315215587853216128, 189.7792518546661142, 9.280090613206597894 ) ) ;
#7941=CARTESIAN_POINT ( 'NONE',  ( 2.051099020578225574, 189.4035295303465034, 4.809436146376961929 ) ) ;
#7942=CARTESIAN_POINT ( 'NONE',  ( -2.500000000000000444, 185.0800000002185186, 5.964466094067261359 ) ) ;
#7943=CARTESIAN_POINT ( 'NONE',  ( -0.9972535833697410146, 227.6950091073211979, 5.358559763169368217 ) ) ;
#7944=CARTESIAN_POINT ( 'NONE',  ( 1.940097806574041073, 228.1129668193434838, 6.565645474235799917 ) ) ;
#7946=DIRECTION ( 'NONE',  ( -6.123233995736766036E-17, 1.000000000000000000, 0.000000000000000000 ) ) ;
#7949=CARTESIAN_POINT ( 'NONE',  ( 0.8561741729129451750, 189.3999999989075604, 4.933012699999999029 ) ) ;
#7955=DIRECTION ( 'NONE',  ( -1.000000000000000000, 0.000000000000000000, 0.000000000000000000 ) ) ;
#7960=CARTESIAN_POINT ( 'NONE',  ( 9.825582188149883933E-17, 184.4499999989075150, 4.933012699999999029 ) ) ;
#7964=CARTESIAN_POINT ( 'NONE',  ( 3.659182332138577465E-16, 202.3202208672780102, 7.308763624242801349 ) ) ;
#7973=VERTEX_POINT ( 'NONE', #5622 ) ;
#7979=CARTESIAN_POINT ( 'NONE',  ( 1.767766952966368432, 189.3999999978150584, 8.767766952966368876 ) ) ;
#7981=CARTESIAN_POINT ( 'NONE',  ( 1.035533905932737975, 184.8499999978150754, 4.500000000000001776 ) ) ;
#7985=CARTESIAN_POINT ( 'NONE',  ( -1.767766952966369765, 189.2699999975965568, 8.767766952966368876 ) ) ;
#7986=CARTESIAN_POINT ( 'NONE',  ( -1.977913707823687250, 228.3348771801055364, 7.206535253053350409 ) ) ;
#7988=CARTESIAN_POINT ( 'NONE',  ( -1.057007967372188606, 228.1937333886401120, 9.987756413537558942 ) ) ;
#7993=CARTESIAN_POINT ( 'NONE',  ( -7.826584432629735133E-16, 189.2999999978150356, 9.500000000000001776 ) ) ;
#7998=( LENGTH_UNIT ( ) NAMED_UNIT ( * ) SI_UNIT ( .MILLI., .METRE. ) );
#8003=CARTESIAN_POINT ( 'NONE',  ( -6.911788849595090767E-16, 187.7999999999999829, 9.500000000000001776 ) ) ;
#8005=CARTESIAN_POINT ( 'NONE',  ( -0.2609190394019921810, 228.9066108255455276, 8.857734630635405892 ) ) ;
#8011=CARTESIAN_POINT ( 'NONE',  ( 1.035533905932737753, 187.3499999999999659, 4.500000000000000888 ) ) ;
#8016=COLOUR_RGB ( '', 0.72549020, 0.75294118, 0.79215686) ;
#8019=CARTESIAN_POINT ( 'NONE',  ( -1.933502023194013875, 228.0279153893430077, 9.500182718874965460 ) ) ;
#8022=CARTESIAN_POINT ( 'NONE',  ( -2.500000000000000444, 185.1300000002185016, 7.000000000000000000 ) ) ;
#8023=CARTESIAN_POINT ( 'NONE',  ( -1.316422468852913585, 227.7699220668886539, 5.574912663155255466 ) ) ;
#8024=CARTESIAN_POINT ( 'NONE',  ( 0.8212144138252523984, 228.8542370555972809, 8.706476195820313180 ) ) ;
#8029=CARTESIAN_POINT ( 'NONE',  ( -2.066987300000001415, 184.6999999989075150, 7.856174172912944620 ) ) ;
#8044=FACE_OUTER_BOUND ( 'NONE', #11642, .T. ) ;
#8053=CARTESIAN_POINT ( 'NONE',  ( 3.659182332138577465E-16, 214.7097693073062032, 7.296684523004520528 ) ) ;
#8054=ORIENTED_EDGE ( 'NONE', *, *, #8359, .T. ) ;
#8060=CARTESIAN_POINT ( 'NONE',  ( 1.461580736456473018, 184.5499999989075093, 5.538419263543527649 ) ) ;
#8063=CARTESIAN_POINT ( 'NONE',  ( -2.500000000000000444, 185.8999999978150584, 7.000000000000000000 ) ) ;
#8064=CARTESIAN_POINT ( 'NONE',  ( 2.500000000000000444, 188.8499999999999659, 5.964466094067262247 ) ) ;
#8065=CARTESIAN_POINT ( 'NONE',  ( 2.500000000000000000, 188.7199999975965738, 8.035533905932739529 ) ) ;
#8066=CARTESIAN_POINT ( 'NONE',  ( 2.441738273555474681, 226.7282248110694809, 5.674544857840881029 ) ) ;
#8071=EDGE_CURVE ( 'NONE', #25, #15176, #11000, .T. ) ;
#8079=EDGE_CURVE ( 'NONE', #5268, #13744, #1316, .T. ) ;
#8087=CARTESIAN_POINT ( 'NONE',  ( 4.743384504624081899E-17, 185.6999999978150697, 4.500000000000000000 ) ) ;
#8088=AXIS2_PLACEMENT_3D ( 'NONE', #4863, #3653, #7551 ) ;
#8090=CARTESIAN_POINT ( 'NONE',  ( -1.989902382949138460, 228.2815652486739282, 7.052567354366601649 ) ) ;
#8095=CARTESIAN_POINT ( 'NONE',  ( 2.500000000000000000, 188.0000000000000000, 7.000000000000000000 ) ) ;
#8096=DIRECTION ( 'NONE',  ( -6.123233995736766036E-17, 1.000000000000000000, 0.000000000000000000 ) ) ;
#8102=CARTESIAN_POINT ( 'NONE',  ( -2.866366203691001147, 227.0037563968904237, 6.486100089110839129 ) ) ;
#8103=SURFACE_STYLE_FILL_AREA ( #15656 ) ;
#8104=CARTESIAN_POINT ( 'NONE',  ( 1.294034140306127068, 188.9999999982559586, 4.853059374542415760 ) ) ;
#8106=CARTESIAN_POINT ( 'NONE',  ( -1.990742470614812465, 228.3030780210874866, 7.114697468104904665 ) ) ;
#8107=CARTESIAN_POINT ( 'NONE',  ( 1.924362066950147332, 228.0923243445923276, 6.506028829785237555 ) ) ;
#8114=CARTESIAN_POINT ( 'NONE',  ( -1.461580736456473684, 184.7499999989074979, 8.461580736456474128 ) ) ;
#8118=CARTESIAN_POINT ( 'NONE',  ( 2.066987300000000083, 185.2499999989074979, 7.000000000000000000 ) ) ;
#8120=CARTESIAN_POINT ( 'NONE',  ( -4.811147140404425926E-16, 185.6499999989075320, 9.066987300000000971 ) ) ;
#8124=CARTESIAN_POINT ( 'NONE',  ( 0.000000000000000000, 215.7452399395091049, 13.29567785264566027 ) ) ;
#8125=CARTESIAN_POINT ( 'NONE',  ( -1.035533905932737975, 188.9499999978150129, 4.500000000000001776 ) ) ;
#8127=CARTESIAN_POINT ( 'NONE',  ( -0.07717340183324797320, 189.6978550888158281, 10.38866401756451552 ) ) ;
#8136=ADVANCED_FACE ( 'NONE', ( #12205 ), #11015, .T. ) ;
#8141=CARTESIAN_POINT ( 'NONE',  ( 1.767766952966369098, 189.5999999978150470, 5.232233047033630235 ) ) ;
#8144=DIRECTION ( 'NONE',  ( 0.8660254037844503650, -0.4999999999999796829, -0.000000000000000000 ) ) ;
#8148=CARTESIAN_POINT ( 'NONE',  ( 0.9678947859540896204, 226.3761757439112898, 4.637006245081842337 ) ) ;
#8151=ORIENTED_EDGE ( 'NONE', *, *, #5529, .F. ) ;
#8164=CARTESIAN_POINT ( 'NONE',  ( -0.001074311305641557088, 226.3251817249170017, 4.486671161788877704 ) ) ;
#8165=CARTESIAN_POINT ( 'NONE',  ( 1.035533905932738419, 186.1499999978150584, 9.500000000000003553 ) ) ;
#8167=CARTESIAN_POINT ( 'NONE',  ( -0.3256308520141213414, 228.9034500205340237, 8.848606045481535176 ) ) ;
#8171=CARTESIAN_POINT ( 'NONE',  ( 2.500000000000000444, 186.4000000000000057, 7.000000000000000000 ) ) ;
#8181=CARTESIAN_POINT ( 'NONE',  ( -2.770343633091874036, 227.6599362732561644, 8.417748511065344275 ) ) ;
#8183=CARTESIAN_POINT ( 'NONE',  ( 2.500000000000000444, 186.4000000000000057, 7.000000000000000000 ) ) ;
#8184=CARTESIAN_POINT ( 'NONE',  ( 1.035533905932738419, 185.3800000002184731, 9.500000000000003553 ) ) ;
#8186=CARTESIAN_POINT ( 'NONE',  ( 1.886647494277889692, 228.0514830721454871, 6.388076905524764371 ) ) ;
#8193=CARTESIAN_POINT ( 'NONE',  ( 1.461580736456472351, 189.1499999989075320, 8.461580736456474128 ) ) ;
#8199=CARTESIAN_POINT ( 'NONE',  ( 0.8561741729129455081, 185.3999999989075604, 4.933012699999999029 ) ) ;
#8201=CARTESIAN_POINT ( 'NONE',  ( 2.066987300000000083, 187.3999999989075320, 7.856174172912946396 ) ) ;
#8205=CARTESIAN_POINT ( 'NONE',  ( -5.999999999999999112, 201.6409668649147022, 13.30942870683726120 ) ) ;
#8209=ORIENTED_EDGE ( 'NONE', *, *, #5529, .T. ) ;
#8211=ORIENTED_EDGE ( 'NONE', *, *, #10754, .T. ) ;
#8213=CARTESIAN_POINT ( 'NONE',  ( 2.066987300000000083, 184.4999999989074979, 6.143825827087054492 ) ) ;
#8215=ORIENTED_EDGE ( 'NONE', *, *, #14278, .T. ) ;
#8219=CARTESIAN_POINT ( 'NONE',  ( -1.035533905932737975, 188.1499999978150868, 4.500000000000000888 ) ) ;
#8222=ADVANCED_BREP_SHAPE_REPRESENTATION ( '', ( #10455, #14201 ), #4310 ) ;
#8227=CARTESIAN_POINT ( 'NONE',  ( 1.829800800964088481, 226.5245823332902546, 5.074452397578279594 ) ) ;
#8246=CARTESIAN_POINT ( 'NONE',  ( -1.035533905932739751, 187.7500000000000284, 9.500000000000003553 ) ) ;
#8247=CARTESIAN_POINT ( 'NONE',  ( -1.160340649284625325, 228.7901875120212196, 8.521497460825987247 ) ) ;
#8258=CARTESIAN_POINT ( 'NONE',  ( 1.767766952966369098, 186.5000000000000000, 5.232233047033630235 ) ) ;
#8259=CARTESIAN_POINT ( 'NONE',  ( -2.687528980000447820, 226.8550369918930869, 6.048145777815692625 ) ) ;
#8262=CARTESIAN_POINT ( 'NONE',  ( 2.500000000000000444, 184.7800000002184788, 5.964466094067262247 ) ) ;
#8264=CARTESIAN_POINT ( 'NONE',  ( -1.212146835196386663, 227.7435586823976337, 5.498773705076675178 ) ) ;
#8270=CARTESIAN_POINT ( 'NONE',  ( 2.066987300000000083, 188.2999999989075093, 6.143825827087054492 ) ) ;
#8280=CARTESIAN_POINT ( 'NONE',  ( 2.066987300000000083, 185.7999999989075093, 7.856174172912946396 ) ) ;
#8284=CARTESIAN_POINT ( 'NONE',  ( 0.000000000000000000, 185.8606548077538321, 9.048340948986950849 ) ) ;
#8286=CARTESIAN_POINT ( 'NONE',  ( -1.035533905932739529, 185.2499999978150811, 9.500000000000000000 ) ) ;
#8288=ORIENTED_EDGE ( 'NONE', *, *, #4957, .T. ) ;
#8292=DIRECTION ( 'NONE',  ( -6.123233995736766036E-17, 1.000000000000000000, 0.000000000000000000 ) ) ;
#8298=CARTESIAN_POINT ( 'NONE',  ( -2.066987300000001415, 188.0999999989074922, 7.856174172912944620 ) ) ;
#8303=CARTESIAN_POINT ( 'NONE',  ( 2.383228694455616914, 226.7027912316577556, 5.599607710487992662 ) ) ;
#8324=CARTESIAN_POINT ( 'NONE',  ( 1.035533905932737753, 189.6499999978150868, 4.500000000000000888 ) ) ;
#8325=CARTESIAN_POINT ( 'NONE',  ( -0.1300625424525254092, 228.9108363453237303, 8.869938172763147222 ) ) ;
#8341=CARTESIAN_POINT ( 'NONE',  ( -2.126963226675738117, 226.6093206107916274, 5.324180815053653149 ) ) ;
#8343=CARTESIAN_POINT ( 'NONE',  ( 1.074754184052031381, 190.0681451684283729, 4.397840615916859264 ) ) ;
#8344=CARTESIAN_POINT ( 'NONE',  ( -1.767766952966369765, 187.6300000002185016, 8.767766952966368876 ) ) ;
#8347=CARTESIAN_POINT ( 'NONE',  ( 1.161994134746590523, 227.7310455073454136, 5.462634941821782775 ) ) ;
#8353=CARTESIAN_POINT ( 'NONE',  ( -0.8561741729129458411, 187.6999999989075150, 4.933012699999999029 ) ) ;
#8355=CARTESIAN_POINT ( 'NONE',  ( -2.066987300000001415, 186.2999999989075093, 7.856174172912944620 ) ) ;
#8358=CARTESIAN_POINT ( 'NONE',  ( -2.500000000000000444, 186.0000000000000000, 7.000000000000000000 ) ) ;
#8359=EDGE_CURVE ( 'NONE', #5418, #2406, #2951, .T. ) ;
#8363=CARTESIAN_POINT ( 'NONE',  ( 0.8561741729129460632, 187.2999999989075661, 9.066987300000000971 ) ) ;
#8369=CARTESIAN_POINT ( 'NONE',  ( 2.500000000000000444, 184.0000000000000000, 7.000000000000000000 ) ) ;
#8377=CARTESIAN_POINT ( 'NONE',  ( 0.2602597315884058182, 228.9118724663684645, 8.872930549436382819 ) ) ;
#8379=EDGE_CURVE ( 'NONE', #12014, #3363, #4719, .T. ) ;
#8383=CARTESIAN_POINT ( 'NONE',  ( 2.066987300000000083, 187.6999999989075150, 6.143825827087054492 ) ) ;
#8391=CARTESIAN_POINT ( 'NONE',  ( 1.240393925004889208, 226.4108590421392933, 4.739248726333301853 ) ) ;
#8411=CARTESIAN_POINT ( 'NONE',  ( -1.767766952966369765, 186.7999999978150356, 8.767766952966368876 ) ) ;
#8412=CARTESIAN_POINT ( 'NONE',  ( 0.6359992007181909379, 226.3469529472061765, 4.550856198837272437 ) ) ;
#8416=CARTESIAN_POINT ( 'NONE',  ( -1.016439536705160407E-17, 228.2551366889529731, 10.16828399152529272 ) ) ;
#8424=CARTESIAN_POINT ( 'NONE',  ( -1.172763158762331281, 226.4018383945252992, 4.712657049679232379 ) ) ;
#8426=CARTESIAN_POINT ( 'NONE',  ( 2.500000000000000444, 186.2800000002184788, 8.035533905932739529 ) ) ;
#8428=CARTESIAN_POINT ( 'NONE',  ( -0.7328022267957914337, 227.6546247107034446, 5.241927322362504249 ) ) ;
#8429=CARTESIAN_POINT ( 'NONE',  ( -2.913793338554793166E-15, 228.9118723800512782, 8.872930300147347182 ) ) ;
#8434=CARTESIAN_POINT ( 'NONE',  ( 2.066987299999999639, 188.1999999989075150, 7.856174172912946396 ) ) ;
#8436=CARTESIAN_POINT ( 'NONE',  ( -2.066987300000001415, 184.6999999989075150, 7.856174172912944620 ) ) ;
#8444=CARTESIAN_POINT ( 'NONE',  ( -2.066987300000000971, 185.4999999989075263, 7.856174172912944620 ) ) ;
#8465=CARTESIAN_POINT ( 'NONE',  ( 1.461580736456473018, 186.1499999989075320, 5.538419263543527649 ) ) ;
#8467=( BOUNDED_CURVE ( )  B_SPLINE_CURVE ( 2, ( #3051, #423, #6567, #7981, #9182, #1772, #6645, #9258, #7746 ),
 .UNSPECIFIED., .F., .F. ) 
 B_SPLINE_CURVE_WITH_KNOTS ( ( 3, 2, 2, 2, 3 ),
 ( 0.000000000000000000, 0.01785714285714285268, 0.03571428571428570536, 0.05357142857142856152, 0.07142857142857141073 ),
 .UNSPECIFIED. ) 
 CURVE ( )  GEOMETRIC_REPRESENTATION_ITEM ( )  RATIONAL_B_SPLINE_CURVE ( ( 1.000000000000000000, 0.9238795325112867385, 1.000000000000000000, 0.9238795325112867385, 1.000000000000000000, 0.9238795325112867385, 1.000000000000000000, 0.9238795325112868495, 0.9999999999999998890 ) ) 
 REPRESENTATION_ITEM ( '' )  );
#8475=CARTESIAN_POINT ( 'NONE',  ( -2.052299789776659722, 226.5858468330626465, 5.255005641065958244 ) ) ;
#8478=VERTEX_POINT ( 'NONE', #9738 ) ;
#8481=( BOUNDED_CURVE ( )  B_SPLINE_CURVE ( 3, ( #2933, #9292, #9145, #9449 ),
 .UNSPECIFIED., .F., .F. ) 
 B_SPLINE_CURVE_WITH_KNOTS ( ( 4, 4 ),
 ( 0.5000000000000000000, 0.5000594734819727716 ),
 .UNSPECIFIED. ) 
 CURVE ( )  GEOMETRIC_REPRESENTATION_ITEM ( )  RATIONAL_B_SPLINE_CURVE ( ( 0.9996420244238370945, 0.9997613282504840271, 0.9998806534425321857, 0.9999999999999814593 ) ) 
 REPRESENTATION_ITEM ( '' )  );
#8492=CARTESIAN_POINT ( 'NONE',  ( 2.500000000000000444, 184.0000000000000000, 7.000000000000000000 ) ) ;
#8495=CARTESIAN_POINT ( 'NONE',  ( 1.767766952966369098, 188.7999999978150356, 5.232233047033630235 ) ) ;
#8496=CARTESIAN_POINT ( 'NONE',  ( 1.628454131612142364, 226.4793820939146372, 4.941229787183066158 ) ) ;
#8498=CARTESIAN_POINT ( 'NONE',  ( 0.08612929575471790777, 189.4418673012125680, 3.980892606666732281 ) ) ;
#8511=CARTESIAN_POINT ( 'NONE',  ( 2.500000000000000444, 184.0000000000000000, 7.000000000000000000 ) ) ;
#8512=CARTESIAN_POINT ( 'NONE',  ( 1.984153134209927671, 228.3142122347729526, 7.146853712282291049 ) ) ;
#8515=B_SPLINE_CURVE_WITH_KNOTS ( 'NONE', 3,
 ( #6395, #11228, #5191, #11927, #10509, #12962 ),
 .UNSPECIFIED., .F., .F.,
 ( 4, 2, 4 ),
 ( 0.09236347834653250988, 0.5261283886372931651, 0.9760345799090694996 ),
 .UNSPECIFIED. ) ;
#8517=CARTESIAN_POINT ( 'NONE',  ( 2.066987300000000083, 189.0499999989075093, 7.000000000000000000 ) ) ;
#8518=CARTESIAN_POINT ( 'NONE',  ( 0.8561741729129461742, 185.6999999989075434, 9.066987300000000971 ) ) ;
#8527=CARTESIAN_POINT ( 'NONE',  ( -2.066987300000000971, 188.5999999989074922, 6.143825827087054492 ) ) ;
#8534=CARTESIAN_POINT ( 'NONE',  ( 2.500000000000000444, 187.2000000000000171, 7.000000000000000000 ) ) ;
#8547=CARTESIAN_POINT ( 'NONE',  ( -2.066987300000000971, 187.9999999989075263, 6.143825827087054492 ) ) ;
#8555=CARTESIAN_POINT ( 'NONE',  ( -2.087773716237738331, 226.5967140655768048, 5.287030890998575927 ) ) ;
#8570=CARTESIAN_POINT ( 'NONE',  ( 1.767766952966369098, 188.0999999999999943, 5.232233047033630235 ) ) ;
#8572=CARTESIAN_POINT ( 'NONE',  ( -6.844026213814746740E-16, 187.6999999978150697, 9.500000000000001776 ) ) ;
#8573=CARTESIAN_POINT ( 'NONE',  ( 2.998835045281009304, 227.2583357984985639, 7.235791215503737384 ) ) ;
#8576=CARTESIAN_POINT ( 'NONE',  ( -1.726536558038261449, 188.9999999997880877, 8.813927586020868787 ) ) ;
#8583=CARTESIAN_POINT ( 'NONE',  ( 1.034563906089895458, 226.3842683607827553, 4.660856843270724248 ) ) ;
#8588=CARTESIAN_POINT ( 'NONE',  ( -1.035533905932739751, 187.6800000002184845, 9.500000000000003553 ) ) ;
#8591=CARTESIAN_POINT ( 'NONE',  ( 1.864425960470169619, 228.0311117417621745, 6.329243341474429130 ) ) ;
#8596=CARTESIAN_POINT ( 'NONE',  ( -0.8561741729129471734, 187.1999999989075434, 9.066987300000000971 ) ) ;
#8597=CARTESIAN_POINT ( 'NONE',  ( 2.066987300000000971, 185.0999999989074922, 6.143825827087054492 ) ) ;
#8600=CARTESIAN_POINT ( 'NONE',  ( -2.066987300000000527, 185.6999999989075150, 7.856174172912944620 ) ) ;
#8601=ORIENTED_EDGE ( 'NONE', *, *, #10094, .F. ) ;
#8605=CARTESIAN_POINT ( 'NONE',  ( 0.000000000000000000, 201.6409668649146738, 13.30942870683726298 ) ) ;
#8606=CARTESIAN_POINT ( 'NONE',  ( 2.066987299999999639, 188.9999999989075263, 7.856174172912946396 ) ) ;
#8608=CARTESIAN_POINT ( 'NONE',  ( 0.6765616680526839177, 189.0525113742165502, 10.11220174261750593 ) ) ;
#8610=LINE ( 'NONE', #4864, #10758 ) ;
#8615=ORIENTED_EDGE ( 'NONE', *, *, #13288, .F. ) ;
#8616=VERTEX_POINT ( 'NONE', #5993 ) ;
#8623=CARTESIAN_POINT ( 'NONE',  ( -1.461580736456473018, 186.3499999989075206, 5.538419263543527649 ) ) ;
#8630=CARTESIAN_POINT ( 'NONE',  ( -2.521794825564176890, 226.7667903661470348, 5.788166807254388146 ) ) ;
#8631=APPLICATION_CONTEXT ( 'automotive_design' ) ;
#8643=DIRECTION ( 'NONE',  ( 6.123233995738439900E-17, 0.000000000000000000, -1.000000000000000000 ) ) ;
#8650=CARTESIAN_POINT ( 'NONE',  ( 2.500000000000000000, 189.4499999978150697, 8.035533905932739529 ) ) ;
#8651=CARTESIAN_POINT ( 'NONE',  ( 2.998712701283978710, 227.3219367242041926, 7.423021690895281743 ) ) ;
#8652=CARTESIAN_POINT ( 'NONE',  ( -0.3319738467526104908, 189.0000000000805187, 9.481785014843145731 ) ) ;
#8664=CARTESIAN_POINT ( 'NONE',  ( -7.352245982167326943E-16, 188.5300000002185072, 9.500000000000001776 ) ) ;
#8666=CARTESIAN_POINT ( 'NONE',  ( 1.964981070171530675, 228.3669111765908895, 7.299051262003229290 ) ) ;
#8672=CARTESIAN_POINT ( 'NONE',  ( -2.066987300000000527, 185.4499999989075150, 7.000000000000000000 ) ) ;
#8674=CARTESIAN_POINT ( 'NONE',  ( -4.946672411965113980E-16, 185.8499999989075206, 9.066987300000000971 ) ) ;
#8676=CARTESIAN_POINT ( 'NONE',  ( -2.500000000000000444, 184.4000000000000057, 7.000000000000000000 ) ) ;
#8681=CARTESIAN_POINT ( 'NONE',  ( -2.127985206219880077, 189.0000000000000000, 5.658978462642562768 ) ) ;
#8691=CARTESIAN_POINT ( 'NONE',  ( -0.8561741729129467293, 185.7999999989075093, 9.066987299999999195 ) ) ;
#8694=CARTESIAN_POINT ( 'NONE',  ( 0.000000000000000000, 184.0000000000000000, 7.000000000000000000 ) ) ;
#8705=CARTESIAN_POINT ( 'NONE',  ( -2.884911204282110120, 227.0244024278241000, 6.546979792117293862 ) ) ;
#8708=ORIENTED_EDGE ( 'NONE', *, *, #3135, .F. ) ;
#8716=CARTESIAN_POINT ( 'NONE',  ( -2.500000000000000444, 186.7499999978150242, 8.035533905932737753 ) ) ;
#8721=CARTESIAN_POINT ( 'NONE',  ( 1.035533905932737975, 184.9199999975965909, 4.500000000000000888 ) ) ;
#8722=CARTESIAN_POINT ( 'NONE',  ( -1.238081232355301875, 227.7501834494555055, 5.517906410191214306 ) ) ;
#8723=CARTESIAN_POINT ( 'NONE',  ( 2.900052503084635358, 227.0405808247315917, 6.594625917879634258 ) ) ;
#8732=CARTESIAN_POINT ( 'NONE',  ( 2.734553966056355812, 226.8926218724402020, 6.158846296097578055 ) ) ;
#8738=CARTESIAN_POINT ( 'NONE',  ( -1.767766952966369542, 184.5000000000000000, 8.767766952966368876 ) ) ;
#8741=CARTESIAN_POINT ( 'NONE',  ( 1.974798917232459150, 228.1755836975312945, 6.746486589875083872 ) ) ;
#8745=CARTESIAN_POINT ( 'NONE',  ( 1.035533905932737975, 184.1500000000000341, 4.500000000000000888 ) ) ;
#8747=CARTESIAN_POINT ( 'NONE',  ( 2.066987299999999639, 188.4999999989075263, 6.143825827087054492 ) ) ;
#8752=( NAMED_UNIT ( * ) PLANE_ANGLE_UNIT ( ) SI_UNIT ( $, .RADIAN. ) );
#8753=CARTESIAN_POINT ( 'NONE',  ( -5.999999999999999112, 221.4150671951173592, 6.196499129422101682 ) ) ;
#8754=CARTESIAN_POINT ( 'NONE',  ( -2.066987300000000971, 188.6499999989075036, 7.000000000000000000 ) ) ;
#8756=CARTESIAN_POINT ( 'NONE',  ( 0.08805000471466810363, 188.9999999996602469, 9.502418226916221400 ) ) ;
#8762=VERTEX_POINT ( 'NONE', #11534 ) ;
#8763=CARTESIAN_POINT ( 'NONE',  ( -2.066987300000000083, 187.1999999989075434, 6.143825827087054492 ) ) ;
#8766=EDGE_CURVE ( 'NONE', #14218, #8478, #8515, .T. ) ;
#8774=CARTESIAN_POINT ( 'NONE',  ( -0.9143442643220817123, 228.2093053035189030, 10.03355751118253636 ) ) ;
#8783=CARTESIAN_POINT ( 'NONE',  ( -1.827163138824825950, 228.0559401102076151, 9.582586618047248095 ) ) ;
#8786=ADVANCED_FACE ( 'NONE', ( #8044 ), #5205, .T. ) ;
#8789=CARTESIAN_POINT ( 'NONE',  ( 0.2558939153494951824, 188.9999999999999716, 4.506307806592411147 ) ) ;
#8801=CARTESIAN_POINT ( 'NONE',  ( -1.767766952966369542, 186.0699999975965397, 8.767766952966368876 ) ) ;
#8802=CARTESIAN_POINT ( 'NONE',  ( 0.5174937098143853609, 227.6312805367891201, 5.174508016632918483 ) ) ;
#8803=CARTESIAN_POINT ( 'NONE',  ( -2.842171547016528965, 226.9791356524935395, 6.413666598675894726 ) ) ;
#8804=CARTESIAN_POINT ( 'NONE',  ( -2.233311234937184420, 189.1493003526281882, 9.186062866647521474 ) ) ;
#8811=CARTESIAN_POINT ( 'NONE',  ( 2.421481774831334199, 227.8602969206058617, 9.007210671174304295 ) ) ;
#8816=CARTESIAN_POINT ( 'NONE',  ( -1.767766952966369765, 186.0999999999999943, 8.767766952966368876 ) ) ;
#8818=CARTESIAN_POINT ( 'NONE',  ( -1.690976820968455474, 227.9165037442230926, 5.998248907768082283 ) ) ;
#8824=CARTESIAN_POINT ( 'NONE',  ( 2.500000000000000444, 184.0500000000000114, 5.964466094067262247 ) ) ;
#8826=CARTESIAN_POINT ( 'NONE',  ( -0.8561741729129456191, 188.6999999989075150, 4.933012699999999029 ) ) ;
#8832=CARTESIAN_POINT ( 'NONE',  ( -5.999999999999999112, 189.3270225533669020, 3.938484906660875584 ) ) ;
#8835=CARTESIAN_POINT ( 'NONE',  ( 2.995127566766980554, 189.8664680706473007, 7.560295519963911914 ) ) ;
#8836=CARTESIAN_POINT ( 'NONE',  ( -1.035533905932737975, 188.1499999978150584, 4.500000000000001776 ) ) ;
#8837=CARTESIAN_POINT ( 'NONE',  ( 2.696147639476683455, 189.8139822597015609, 8.673643915089936485 ) ) ;
#8840=CARTESIAN_POINT ( 'NONE',  ( -0.1647438929007866704, 188.9999999999999716, 4.500000000000000000 ) ) ;
#8842=CARTESIAN_POINT ( 'NONE',  ( 0.8561741729129452860, 188.5999999989074922, 4.933012699999999029 ) ) ;
#8859=CARTESIAN_POINT ( 'NONE',  ( -1.767766952966369320, 187.4300000002185129, 5.232233047033630235 ) ) ;
#8865=VERTEX_POINT ( 'NONE', #10742 ) ;
#8878=CARTESIAN_POINT ( 'NONE',  ( -2.500000000000000444, 186.6499999978150299, 5.964466094067261359 ) ) ;
#8880=EDGE_CURVE ( 'NONE', #3363, #5259, #7849, .T. ) ;
#8885=CARTESIAN_POINT ( 'NONE',  ( 1.035533905932737975, 186.5199999975966136, 4.500000000000000888 ) ) ;
#8886=CARTESIAN_POINT ( 'NONE',  ( -1.160340649284625325, 228.7901875120212196, 8.521497460825987247 ) ) ;
#8887=CARTESIAN_POINT ( 'NONE',  ( -2.884911204282110120, 227.0244024278241000, 6.546979792117293862 ) ) ;
#8888=CARTESIAN_POINT ( 'NONE',  ( -1.008179592313656059, 189.0000000000697469, 9.292056966037035792 ) ) ;
#8894=CARTESIAN_POINT ( 'NONE',  ( 2.129007923468051455, 227.9697339865814740, 9.329065678806253814 ) ) ;
#8900=CARTESIAN_POINT ( 'NONE',  ( 2.500000000000000444, 184.7500000000000000, 8.035533905932739529 ) ) ;
#8902=CARTESIAN_POINT ( 'NONE',  ( -0.4523656679209748233, 227.6256624317788635, 5.158282608927489576 ) ) ;
#8906=CARTESIAN_POINT ( 'NONE',  ( 2.500000000000000444, 184.7500000000000000, 8.035533905932739529 ) ) ;
#8909=CARTESIAN_POINT ( 'NONE',  ( 0.8561741729129457301, 189.0999999989075206, 9.066987299999999195 ) ) ;
#8915=CARTESIAN_POINT ( 'NONE',  ( 2.494052150861849171, 189.1790225982191487, 8.847987137205636898 ) ) ;
#8922=CARTESIAN_POINT ( 'NONE',  ( -1.461580736456472795, 185.5499999989075093, 5.538419263543527649 ) ) ;
#8932=CARTESIAN_POINT ( 'NONE',  ( -1.318079107690499852, 228.1589215201366869, 9.885401715239364506 ) ) ;
#8933=CARTESIAN_POINT ( 'NONE',  ( 0.8561741729129451750, 189.3999999989075604, 4.933012699999999029 ) ) ;
#8943=ORIENTED_EDGE ( 'NONE', *, *, #11721, .T. ) ;
#8948=CARTESIAN_POINT ( 'NONE',  ( 2.046085422626991779, 189.0000000000000568, 8.444739450853276708 ) ) ;
#8951=B_SPLINE_CURVE_WITH_KNOTS ( 'NONE', 1,
 ( #7239, #2454 ),
 .UNSPECIFIED., .F., .F.,
 ( 2, 2 ),
 ( 0.000000000000000000, 1.000000000000000000 ),
 .UNSPECIFIED. ) ;
#8955=CARTESIAN_POINT ( 'NONE',  ( -1.035533905932737975, 187.3499999978151038, 4.500000000000000888 ) ) ;
#8957=EDGE_CURVE ( 'NONE', #4790, #12014, #8610, .T. ) ;
#8960=CARTESIAN_POINT ( 'NONE',  ( -2.500000000000000444, 186.7699999975965568, 7.000000000000000000 ) ) ;
#8961=CARTESIAN_POINT ( 'NONE',  ( 1.747590535343585438, 228.0744605602133674, 9.637048244069795544 ) ) ;
#8962=CARTESIAN_POINT ( 'NONE',  ( -2.381136272098726803, 226.7019369474745361, 5.597090573316407358 ) ) ;
#8972=CARTESIAN_POINT ( 'NONE',  ( 1.295909982280349482, 228.1605777260576531, 9.890276522793730152 ) ) ;
#8973=EDGE_CURVE ( 'NONE', #14218, #5590, #9694, .T. ) ;
#8976=CARTESIAN_POINT ( 'NONE',  ( -2.500000000000000888, 188.3999999999999773, 7.000000000000000000 ) ) ;
#8979=CARTESIAN_POINT ( 'NONE',  ( 1.767766952966368654, 185.5000000000000000, 8.767766952966368876 ) ) ;
#8980=CARTESIAN_POINT ( 'NONE',  ( -0.7022813136239680620, 227.6507649362739585, 5.230780073663146013 ) ) ;
#8986=CARTESIAN_POINT ( 'NONE',  ( 2.500000000000000444, 184.0000000000000000, 7.000000000000000000 ) ) ;
#8989=CARTESIAN_POINT ( 'NONE',  ( 0.8561741729129452860, 189.3999999989075889, 4.933012699999999029 ) ) ;
#8996=CARTESIAN_POINT ( 'NONE',  ( 3.003420313107258988, 189.8839437108406969, 7.169374865749266412 ) ) ;
#8998=CARTESIAN_POINT ( 'NONE',  ( 1.513225566872929750, 189.7309853354881852, 9.978542870372216100 ) ) ;
#9003=CARTESIAN_POINT ( 'NONE',  ( -1.461580736456473462, 188.1499999989075320, 8.461580736456472351 ) ) ;
#9005=VERTEX_POINT ( 'NONE', #13591 ) ;
#9009=FACE_OUTER_BOUND ( 'NONE', #1892, .T. ) ;
#9031=ADVANCED_FACE ( 'NONE', ( #5336 ), #3456, .T. ) ;
#9034=CARTESIAN_POINT ( 'NONE',  ( 2.500000000000000444, 184.7499999978150527, 5.964466094067262247 ) ) ;
#9039=CARTESIAN_POINT ( 'NONE',  ( -1.767766952966369320, 186.6699999975965625, 5.232233047033630235 ) ) ;
#9040=CARTESIAN_POINT ( 'NONE',  ( -1.052533753945321227, 228.8137749680355455, 8.589619379135912780 ) ) ;
#9041=CARTESIAN_POINT ( 'NONE',  ( -2.440032737085090275, 227.8520529458832300, 8.982935890751354790 ) ) ;
#9050=CARTESIAN_POINT ( 'NONE',  ( 1.232202550405030683, 228.1699143606124380, 9.917725425114751303 ) ) ;
#9057=CARTESIAN_POINT ( 'NONE',  ( 2.500000000000000000, 188.7999999999999829, 7.000000000000000000 ) ) ;
#9058=CARTESIAN_POINT ( 'NONE',  ( -2.500000000000000888, 187.6500000000000341, 8.035533905932737753 ) ) ;
#9059=CARTESIAN_POINT ( 'NONE',  ( -1.740752211025599738, 227.9442165381023528, 6.078285037125840340 ) ) ;
#9064=CARTESIAN_POINT ( 'NONE',  ( -1.035533905932739529, 185.3499999999999659, 9.500000000000003553 ) ) ;
#9065=CARTESIAN_POINT ( 'NONE',  ( -4.743384504624081899E-17, 187.2999999978150356, 4.500000000000000000 ) ) ;
#9066=CARTESIAN_POINT ( 'NONE',  ( 2.066987300000000083, 186.8499999989075206, 7.000000000000000000 ) ) ;
#9070=( BOUNDED_CURVE ( )  B_SPLINE_CURVE ( 2, ( #11830, #15429, #9304, #1973, #5803, #701, #4292, #1895, #6850 ),
 .UNSPECIFIED., .F., .F. ) 
 B_SPLINE_CURVE_WITH_KNOTS ( ( 3, 2, 2, 2, 3 ),
 ( 0.07142857142857142461, 0.08928571428571428770, 0.1071428571428571369, 0.1250000000000000000, 0.1428571428571428492 ),
 .UNSPECIFIED. ) 
 CURVE ( )  GEOMETRIC_REPRESENTATION_ITEM ( )  RATIONAL_B_SPLINE_CURVE ( ( 1.000000000000000000, 0.9238795325112867385, 1.000000000000000000, 0.9238795325112867385, 1.000000000000000000, 0.9238795325112867385, 1.000000000000000000, 0.9238795325112867385, 1.000000000000000000 ) ) 
 REPRESENTATION_ITEM ( '' )  );
#9071=CARTESIAN_POINT ( 'NONE',  ( -5.999999999999999112, 185.8606548077538321, 9.048340948986950849 ) ) ;
#9073=EDGE_CURVE ( 'NONE', #2326, #2929, #14334, .T. ) ;
#9074=CARTESIAN_POINT ( 'NONE',  ( 2.463761206207551346, 189.9754024155355694, 5.513296855513769579 ) ) ;
#9083=CARTESIAN_POINT ( 'NONE',  ( -0.8561741729129457301, 186.0999999989074922, 4.933012699999999029 ) ) ;
#9084=ORIENTED_EDGE ( 'NONE', *, *, #14690, .T. ) ;
#9096=CARTESIAN_POINT ( 'NONE',  ( -0.1960076320828026963, 228.2536001344089982, 10.16376666290868336 ) ) ;
#9110=CARTESIAN_POINT ( 'NONE',  ( 1.035533905932737753, 189.6499999978150868, 4.500000000000000888 ) ) ;
#9114=CARTESIAN_POINT ( 'NONE',  ( 2.500000000000000000, 188.7699999975965568, 7.000000000000000000 ) ) ;
#9115=CARTESIAN_POINT ( 'NONE',  ( -1.886200273035058439, 228.4697824026276294, 7.596149230188033563 ) ) ;
#9116=CARTESIAN_POINT ( 'NONE',  ( -2.898051746902431614, 227.0396595591786308, 6.591911377507474690 ) ) ;
#9132=CARTESIAN_POINT ( 'NONE',  ( -2.500000000000000888, 188.3999999999999773, 7.000000000000000000 ) ) ;
#9133=CARTESIAN_POINT ( 'NONE',  ( -0.6404026449181154934, 227.6435107573390724, 5.209829591148105621 ) ) ;
#9136=EDGE_CURVE ( 'NONE', #7504, #12468, #1990, .T. ) ;
#9138=CARTESIAN_POINT ( 'NONE',  ( 1.035533905932737975, 185.7500000000000568, 4.500000000000000888 ) ) ;
#9139=CARTESIAN_POINT ( 'NONE',  ( -2.500000000000000444, 184.0000000000000000, 7.000000000000000000 ) ) ;
#9145=CARTESIAN_POINT ( 'NONE',  ( -0.0003580824083057882324, 226.3251816641676726, 4.486670979270475534 ) ) ;
#9147=CARTESIAN_POINT ( 'NONE',  ( 2.491866682565489377, 188.9999999978042524, 7.260727731289393638 ) ) ;
#9150=CARTESIAN_POINT ( 'NONE',  ( 1.496490727326450720, 228.6905582067893477, 8.233762344832721070 ) ) ;
#9155=CARTESIAN_POINT ( 'NONE',  ( 2.066987300000000083, 186.5999999989074922, 7.856174172912946396 ) ) ;
#9159=EDGE_CURVE ( 'NONE', #15176, #14218, #3224, .T. ) ;
#9163=CARTESIAN_POINT ( 'NONE',  ( 0.8561741729129458411, 184.3999999989075320, 4.933012699999999029 ) ) ;
#9167=CARTESIAN_POINT ( 'NONE',  ( 0.000000000000000000, 215.7452399395091049, 13.29567785264566027 ) ) ;
#9181=CARTESIAN_POINT ( 'NONE',  ( 1.767766952966368432, 187.7999999978150356, 8.767766952966368876 ) ) ;
#9182=CARTESIAN_POINT ( 'NONE',  ( 9.825582188149883933E-17, 184.8999999978150584, 4.500000000000000000 ) ) ;
#9184=SHAPE_DEFINITION_REPRESENTATION ( #15297, #11283 ) ;
#9186=CARTESIAN_POINT ( 'NONE',  ( -1.016439536705160407E-16, 188.1699999975965625, 4.500000000000000000 ) ) ;
#9187=CARTESIAN_POINT ( 'NONE',  ( 1.583222688839772019, 228.1098062731747689, 9.740983991995673108 ) ) ;
#9191=ORIENTED_EDGE ( 'NONE', *, *, #4080, .F. ) ;
#9198=FILL_AREA_STYLE ('',( #7918 ) ) ;
#9203=CARTESIAN_POINT ( 'NONE',  ( -1.767766952966369098, 184.9999999978150527, 5.232233047033630235 ) ) ;
#9205=CARTESIAN_POINT ( 'NONE',  ( 0.3900692251286368428, 228.2474522196246767, 10.14569219465573546 ) ) ;
#9212=CARTESIAN_POINT ( 'NONE',  ( -1.767766952966369765, 186.0999999999999943, 8.767766952966368876 ) ) ;
#9217=CARTESIAN_POINT ( 'NONE',  ( -2.500000000000000444, 186.7500000000000000, 5.964466094067261359 ) ) ;
#9218=CARTESIAN_POINT ( 'NONE',  ( -1.016439536705160407E-17, 228.2551366889529731, 10.16828399152529272 ) ) ;
#9222=CARTESIAN_POINT ( 'NONE',  ( 0.08612881260894005020, 189.4418673018899142, 3.980892592272581076 ) ) ;
#9223=CARTESIAN_POINT ( 'NONE',  ( -1.035533905932737975, 185.7800000002185072, 4.500000000000000888 ) ) ;
#9225=CARTESIAN_POINT ( 'NONE',  ( 0.7014106675288342974, 228.8704641679326244, 8.753341021778663134 ) ) ;
#9230=CARTESIAN_POINT ( 'NONE',  ( 0.000000000000000000, 186.0499999989075093, 4.933012699999999029 ) ) ;
#9235=CARTESIAN_POINT ( 'NONE',  ( 8.809142651444723526E-17, 184.6499999989075320, 4.933012699999999029 ) ) ;
#9236=CARTESIAN_POINT ( 'NONE',  ( 2.500000000000000444, 184.0000000000000000, 7.000000000000000000 ) ) ;
#9237=CARTESIAN_POINT ( 'NONE',  ( -4.302927372051845722E-16, 184.8499999989074922, 9.066987300000000971 ) ) ;
#9241=CARTESIAN_POINT ( 'NONE',  ( 0.000000000000000000, 194.5935680195190116, 12.11154058223188201 ) ) ;
#9253=CARTESIAN_POINT ( 'NONE',  ( 1.767766952966369320, 184.9000000000000057, 5.232233047033630235 ) ) ;
#9257=CARTESIAN_POINT ( 'NONE',  ( -7.352245982167326943E-16, 188.4999999978150527, 9.500000000000001776 ) ) ;
#9258=CARTESIAN_POINT ( 'NONE',  ( -2.499999999999999556, 185.0499999978150072, 5.964466094067259583 ) ) ;
#9264=CARTESIAN_POINT ( 'NONE',  ( 1.628454131612142364, 226.4793820939146372, 4.941229787183066158 ) ) ;
#9274=CARTESIAN_POINT ( 'NONE',  ( 0.000000000000000000, 184.0000000000000000, 7.000000000000000000 ) ) ;
#9281=CARTESIAN_POINT ( 'NONE',  ( 2.500000000000000444, 184.6999999978150697, 7.000000000000000000 ) ) ;
#9283=CARTESIAN_POINT ( 'NONE',  ( -1.770887355114397321, 228.5581793045761287, 7.851444524843710582 ) ) ;
#9287=CARTESIAN_POINT ( 'NONE',  ( -1.035533905932737975, 186.6500000000000057, 4.500000000000000888 ) ) ;
#9292=CARTESIAN_POINT ( 'NONE',  ( -0.0007161861819565282445, 226.3251816840472657, 4.486671040222605988 ) ) ;
#9293=CARTESIAN_POINT ( 'NONE',  ( -2.048913241472479108, 189.7603925237210660, 9.570315070074567387 ) ) ;
#9295=CARTESIAN_POINT ( 'NONE',  ( -1.035533905932737753, 184.1800000002185129, 4.500000000000000888 ) ) ;
#9296=CARTESIAN_POINT ( 'NONE',  ( -1.990566740715900895, 228.1747751937680846, 6.744151584892693840 ) ) ;
#9297=CARTESIAN_POINT ( 'NONE',  ( 1.984153134209927671, 228.3142122347729526, 7.146853712282291049 ) ) ;
#9303=CARTESIAN_POINT ( 'NONE',  ( 9.825582188149883933E-17, 184.4499999989075150, 4.933012699999999029 ) ) ;
#9304=CARTESIAN_POINT ( 'NONE',  ( -1.767766952966369542, 184.5000000000000000, 8.767766952966368876 ) ) ;
#9305=EDGE_CURVE ( 'NONE', #12468, #14260, #15054, .T. ) ;
#9308=CARTESIAN_POINT ( 'NONE',  ( -2.500000000000000444, 186.0499999999999829, 8.035533905932737753 ) ) ;
#9311=CARTESIAN_POINT ( 'NONE',  ( -2.066987300000000971, 186.2999999989075093, 7.856174172912944620 ) ) ;
#9315=CARTESIAN_POINT ( 'NONE',  ( -5.999999999999999112, 202.3202208672780102, 7.308763624254441815 ) ) ;
#9323=CARTESIAN_POINT ( 'NONE',  ( 0.6427959281715842632, 227.6423845907872021, 5.206577157913290677 ) ) ;
#9329=CARTESIAN_POINT ( 'NONE',  ( -1.035533905932739751, 188.4499999978150413, 9.500000000000003553 ) ) ;
#9332=CARTESIAN_POINT ( 'NONE',  ( 4.743384504624081899E-17, 185.6999999978150697, 4.500000000000000000 ) ) ;
#9336=CARTESIAN_POINT ( 'NONE',  ( 2.976061188595913176, 227.1638826975962502, 6.957706536906315797 ) ) ;
#9337=CARTESIAN_POINT ( 'NONE',  ( -1.328763708711319325, 228.1557872355912195, 9.876186263205003257 ) ) ;
#9340=CARTESIAN_POINT ( 'NONE',  ( 2.500000000000000000, 188.6499999978150584, 8.035533905932739529 ) ) ;
#9355=CARTESIAN_POINT ( 'NONE',  ( 1.035533905932737753, 188.9499999999999886, 4.500000000000000888 ) ) ;
#9358=CARTESIAN_POINT ( 'NONE',  ( -0.7013870287959992345, 228.8704690996177646, 8.753355264767147759 ) ) ;
#9362=CARTESIAN_POINT ( 'NONE',  ( 1.767766952966368432, 187.0999999999999943, 8.767766952966368876 ) ) ;
#9371=CARTESIAN_POINT ( 'NONE',  ( -2.684371489741315120, 227.7208608295982799, 8.597006646416071263 ) ) ;
#9372=( LENGTH_UNIT ( ) NAMED_UNIT ( * ) SI_UNIT ( .MILLI., .METRE. ) );
#9376=CARTESIAN_POINT ( 'NONE',  ( 1.452733574390970395, 228.7063250495755540, 8.279297886081021574 ) ) ;
#9378=LINE ( 'NONE', #15266, #164 ) ;
#9381=CARTESIAN_POINT ( 'NONE',  ( -2.066987300000000971, 184.5999999989074922, 6.143825827087054492 ) ) ;
#9385=VECTOR ( 'NONE', #5809, 1000.000000000000000 ) ;
#9386=CARTESIAN_POINT ( 'NONE',  ( 2.066987300000000083, 184.4999999989074979, 6.143825827087054492 ) ) ;
#9388=CARTESIAN_POINT ( 'NONE',  ( 2.066987300000000083, 186.5999999989074922, 7.856174172912946396 ) ) ;
#9392=CARTESIAN_POINT ( 'NONE',  ( -5.999999999999999112, 215.0542865858234336, 7.296348638347391891 ) ) ;
#9401=CARTESIAN_POINT ( 'NONE',  ( 2.066987300000000083, 184.4499999989075150, 7.000000000000000000 ) ) ;
#9408=CARTESIAN_POINT ( 'NONE',  ( 2.500000000000000444, 187.8499999978150470, 8.035533905932739529 ) ) ;
#9411=CARTESIAN_POINT ( 'NONE',  ( 1.035533905932737975, 185.6499999978150584, 4.500000000000001776 ) ) ;
#9412=EDGE_CURVE ( 'NONE', #9005, #7444, #2062, .T. ) ;
#9415=CARTESIAN_POINT ( 'NONE',  ( 1.767766952966369098, 188.8699999975965511, 5.232233047033630235 ) ) ;
#9416=CARTESIAN_POINT ( 'NONE',  ( 2.548737910730607403, 227.7996913757372397, 8.828908791204545636 ) ) ;
#9436=CARTESIAN_POINT ( 'NONE',  ( 1.767766952966369320, 184.7999999978150356, 5.232233047033630235 ) ) ;
#9437=CARTESIAN_POINT ( 'NONE',  ( -0.06495987523897406302, 228.9118723585069120, 8.872930237925691799 ) ) ;
#9441=CARTESIAN_POINT ( 'NONE',  ( -0.9975899816380627838, 189.4340297135221647, 4.147879558749815843 ) ) ;
#9442=CARTESIAN_POINT ( 'NONE',  ( 2.500000000000000444, 187.2500000000000000, 5.964466094067262247 ) ) ;
#9443=CARTESIAN_POINT ( 'NONE',  ( -2.500000000000000888, 188.3999999999999773, 7.000000000000000000 ) ) ;
#9449=CARTESIAN_POINT ( 'NONE',  ( -5.385276659965230388E-16, 226.3251816629291966, 4.486670979098442480 ) ) ;
#9450=CARTESIAN_POINT ( 'NONE',  ( -2.996310406655163572, 227.3383267913470149, 7.471278767517968156 ) ) ;
#9452=CARTESIAN_POINT ( 'NONE',  ( -1.035533905932739529, 184.4800000002184959, 9.500000000000003553 ) ) ;
#9454=CARTESIAN_POINT ( 'NONE',  ( 1.132923824227977772, 228.7961917368426157, 8.538838004569329954 ) ) ;
#9457=AXIS2_PLACEMENT_3D ( 'NONE', #9274, #13958, #6968 ) ;
#9460=CARTESIAN_POINT ( 'NONE',  ( 0.8561741729129457301, 186.7999999989074809, 4.933012699999999029 ) ) ;
#9469=CARTESIAN_POINT ( 'NONE',  ( 2.066987300000000527, 185.8499999989074922, 7.000000000000000000 ) ) ;
#9473=CARTESIAN_POINT ( 'NONE',  ( 0.000000000000000000, 186.5669965222008386, 9.317226423031119253 ) ) ;
#9476=( BOUNDED_SURFACE ( )  B_SPLINE_SURFACE ( 1, 2, ( 
 ( #7083, #9386, #10426, #11919, #9235, #12798, #11763, #1900, #14224, #3179, #11690, #10502, #3331, #4454, #14149, #3251, #8118, #2056, #865, #8199, #10576, #13831, #8922, #12483, #2864, #7557, #390, #8691, #2944, #5178, #7792, #11215, #1505, #2785, #5260, #10107, #15037, #1739, #14962, #7638, #10184, #10262, #2707, #11368, #9954, #316, #3818, #6614, #1583, #4051, #10031, #13521, #13756, #240, #5416, #8763, #6381, #14879, #2628, #6461, #11293, #547, #12406, #11140, #5102, #7712, #12329, #12562, #1660, #6534, #7484, #470, #5341, #4131, #9003, #12639, #1424, #3968, #11446, #6299, #14805, #3890, #13597, #8842, #13674, #6688, #699, #2051, #6849, #936, #10339, #12789, #4526, #5573, #8193, #15353, #861, #4448, #6926, #7949, #13990 ),
 ( #10570, #7876, #11758, #7000, #9303, #4371, #14142, #9381, #3246, #8029, #8114, #3097, #11685, #4213, #14219, #10419, #3327, #6768, #1893, #14064, #784, #5647, #15427, #13028, #10497, #3172, #5728, #5802, #11600, #2127, #5495, #15270, #15115, #11829, #12867, #12951, #9230, #9083, #13908, #11522, #3020, #4291, #1971, #12717, #1816, #623, #15193, #9155, #9540, #13347, #1331, #9460, #3482, #7237, #9783, #14629, #3565, #12076, #11995, #8596, #13107, #9625, #15587, #2534, #10648, #4690, #4767, #14544, #13430, #8353, #11912, #2369, #1175, #9706, #6043, #1099, #2452, #1020, #5962, #8434, #15666, #8270, #5883, #10889, #1253, #7388, #10807, #12154, #14377, #3641, #5030, #7315, #3719, #13191, #4851, #3401, #8517, #6129, #10965, #7158, #2208 ) ),
 .UNSPECIFIED., .F., .F., .F. ) 
 B_SPLINE_SURFACE_WITH_KNOTS ( ( 2, 2 ),
 ( 3, 2, 2, 2, 2, 2, 2, 2, 2, 2, 2, 2, 2, 2, 2, 2, 2, 2, 2, 2, 2, 2, 2, 2, 2, 2, 2, 2, 2, 2, 2, 2, 2, 2, 2, 2, 2, 2, 2, 2, 2, 2, 2, 2, 2, 2, 2, 2, 2, 2, 3 ),
 ( 0.000000000000000000, 1.000000000000000000 ),
 ( 0.000000000000000000, 0.01785714285714285615, 0.03571428571428571230, 0.05357142857142856845, 0.07142857142857142461, 0.08928571428571428770, 0.1071428571428571369, 0.1250000000000000000, 0.1428571428571428492, 0.1607142857142857262, 0.1785714285714285754, 0.1964285714285714246, 0.2142857142857142738, 0.2321428571428571508, 0.2500000000000000000, 0.2678571428571428492, 0.2857142857142856984, 0.3035714285714285476, 0.3214285714285714524, 0.3392857142857143016, 0.3571428571428571508, 0.3750000000000000000, 0.3928571428571428492, 0.4107142857142856984, 0.4285714285714285476, 0.4464285714285714524, 0.4642857142857143016, 0.4821428571428571508, 0.5000000000000000000, 0.5178571428571429047, 0.5357142857142856984, 0.5535714285714286031, 0.5714285714285713969, 0.5892857142857143016, 0.6071428571428570953, 0.6250000000000000000, 0.6428571428571429047, 0.6607142857142856984, 0.6785714285714286031, 0.6964285714285713969, 0.7142857142857143016, 0.7321428571428570953, 0.7500000000000000000, 0.7678571428571429047, 0.7857142857142856984, 0.8035714285714286031, 0.8214285714285713969, 0.8392857142857143016, 0.8571428571428570953, 0.8750000000000000000, 0.8928571428571429047 ),
 .UNSPECIFIED. ) 
 GEOMETRIC_REPRESENTATION_ITEM ( )  RATIONAL_B_SPLINE_SURFACE ( (
 ( 1.000000000000000000, 0.9238795325112867385, 1.000000000000000000, 0.9238795325112867385, 1.000000000000000000, 0.9238795325112867385, 1.000000000000000000, 0.9238795325112867385, 1.000000000000000000, 0.9238795325112867385, 1.000000000000000000, 0.9238795325112867385, 1.000000000000000000, 0.9238795325112867385, 1.000000000000000000, 0.9238795325112867385, 1.000000000000000000, 0.9238795325112867385, 1.000000000000000000, 0.9238795325112867385, 1.000000000000000000, 0.9238795325112867385, 1.000000000000000000, 0.9238795325112867385, 1.000000000000000000, 0.9238795325112867385, 1.000000000000000000, 0.9238795325112867385, 1.000000000000000000, 0.9238795325112867385, 1.000000000000000000, 0.9238795325112867385, 1.000000000000000000, 0.9238795325112867385, 1.000000000000000000, 0.9238795325112867385, 1.000000000000000000, 0.9238795325112867385, 1.000000000000000000, 0.9238795325112867385, 1.000000000000000000, 0.9238795325112867385, 1.000000000000000000, 0.9238795325112867385, 1.000000000000000000, 0.9238795325112867385, 1.000000000000000000, 0.9238795325112867385, 1.000000000000000000, 0.9238795325112867385, 1.000000000000000000, 0.9238795325112867385, 1.000000000000000000, 0.9238795325112867385, 1.000000000000000000, 0.9238795325112867385, 1.000000000000000000, 0.9238795325112867385, 1.000000000000000000, 0.9238795325112867385, 1.000000000000000000, 0.9238795325112867385, 1.000000000000000000, 0.9238795325112867385, 1.000000000000000000, 0.9238795325112867385, 1.000000000000000000, 0.9238795325112867385, 1.000000000000000000, 0.9238795325112867385, 1.000000000000000000, 0.9238795325112867385, 1.000000000000000000, 0.9238795325112867385, 1.000000000000000000, 0.9238795325112867385, 1.000000000000000000, 0.9238795325112867385, 1.000000000000000000, 0.9238795325112867385, 1.000000000000000000, 0.9238795325112867385, 1.000000000000000000, 0.9238795325112867385, 1.000000000000000000, 0.9238795325112867385, 1.000000000000000000, 0.9238795325112867385, 1.000000000000000000, 0.9238795325112867385, 1.000000000000000000, 0.9238795325112867385, 1.000000000000000000, 0.9238795325112867385, 1.000000000000000000, 0.9238795325112867385, 1.000000000000000000, 0.9238795325112867385, 1.000000000000000000, 0.9238795325112867385, 1.000000000000000000),
 ( 1.000000000000000000, 0.9238795325112867385, 1.000000000000000000, 0.9238795325112867385, 1.000000000000000000, 0.9238795325112867385, 1.000000000000000000, 0.9238795325112867385, 1.000000000000000000, 0.9238795325112867385, 1.000000000000000000, 0.9238795325112867385, 1.000000000000000000, 0.9238795325112867385, 1.000000000000000000, 0.9238795325112867385, 1.000000000000000000, 0.9238795325112867385, 1.000000000000000000, 0.9238795325112867385, 1.000000000000000000, 0.9238795325112867385, 1.000000000000000000, 0.9238795325112867385, 1.000000000000000000, 0.9238795325112867385, 1.000000000000000000, 0.9238795325112867385, 1.000000000000000000, 0.9238795325112867385, 1.000000000000000000, 0.9238795325112867385, 1.000000000000000000, 0.9238795325112867385, 1.000000000000000000, 0.9238795325112867385, 1.000000000000000000, 0.9238795325112867385, 1.000000000000000000, 0.9238795325112867385, 1.000000000000000000, 0.9238795325112867385, 1.000000000000000000, 0.9238795325112867385, 1.000000000000000000, 0.9238795325112867385, 1.000000000000000000, 0.9238795325112867385, 1.000000000000000000, 0.9238795325112867385, 1.000000000000000000, 0.9238795325112867385, 1.000000000000000000, 0.9238795325112867385, 1.000000000000000000, 0.9238795325112867385, 1.000000000000000000, 0.9238795325112867385, 1.000000000000000000, 0.9238795325112867385, 1.000000000000000000, 0.9238795325112867385, 1.000000000000000000, 0.9238795325112867385, 1.000000000000000000, 0.9238795325112867385, 1.000000000000000000, 0.9238795325112867385, 1.000000000000000000, 0.9238795325112867385, 1.000000000000000000, 0.9238795325112867385, 1.000000000000000000, 0.9238795325112867385, 1.000000000000000000, 0.9238795325112867385, 1.000000000000000000, 0.9238795325112867385, 1.000000000000000000, 0.9238795325112867385, 1.000000000000000000, 0.9238795325112867385, 1.000000000000000000, 0.9238795325112867385, 1.000000000000000000, 0.9238795325112867385, 1.000000000000000000, 0.9238795325112867385, 1.000000000000000000, 0.9238795325112867385, 1.000000000000000000, 0.9238795325112867385, 1.000000000000000000, 0.9238795325112867385, 1.000000000000000000, 0.9238795325112867385, 1.000000000000000000, 0.9238795325112867385, 1.000000000000000000, 0.9238795325112867385, 1.000000000000000000) ) ) 
 REPRESENTATION_ITEM ( '' )  SURFACE ( )  );
#9483=VERTEX_POINT ( 'NONE', #5414 ) ;
#9484=( BOUNDED_CURVE ( )  B_SPLINE_CURVE ( 2, ( #8976, #1634, #11343, #7847, #13733, #11574, #2840, #10394, #599 ),
 .UNSPECIFIED., .F., .F. ) 
 B_SPLINE_CURVE_WITH_KNOTS ( ( 3, 2, 2, 2, 3 ),
 ( 0.7857142857142856984, 0.8035714285714286031, 0.8214285714285713969, 0.8392857142857143016, 0.8571428571428570953 ),
 .UNSPECIFIED. ) 
 CURVE ( )  GEOMETRIC_REPRESENTATION_ITEM ( )  RATIONAL_B_SPLINE_CURVE ( ( 1.000000000000000000, 0.9238795325112867385, 1.000000000000000000, 0.9238795325112867385, 1.000000000000000000, 0.9238795325112867385, 1.000000000000000000, 0.9238795325112867385, 1.000000000000000000 ) ) 
 REPRESENTATION_ITEM ( '' )  );
#9489=CARTESIAN_POINT ( 'NONE',  ( 0.8561741729129455081, 186.1999999989075150, 4.933012699999999029 ) ) ;
#9495=CARTESIAN_POINT ( 'NONE',  ( 2.990158053860457077, 227.3692281962998436, 7.562228658338257858 ) ) ;
#9496=CARTESIAN_POINT ( 'NONE',  ( 0.000000000000000000, 184.0000000000000000, 7.000000000000000000 ) ) ;
#9506=ORIENTED_EDGE ( 'NONE', *, *, #10911, .F. ) ;
#9516=CARTESIAN_POINT ( 'NONE',  ( 1.767766952966369098, 189.5999999978150470, 5.232233047033630235 ) ) ;
#9517=CARTESIAN_POINT ( 'NONE',  ( -1.886200273035058439, 228.4697824026276294, 7.596149230188033563 ) ) ;
#9519=CARTESIAN_POINT ( 'NONE',  ( -0.3320323468824299962, 190.0863194065883022, 4.213467285827682041 ) ) ;
#9531=CARTESIAN_POINT ( 'NONE',  ( -2.817344785281778563, 226.9578842961288103, 6.351048551979458168 ) ) ;
#9533=CARTESIAN_POINT ( 'NONE',  ( 1.035533905932738197, 186.1800000002184845, 9.500000000000003553 ) ) ;
#9535=CARTESIAN_POINT ( 'NONE',  ( -0.3251550031287174236, 227.6173728764936186, 5.134341900458684549 ) ) ;
#9539=ORIENTED_EDGE ( 'NONE', *, *, #8766, .T. ) ;
#9540=CARTESIAN_POINT ( 'NONE',  ( 2.066987300000000527, 186.6499999989075320, 7.000000000000000000 ) ) ;
#9541=CARTESIAN_POINT ( 'NONE',  ( -5.285485590866834116E-16, 186.4499999989075150, 9.066987300000000971 ) ) ;
#9551=CARTESIAN_POINT ( 'NONE',  ( 0.8561741729129457301, 185.9999999989074979, 4.933012699999999029 ) ) ;
#9561=ORIENTED_EDGE ( 'NONE', *, *, #2836, .T. ) ;
#9567=CARTESIAN_POINT ( 'NONE',  ( 0.8561741729129455081, 186.9999999989074979, 4.933012699999999029 ) ) ;
#9573=CARTESIAN_POINT ( 'NONE',  ( -0.6817270424356797198, 226.3498696214933545, 4.559454910794151772 ) ) ;
#9575=CYLINDRICAL_SURFACE ( 'NONE', #14338, 2.500000000000000444 ) ;
#9593=CARTESIAN_POINT ( 'NONE',  ( -2.500000000000000888, 188.3499999978150186, 8.035533905932737753 ) ) ;
#9595=CARTESIAN_POINT ( 'NONE',  ( 2.191560967657306680, 226.6301005958437145, 5.385416860794732585 ) ) ;
#9600=FACE_OUTER_BOUND ( 'NONE', #11799, .T. ) ;
#9609=DIRECTION ( 'NONE',  ( -6.123233995736766036E-17, 1.000000000000000000, 0.000000000000000000 ) ) ;
#9612=VECTOR ( 'NONE', #11840, 1000.000000000000000 ) ;
#9614=CARTESIAN_POINT ( 'NONE',  ( -1.191764142581503760, 226.4044614763379855, 4.720388933816794363 ) ) ;
#9616=CARTESIAN_POINT ( 'NONE',  ( -2.500000000000000888, 188.3300000002184902, 7.000000000000000000 ) ) ;
#9618=CARTESIAN_POINT ( 'NONE',  ( 0.8230742150784297051, 227.6668866512619047, 5.277340506070477666 ) ) ;
#9621=CARTESIAN_POINT ( 'NONE',  ( 1.496490727326450720, 228.6905582067893477, 8.233762344832721070 ) ) ;
#9623=CARTESIAN_POINT ( 'NONE',  ( 0.000000000000000000, 184.0000000000000000, 7.000000000000000000 ) ) ;
#9625=CARTESIAN_POINT ( 'NONE',  ( 0.8561741729129460632, 187.2999999989075661, 9.066987300000000971 ) ) ;
#9627=CARTESIAN_POINT ( 'NONE',  ( -2.066987300000000527, 184.6499999989075320, 7.000000000000000000 ) ) ;
#9628=CARTESIAN_POINT ( 'NONE',  ( -2.500000000000000444, 187.4999999978150527, 7.000000000000000000 ) ) ;
#9632=CARTESIAN_POINT ( 'NONE',  ( 5.999999999999999112, 221.4150671951173592, 6.196499129422101682 ) ) ;
#9633=CARTESIAN_POINT ( 'NONE',  ( 2.066987300000000083, 188.2499999989075263, 7.000000000000000000 ) ) ;
#9641=CARTESIAN_POINT ( 'NONE',  ( -1.035533905932737975, 187.4500000000000171, 4.500000000000001776 ) ) ;
#9653=CARTESIAN_POINT ( 'NONE',  ( -0.8561741729129456191, 188.6999999989075150, 4.933012699999999029 ) ) ;
#9660=CARTESIAN_POINT ( 'NONE',  ( -1.328763708711319325, 228.1557872355912195, 9.876186263205003257 ) ) ;
#9661=DIRECTION ( 'NONE',  ( -6.123233995736766036E-17, 1.000000000000000000, 0.000000000000000000 ) ) ;
#9665=ORIENTED_EDGE ( 'NONE', *, *, #2036, .T. ) ;
#9680=CARTESIAN_POINT ( 'NONE',  ( -1.767766952966369320, 188.1999999978150697, 5.232233047033630235 ) ) ;
#9681=CARTESIAN_POINT ( 'NONE',  ( 1.240393925004889208, 226.4108590421392933, 4.739248726333301853 ) ) ;
#9688=ORIENTED_EDGE ( 'NONE', *, *, #2036, .F. ) ;
#9690=CARTESIAN_POINT ( 'NONE',  ( 2.500000000000000444, 184.0000000000000000, 7.000000000000000000 ) ) ;
#9694=B_SPLINE_CURVE_WITH_KNOTS ( 'NONE', 3,
 ( #13826, #6376, #11363, #13751, #10258, #12323, #8998, #10025, #7633, #5173, #1500, #13667, #8837, #3885, #14800, #15110, #2780, #311, #2859, #2939, #1732, #9948, #12633, #3963, #7787, #542, #1578, #6456, #2701, #11288, #3014, #4208 ),
 .UNSPECIFIED., .F., .F.,
 ( 4, 2, 2, 2, 2, 2, 2, 2, 2, 2, 2, 2, 2, 2, 2, 4 ),
 ( 0.000000000000000000, 0.0005931748005980339630, 0.001186349601196067926, 0.001779524401794101889, 0.002372699202392135852, 0.002965874002990170465, 0.003559048803588205946, 0.004152223604186240126, 0.004745398404784276040, 0.005338573205382311088, 0.005931748005980345267, 0.007118097607176415362, 0.007711272407774453011, 0.008304447208372488926, 0.008897622008970526575, 0.009490796809568564224 ),
 .UNSPECIFIED. ) ;
#9699=CARTESIAN_POINT ( 'NONE',  ( -1.767766952966369765, 188.4300000002185129, 8.767766952966368876 ) ) ;
#9700=CARTESIAN_POINT ( 'NONE',  ( -1.889311774764879104, 228.4700178340609114, 7.596829169595165077 ) ) ;
#9701=CARTESIAN_POINT ( 'NONE',  ( 0.9660064634511277282, 228.8301302322938966, 8.636854315157751927 ) ) ;
#9704=ORIENTED_EDGE ( 'NONE', *, *, #11721, .F. ) ;
#9706=CARTESIAN_POINT ( 'NONE',  ( -2.066987300000001859, 187.8999999989075036, 7.856174172912944620 ) ) ;
#9708=CARTESIAN_POINT ( 'NONE',  ( 2.066987300000000527, 187.4499999989075150, 7.000000000000000000 ) ) ;
#9716=CARTESIAN_POINT ( 'NONE',  ( 0.8561741729129456191, 188.3999999989075036, 4.933012699999999029 ) ) ;
#9720=FACE_OUTER_BOUND ( 'NONE', #11870, .T. ) ;
#9735=CARTESIAN_POINT ( 'NONE',  ( 1.461580736456472573, 185.9499999989075150, 8.461580736456474128 ) ) ;
#9738=CARTESIAN_POINT ( 'NONE',  ( -1.016439536705160407E-17, 228.2551366889529731, 10.16828399152529272 ) ) ;
#9743=FACE_OUTER_BOUND ( 'NONE', #12738, .T. ) ;
#9744=CARTESIAN_POINT ( 'NONE',  ( -2.257095642740105212, 226.6533546677793538, 5.453940291146690988 ) ) ;
#9745=DIRECTION ( 'NONE',  ( -1.000000000000000000, 0.000000000000000000, 0.000000000000000000 ) ) ;
#9752=CARTESIAN_POINT ( 'NONE',  ( 1.767766952966368654, 185.5000000000000000, 8.767766952966368876 ) ) ;
#9762=CARTESIAN_POINT ( 'NONE',  ( -1.767766952966369320, 188.9999999978150527, 5.232233047033630235 ) ) ;
#9763=CARTESIAN_POINT ( 'NONE',  ( -0.1984404311693547251, 226.3267777912124075, 4.491376718485652120 ) ) ;
#9777=CARTESIAN_POINT ( 'NONE',  ( 1.767766952966368432, 188.6300000002185016, 8.767766952966368876 ) ) ;
#9779=CARTESIAN_POINT ( 'NONE',  ( 1.974531203966234827, 228.3459296953993203, 7.238455547615789243 ) ) ;
#9783=CARTESIAN_POINT ( 'NONE',  ( -1.461580736456473240, 186.9499999989075150, 5.538419263543526760 ) ) ;
#9784=CARTESIAN_POINT ( 'NONE',  ( -2.066987300000001415, 187.0999999989075206, 7.856174172912944620 ) ) ;
#9786=CARTESIAN_POINT ( 'NONE',  ( 2.066987299999999639, 185.1999999989075434, 7.856174172912946396 ) ) ;
#9790=CARTESIAN_POINT ( 'NONE',  ( 5.999999999999999112, 187.2933328889893403, 9.583808270834989429 ) ) ;
#9810=CARTESIAN_POINT ( 'NONE',  ( -0.8561741729129455081, 187.0999999989075206, 4.933012699999999029 ) ) ;
#9812=ADVANCED_FACE ( 'NONE', ( #3480 ), #3563, .T. ) ;
#9818=CARTESIAN_POINT ( 'NONE',  ( -2.753288529192227774, 227.6732037325579654, 8.456785184543583966 ) ) ;
#9821=ORIENTED_EDGE ( 'NONE', *, *, #14278, .F. ) ;
#9824=CARTESIAN_POINT ( 'NONE',  ( 2.174074108551606876, 189.0000000000000000, 5.753087109996226189 ) ) ;
#9834=CARTESIAN_POINT ( 'NONE',  ( -2.500000000000000444, 187.4499999978150981, 5.964466094067261359 ) ) ;
#9835=CARTESIAN_POINT ( 'NONE',  ( 2.379866841847371628, 227.8775224696199473, 9.057852156131547261 ) ) ;
#9836=CARTESIAN_POINT ( 'NONE',  ( -1.343479350821820129, 189.0800738899199018, 9.870497036542587921 ) ) ;
#9841=CARTESIAN_POINT ( 'NONE',  ( 0.000000000000000000, 184.0000000000000000, 7.000000000000000000 ) ) ;
#9843=CARTESIAN_POINT ( 'NONE',  ( 1.933170805762127076, 226.5518075033767786, 5.154678494461841787 ) ) ;
#9850=CARTESIAN_POINT ( 'NONE',  ( 2.500000000000000444, 186.3300000002185186, 7.000000000000000000 ) ) ;
#9853=CARTESIAN_POINT ( 'NONE',  ( 0.7014106675288342974, 228.8704641679326244, 8.753341021778663134 ) ) ;
#9858=CARTESIAN_POINT ( 'NONE',  ( -4.743384504624081899E-17, 186.8499999989074922, 4.933012699999999029 ) ) ;
#9868=CARTESIAN_POINT ( 'NONE',  ( -1.382083006809480485, 189.0000000000000000, 9.086164795105178271 ) ) ;
#9885=FACE_OUTER_BOUND ( 'NONE', #4096, .T. ) ;
#9894=CARTESIAN_POINT ( 'NONE',  ( -2.599074790483714370, 227.7726799100639994, 8.749447567440038043 ) ) ;
#9900=CARTESIAN_POINT ( 'NONE',  ( 0.5022380396211999498, 188.9999999999999716, 9.452991705245926468 ) ) ;
#9904=PLANE ( 'NONE',  #14935 ) ;
#9905=CARTESIAN_POINT ( 'NONE',  ( 1.767766952966369320, 185.5999999978150754, 5.232233047033630235 ) ) ;
#9910=CARTESIAN_POINT ( 'NONE',  ( -1.767766952966369542, 185.2699999975965568, 8.767766952966368876 ) ) ;
#9911=CARTESIAN_POINT ( 'NONE',  ( -1.385362557672197736, 227.7924883072852822, 5.640085252515396164 ) ) ;
#9913=CARTESIAN_POINT ( 'NONE',  ( 2.807343268925317492, 227.6302376672054208, 8.330365510804844220 ) ) ;
#9914=CARTESIAN_POINT ( 'NONE',  ( -0.07717340183324516989, 189.6978550888158850, 10.38866401756452262 ) ) ;
#9921=CARTESIAN_POINT ( 'NONE',  ( 2.771580177427784619, 226.9203070754519729, 6.240395558440384960 ) ) ;
#9928=CARTESIAN_POINT ( 'NONE',  ( 1.767766952966369098, 187.2300000002184959, 5.232233047033630235 ) ) ;
#9930=CARTESIAN_POINT ( 'NONE',  ( 1.360905158423219241, 228.7363411735375962, 8.365986164091459898 ) ) ;
#9934=CARTESIAN_POINT ( 'NONE',  ( -2.066987300000001859, 188.6999999989075150, 7.856174172912944620 ) ) ;
#9935=CARTESIAN_POINT ( 'NONE',  ( 2.500000000000000444, 187.0999999978150754, 7.000000000000000000 ) ) ;
#9936=CARTESIAN_POINT ( 'NONE',  ( 2.066987300000000083, 186.0499999989075093, 7.000000000000000000 ) ) ;
#9938=AXIS2_PLACEMENT_3D ( 'NONE', #10951, #10873, #12640 ) ;
#9941=B_SPLINE_CURVE_WITH_KNOTS ( 'NONE', 3,
 ( #13216, #8377, #10672, #881, #11778, #7259, #13050, #15689, #10591, #10827, #4554, #12970, #2309, #4791, #4711, #2229, #15530, #5905, #14238, #9323, #15453, #12096, #13128, #15610 ),
 .UNSPECIFIED., .F., .F.,
 ( 4, 2, 2, 2, 2, 2, 2, 2, 2, 2, 2, 4 ),
 ( 0.000000000000000000, 0.06249999999999945877, 0.1249999999999989175, 0.1562499999999986400, 0.1874999999999983902, 0.2499999999999993339, 0.3125000000000002776, 0.3437500000000007216, 0.3750000000000011657, 0.4375000000000006661, 0.4687500000000003331, 0.5000000000000000000 ),
 .UNSPECIFIED. ) ;
#9948=CARTESIAN_POINT ( 'NONE',  ( 2.656575965584776711, 189.9553606806719017, 5.797866007794856280 ) ) ;
#9954=CARTESIAN_POINT ( 'NONE',  ( -5.421010862427522170E-16, 186.6499999989075320, 9.066987300000000971 ) ) ;
#9963=CARTESIAN_POINT ( 'NONE',  ( -1.126573280235289021, 228.1844602338491370, 9.960491586248465978 ) ) ;
#9972=CARTESIAN_POINT ( 'NONE',  ( -2.051698115976866355, 227.9946287341323057, 9.402281653761695779 ) ) ;
#9975=ORIENTED_EDGE ( 'NONE', *, *, #9136, .F. ) ;
#9977=CARTESIAN_POINT ( 'NONE',  ( 0.9656511469083723931, 188.9999999999999716, 4.686691486504618531 ) ) ;
#9984=CARTESIAN_POINT ( 'NONE',  ( -1.767766952966369765, 187.5999999978150754, 8.767766952966368876 ) ) ;
#9989=CARTESIAN_POINT ( 'NONE',  ( 2.500000000000000444, 185.6199999975965795, 5.964466094067262247 ) ) ;
#9990=CARTESIAN_POINT ( 'NONE',  ( 0.5489208960863538600, 227.6341400683239726, 5.182766506802777506 ) ) ;
#9991=CARTESIAN_POINT ( 'NONE',  ( -2.257704606524308488, 227.9260547655458140, 9.200601119324863575 ) ) ;
#9993=CARTESIAN_POINT ( 'NONE',  ( -2.877165451417496023, 189.2399726852219715, 8.034986858290199763 ) ) ;
#10001=CARTESIAN_POINT ( 'NONE',  ( 1.974191107854609495, 228.0195094073193331, 9.475456042165514958 ) ) ;
#10008=CARTESIAN_POINT ( 'NONE',  ( -2.500000000000000444, 186.8499999999999943, 8.035533905932737753 ) ) ;
#10010=CARTESIAN_POINT ( 'NONE',  ( -1.212146835196386663, 227.7435586823976337, 5.498773705076675178 ) ) ;
#10014=CARTESIAN_POINT ( 'NONE',  ( 1.767766952966369320, 184.0999999999999943, 5.232233047033630235 ) ) ;
#10016=CARTESIAN_POINT ( 'NONE',  ( 1.461580736456472351, 187.5499999989075093, 8.461580736456474128 ) ) ;
#10023=CARTESIAN_POINT ( 'NONE',  ( 2.174074109817228706, 188.9999999993558504, 5.753087114337779973 ) ) ;
#10025=CARTESIAN_POINT ( 'NONE',  ( 1.840960705394127928, 189.7476812664443742, 9.752039420742224962 ) ) ;
#10029=CARTESIAN_POINT ( 'NONE',  ( -0.6508408531687689402, 189.0000000000000000, 4.580680803288122327 ) ) ;
#10031=CARTESIAN_POINT ( 'NONE',  ( 1.461580736456472795, 186.9499999989075150, 5.538419263543527649 ) ) ;
#10041=CARTESIAN_POINT ( 'NONE',  ( -1.991442181821953650, 228.0119299072603383, 9.453167579138481713 ) ) ;
#10061=CARTESIAN_POINT ( 'NONE',  ( -2.500000000000000444, 187.4999999978150527, 7.000000000000000000 ) ) ;
#10062=CARTESIAN_POINT ( 'NONE',  ( -2.500000000000000444, 185.9499999978150413, 8.035533905932737753 ) ) ;
#10067=CARTESIAN_POINT ( 'NONE',  ( 1.035533905932737753, 187.3199999975965966, 4.500000000000000888 ) ) ;
#10068=CARTESIAN_POINT ( 'NONE',  ( -1.938951794131667850, 228.1124887269953092, 6.564264716264994526 ) ) ;
#10069=CARTESIAN_POINT ( 'NONE',  ( -2.052299789776659722, 226.5858468330626465, 5.255005641065958244 ) ) ;
#10070=CARTESIAN_POINT ( 'NONE',  ( -0.7435873775819946685, 188.9999999999307931, 9.391030955749405607 ) ) ;
#10076=CARTESIAN_POINT ( 'NONE',  ( 2.814970402829801710, 226.9540368158492925, 6.339744779883301540 ) ) ;
#10081=( BOUNDED_CURVE ( )  B_SPLINE_CURVE ( 2, ( #5741, #11697, #10662, #4704, #3414, #8125, #15682, #6938, #2302 ),
 .UNSPECIFIED., .F., .F. ) 
 B_SPLINE_CURVE_WITH_KNOTS ( ( 3, 2, 2, 2, 3 ),
 ( 0.7142857142857143016, 0.7321428571428570953, 0.7500000000000000000, 0.7678571428571429047, 0.7678695020645334157 ),
 .UNSPECIFIED. ) 
 CURVE ( )  GEOMETRIC_REPRESENTATION_ITEM ( )  RATIONAL_B_SPLINE_CURVE ( ( 1.000000000000000000, 0.9238795325112867385, 1.000000000000000000, 0.9238795325112867385, 1.000000000000000000, 0.9238795325112867385, 1.000000000000000000, 0.9999473158359161173, 0.9998947045988972882 ) ) 
 REPRESENTATION_ITEM ( '' )  );
#10082=CARTESIAN_POINT ( 'NONE',  ( 1.767766952966368432, 187.0999999999999943, 8.767766952966368876 ) ) ;
#10085=CARTESIAN_POINT ( 'NONE',  ( -1.132970084112051579, 227.7246690377758398, 5.444219334014433365 ) ) ;
#10086=CARTESIAN_POINT ( 'NONE',  ( -1.965116437629976787E-16, 189.2499999989075263, 4.933012699999999029 ) ) ;
#10089=CARTESIAN_POINT ( 'NONE',  ( 2.066987299999999639, 188.1999999989075150, 7.856174172912946396 ) ) ;
#10091=CARTESIAN_POINT ( 'NONE',  ( -0.8561741729129456191, 187.8999999989075320, 4.933012699999999029 ) ) ;
#10094=EDGE_CURVE ( 'NONE', #13484, #3329, #14963, .T. ) ;
#10096=CARTESIAN_POINT ( 'NONE',  ( 0.000000000000000000, 201.6409668649146738, 13.30942870683726298 ) ) ;
#10100=CARTESIAN_POINT ( 'NONE',  ( 2.328196544915174027, 189.0000000006442065, 6.072157968082956714 ) ) ;
#10104=CARTESIAN_POINT ( 'NONE',  ( 2.500000000000000444, 184.3499999989075206, 7.000000000000000000 ) ) ;
#10107=CARTESIAN_POINT ( 'NONE',  ( 0.8561741729129455081, 186.1999999989075150, 4.933012699999999029 ) ) ;
#10119=CARTESIAN_POINT ( 'NONE',  ( -0.4746045441281580013, 189.7004852670901585, 10.35781894787841573 ) ) ;
#10141=CARTESIAN_POINT ( 'NONE',  ( -2.500000000000000444, 185.8999999978150584, 7.000000000000000000 ) ) ;
#10146=CARTESIAN_POINT ( 'NONE',  ( -6.911788849595090767E-16, 187.7699999975965568, 9.500000000000001776 ) ) ;
#10147=CARTESIAN_POINT ( 'NONE',  ( 0.8239120926223584274, 228.2181226988968774, 10.05946334177977519 ) ) ;
#10148=CARTESIAN_POINT ( 'NONE',  ( -2.733336431741188566, 227.6877042401139022, 8.499448515046434949 ) ) ;
#10150=CARTESIAN_POINT ( 'NONE',  ( -0.6060429735925918493, 188.9999999999195950, 9.429439317718889768 ) ) ;
#10157=CARTESIAN_POINT ( 'NONE',  ( 2.998004403696063580, 227.2514993113943547, 7.215655842644150830 ) ) ;
#10162=CARTESIAN_POINT ( 'NONE',  ( -1.767766952966369542, 185.2999999999999829, 8.767766952966368876 ) ) ;
#10163=CARTESIAN_POINT ( 'NONE',  ( -1.814481855529834764, 227.9916279875985765, 6.215212007442850961 ) ) ;
#10167=CARTESIAN_POINT ( 'NONE',  ( 1.767766952966369320, 184.9000000000000057, 5.232233047033630235 ) ) ;
#10169=CARTESIAN_POINT ( 'NONE',  ( -2.066987300000000527, 187.9999999989075263, 6.143825827087054492 ) ) ;
#10175=( BOUNDED_CURVE ( )  B_SPLINE_CURVE ( 2, ( #9935, #14787, #11200, #13578, #9065, #3003, #845, #6908, #4508 ),
 .UNSPECIFIED., .F., .F. ) 
 B_SPLINE_CURVE_WITH_KNOTS ( ( 3, 2, 2, 2, 3 ),
 ( 0.4285714285714285476, 0.4464285714285714524, 0.4642857142857143016, 0.4821428571428571508, 0.5000000000000000000 ),
 .UNSPECIFIED. ) 
 CURVE ( )  GEOMETRIC_REPRESENTATION_ITEM ( )  RATIONAL_B_SPLINE_CURVE ( ( 1.000000000000000000, 0.9238795325112867385, 1.000000000000000000, 0.9238795325112867385, 1.000000000000000000, 0.9238795325112867385, 1.000000000000000000, 0.9238795325112867385, 1.000000000000000000 ) ) 
 REPRESENTATION_ITEM ( '' )  );
#10177=CARTESIAN_POINT ( 'NONE',  ( 2.435767896792930376, 189.0000000021955202, 7.586867367984001298 ) ) ;
#10179=CARTESIAN_POINT ( 'NONE',  ( -2.913793338554793166E-15, 228.9118723800512782, 8.872930300147347182 ) ) ;
#10184=CARTESIAN_POINT ( 'NONE',  ( -2.066987300000000083, 186.4499999989075150, 7.000000000000000000 ) ) ;
#10216=CARTESIAN_POINT ( 'NONE',  ( -5.387129544537350156E-16, 185.2999999978150356, 9.500000000000001776 ) ) ;
#10222=CARTESIAN_POINT ( 'NONE',  ( 2.500000000000000444, 185.5699999975965397, 7.000000000000000000 ) ) ;
#10223=CARTESIAN_POINT ( 'NONE',  ( -0.9967757174687167376, 228.8247258804818216, 8.621246238880397428 ) ) ;
#10224=CARTESIAN_POINT ( 'NONE',  ( -0.7768053109583262783, 226.3575155338836282, 4.581995736916623763 ) ) ;
#10234=CARTESIAN_POINT ( 'NONE',  ( 0.1881727879509562662, 228.2551366909677597, 10.16828399086544721 ) ) ;
#10240=CARTESIAN_POINT ( 'NONE',  ( 1.035533905932737753, 186.5499999999999829, 4.500000000000000888 ) ) ;
#10241=CARTESIAN_POINT ( 'NONE',  ( 0.7033144145436343031, 227.6506181221223244, 5.230356066017792571 ) ) ;
#10247=CARTESIAN_POINT ( 'NONE',  ( -0.8561741729129458411, 188.4999999989074979, 4.933012699999999029 ) ) ;
#10249=CARTESIAN_POINT ( 'NONE',  ( -1.461580736456473462, 186.5499999989075093, 8.461580736456472351 ) ) ;
#10253=CARTESIAN_POINT ( 'NONE',  ( -5.999999999999999112, 201.6409668649147022, 13.30942870683726120 ) ) ;
#10255=CARTESIAN_POINT ( 'NONE',  ( 2.572874078457004998, 189.3734677023459199, 5.473824851193815455 ) ) ;
#10258=CARTESIAN_POINT ( 'NONE',  ( 0.9770418472818584998, 189.7111507403969881, 10.22957020356571967 ) ) ;
#10262=CARTESIAN_POINT ( 'NONE',  ( -2.066987300000000971, 186.4999999989075263, 7.856174172912944620 ) ) ;
#10286=CARTESIAN_POINT ( 'NONE',  ( 3.659182332138577465E-16, 195.9933836657089898, 6.233275261299416670 ) ) ;
#10293=CARTESIAN_POINT ( 'NONE',  ( 2.500000000000000000, 188.6999999978150697, 7.000000000000000000 ) ) ;
#10295=CARTESIAN_POINT ( 'NONE',  ( -5.385276659965230388E-16, 226.3251816629291966, 4.486670979098442480 ) ) ;
#10299=CARTESIAN_POINT ( 'NONE',  ( -2.500000000000000444, 188.3199999975965682, 5.964466094067261359 ) ) ;
#10300=CARTESIAN_POINT ( 'NONE',  ( 2.438651006298347301, 227.8520175407923034, 8.982830694042164055 ) ) ;
#10301=CARTESIAN_POINT ( 'NONE',  ( -0.9181233697252281223, 226.3712865412501003, 4.622592831843514993 ) ) ;
#10315=CARTESIAN_POINT ( 'NONE',  ( -2.500000000000000444, 185.0499999978150640, 5.964466094067261359 ) ) ;
#10316=CARTESIAN_POINT ( 'NONE',  ( 0.06504883222449296676, 227.6089665442046339, 5.110063933342379627 ) ) ;
#10321=PRODUCT_DEFINITION ( 'UNKNOWN', '', #13643, #4189 ) ;
#10322=CARTESIAN_POINT ( 'NONE',  ( -2.500000000000000444, 186.0000000000000000, 7.000000000000000000 ) ) ;
#10323=LINE ( 'NONE', #9139, #5312 ) ;
#10325=CARTESIAN_POINT ( 'NONE',  ( 2.066987299999999639, 187.5999999989075491, 7.856174172912946396 ) ) ;
#10331=CARTESIAN_POINT ( 'NONE',  ( 2.082142646712863421, 190.0100437745609554, 5.053690205712503491 ) ) ;
#10332=CARTESIAN_POINT ( 'NONE',  ( 2.500000000000000444, 187.8999999978150584, 7.000000000000000000 ) ) ;
#10334=CARTESIAN_POINT ( 'NONE',  ( 1.986575337946455022, 228.3035988107396292, 7.116201538324070874 ) ) ;
#10339=CARTESIAN_POINT ( 'NONE',  ( -1.461580736456473462, 188.9499999989075150, 8.461580736456472351 ) ) ;
#10343=CARTESIAN_POINT ( 'NONE',  ( 4.404571325722361763E-17, 185.7999999999999829, 4.500000000000000000 ) ) ;
#10351=CARTESIAN_POINT ( 'NONE',  ( -5.999999999999999112, 187.9952603975225429, 3.440894205938198613 ) ) ;
#10352=CARTESIAN_POINT ( 'NONE',  ( 2.500000000000000444, 187.0999999978150754, 7.000000000000000000 ) ) ;
#10369=CARTESIAN_POINT ( 'NONE',  ( 2.066987299999999639, 185.1999999989075150, 7.856174172912946396 ) ) ;
#10375=CARTESIAN_POINT ( 'NONE',  ( 2.500000000000000444, 188.0199999975965852, 5.964466094067262247 ) ) ;
#10376=CARTESIAN_POINT ( 'NONE',  ( 2.467000123265670641, 227.8390626820829823, 8.944723654098295285 ) ) ;
#10394=CARTESIAN_POINT ( 'NONE',  ( 2.500000000000000000, 188.7500000000000000, 8.035533905932739529 ) ) ;
#10396=CARTESIAN_POINT ( 'NONE',  ( 1.767766952966368654, 186.1999999978150697, 8.767766952966368876 ) ) ;
#10397=CARTESIAN_POINT ( 'NONE',  ( -1.361424426418679889, 228.7361946629245892, 8.365563033085530620 ) ) ;
#10401=CARTESIAN_POINT ( 'NONE',  ( -2.500000000000000444, 185.9500000000000455, 5.964466094067261359 ) ) ;
#10403=CARTESIAN_POINT ( 'NONE',  ( -2.066760391300492827E-16, 189.4499999989075150, 4.933012699999999029 ) ) ;
#10407=CARTESIAN_POINT ( 'NONE',  ( 2.500000000000000444, 186.4000000000000057, 7.000000000000000000 ) ) ;
#10410=MECHANICAL_DESIGN_GEOMETRIC_PRESENTATION_REPRESENTATION('',(#14459),#7602);
#10411=CARTESIAN_POINT ( 'NONE',  ( 0.9656511489911946411, 189.0000000017439845, 4.686691485181459171 ) ) ;
#10414=CARTESIAN_POINT ( 'NONE',  ( 1.989910900261709470, 228.2393533748197569, 6.930657055068108363 ) ) ;
#10419=CARTESIAN_POINT ( 'NONE',  ( 2.066987300000000083, 184.9999999989074979, 7.856174172912946396 ) ) ;
#10426=CARTESIAN_POINT ( 'NONE',  ( 1.461580736456473018, 184.5499999989075093, 5.538419263543527649 ) ) ;
#10433=CARTESIAN_POINT ( 'NONE',  ( 5.999999999999999112, 195.9172377311516016, 6.220370292208427188 ) ) ;
#10447=CARTESIAN_POINT ( 'NONE',  ( -0.8561741729129455081, 185.4999999989075548, 4.933012699999999029 ) ) ;
#10454=CARTESIAN_POINT ( 'NONE',  ( -1.058356156152139738, 226.3870070917984094, 4.668936284651906909 ) ) ;
#10455=MANIFOLD_SOLID_BREP ( 'Thread1', #15128 ) ;
#10471=CARTESIAN_POINT ( 'NONE',  ( -1.767766952966369765, 187.7000000000000171, 8.767766952966368876 ) ) ;
#10473=CARTESIAN_POINT ( 'NONE',  ( -1.312946155259101522, 228.7505583286450985, 8.407046118935697976 ) ) ;
#10479=CARTESIAN_POINT ( 'NONE',  ( -1.767766952966369765, 187.7000000000000171, 8.767766952966368876 ) ) ;
#10487=CARTESIAN_POINT ( 'NONE',  ( -2.433389886697037152, 189.7888483223419200, 9.123136959575992577 ) ) ;
#10492=CARTESIAN_POINT ( 'NONE',  ( 0.4194150275617615775, 228.8973402254239033, 8.830960608724256033 ) ) ;
#10497=CARTESIAN_POINT ( 'NONE',  ( -2.066987300000000527, 185.4499999989075150, 7.000000000000000000 ) ) ;
#10502=CARTESIAN_POINT ( 'NONE',  ( -0.8561741729129466183, 184.9999999989074979, 9.066987299999999195 ) ) ;
#10504=CARTESIAN_POINT ( 'NONE',  ( -2.066987300000000527, 186.2499999989074979, 7.000000000000000000 ) ) ;
#10509=CARTESIAN_POINT ( 'NONE',  ( 0.000000000000000000, 222.0378120216257400, 12.20449933502084505 ) ) ;
#10525=CARTESIAN_POINT ( 'NONE',  ( -1.767766952966369320, 188.1999999978150697, 5.232233047033630235 ) ) ;
#10531=CARTESIAN_POINT ( 'NONE',  ( 2.789580270747262780, 227.6450226773988845, 8.373868502673408543 ) ) ;
#10532=CARTESIAN_POINT ( 'NONE',  ( -0.6829126361173057935, 228.2303005364134094, 10.09526665386122346 ) ) ;
#10539=ORIENTED_EDGE ( 'NONE', *, *, #1079, .T. ) ;
#10547=CARTESIAN_POINT ( 'NONE',  ( -1.767766952966369320, 188.2999999999999829, 5.232233047033630235 ) ) ;
#10548=CARTESIAN_POINT ( 'NONE',  ( -2.710505431213761085E-17, 228.2551366889530016, 10.16828399152529983 ) ) ;
#10551=CARTESIAN_POINT ( 'NONE',  ( -1.524659305057740610E-16, 189.0000000000000000, 4.500000000000000000 ) ) ;
#10553=CARTESIAN_POINT ( 'NONE',  ( -1.035533905932739751, 186.1500000000000057, 9.500000000000003553 ) ) ;
#10560=DIRECTION ( 'NONE',  ( 1.000000000000000000, 0.000000000000000000, 0.000000000000000000 ) ) ;
#10561=CARTESIAN_POINT ( 'NONE',  ( -2.500000000000000444, 184.0000000000000000, 7.000000000000000000 ) ) ;
#10562=DIRECTION ( 'NONE',  ( -6.123233995736766036E-17, 1.000000000000000000, 0.000000000000000000 ) ) ;
#10563=FACE_OUTER_BOUND ( 'NONE', #7156, .T. ) ;
#10565=CARTESIAN_POINT ( 'NONE',  ( 1.974531203966234827, 228.3459296953993203, 7.238455547615789243 ) ) ;
#10570=CARTESIAN_POINT ( 'NONE',  ( 2.066987300000000527, 184.2499999989074979, 7.000000000000000000 ) ) ;
#10576=CARTESIAN_POINT ( 'NONE',  ( 3.726944967918921492E-17, 185.4499999989075150, 4.933012699999999029 ) ) ;
#10578=CARTESIAN_POINT ( 'NONE',  ( 1.461580736456473462, 185.1499999989075320, 5.538419263543526760 ) ) ;
#10582=CARTESIAN_POINT ( 'NONE',  ( -5.999999999999999112, 188.6555110544239824, 3.692234042171783415 ) ) ;
#10586=ORIENTED_EDGE ( 'NONE', *, *, #15632, .F. ) ;
#10591=CARTESIAN_POINT ( 'NONE',  ( 1.788462153556203305, 228.5496497207740845, 7.826810600328078849 ) ) ;
#10594=( BOUNDED_SURFACE ( )  B_SPLINE_SURFACE ( 1, 2, ( 
 ( #11245, #9034, #7667, #269, #7745, #347, #13625, #11326, #504, #15068, #3843, #2972, #10216, #1689, #6566, #4001, #2738, #14834, #9905, #5132, #6413, #2818, #12438, #5211, #10141, #10062, #5294, #12356, #2658, #7823, #4084, #12515, #14759, #14993, #7590, #11401, #3919, #422, #14910, #8878, #1614, #8716, #1538, #5371, #4164, #6490, #13860, #578, #13710, #1770, #12672, #6644, #11474, #8955, #6331, #13549, #12591, #13786, #9984, #7512, #1453, #11168, #9181, #9408, #5754, #11856, #3050, #3353, #15379, #8219, #10525, #5447, #4475, #14172, #11633, #9329, #9257, #12901, #13939, #1924, #10293, #13055, #7901, #15147, #15301, #733, #5677, #10598, #4241, #6877, #811, #1845, #3126, #12743, #7979, #3277, #15459, #4321, #8141, #9110, #6720 ),
 ( #11784, #12976, #8060, #2079, #11553, #14020, #2154, #14244, #6952, #7028, #2002, #649, #5522, #886, #11710, #10369, #15220, #4560, #12820, #6797, #5601, #10447, #4403, #14092, #3202, #10918, #3747, #6074, #7418, #16, #9735, #7187, #4878, #4799, #8465, #9489, #13221, #967, #8623, #14320, #10678, #10833, #12025, #1201, #1281, #15538, #2396, #12101, #13136, #7105, #13458, #9567, #5990, #9810, #2482, #2315, #14573, #14659, #3670, #13299, #4635, #4959, #15615, #10757, #3514, #8383, #7264, #5833, #3428, #11942, #6155, #8547, #2235, #8298, #7341, #4717, #13372, #12183, #2561, #1048, #10994, #14409, #1125, #15695, #5911, #9653, #91, #14494, #3591, #5272, #2718, #251, #13688, #2875, #1671, #6234, #5351, #12572, #4063, #8933, #6392 ) ),
 .UNSPECIFIED., .F., .F., .F. ) 
 B_SPLINE_SURFACE_WITH_KNOTS ( ( 2, 2 ),
 ( 3, 2, 2, 2, 2, 2, 2, 2, 2, 2, 2, 2, 2, 2, 2, 2, 2, 2, 2, 2, 2, 2, 2, 2, 2, 2, 2, 2, 2, 2, 2, 2, 2, 2, 2, 2, 2, 2, 2, 2, 2, 2, 2, 2, 2, 2, 2, 2, 2, 2, 3 ),
 ( 0.000000000000000000, 1.000000000000000000 ),
 ( 0.000000000000000000, 0.01785714285714285615, 0.03571428571428571230, 0.05357142857142856845, 0.07142857142857142461, 0.08928571428571428770, 0.1071428571428571369, 0.1250000000000000000, 0.1428571428571428492, 0.1607142857142857262, 0.1785714285714285754, 0.1964285714285714246, 0.2142857142857142738, 0.2321428571428571508, 0.2500000000000000000, 0.2678571428571428492, 0.2857142857142856984, 0.3035714285714285476, 0.3214285714285714524, 0.3392857142857143016, 0.3571428571428571508, 0.3750000000000000000, 0.3928571428571428492, 0.4107142857142856984, 0.4285714285714285476, 0.4464285714285714524, 0.4642857142857143016, 0.4821428571428571508, 0.5000000000000000000, 0.5178571428571429047, 0.5357142857142856984, 0.5535714285714286031, 0.5714285714285713969, 0.5892857142857143016, 0.6071428571428570953, 0.6250000000000000000, 0.6428571428571429047, 0.6607142857142856984, 0.6785714285714286031, 0.6964285714285713969, 0.7142857142857143016, 0.7321428571428570953, 0.7500000000000000000, 0.7678571428571429047, 0.7857142857142856984, 0.8035714285714286031, 0.8214285714285713969, 0.8392857142857143016, 0.8571428571428570953, 0.8750000000000000000, 0.8928571428571429047 ),
 .UNSPECIFIED. ) 
 GEOMETRIC_REPRESENTATION_ITEM ( )  RATIONAL_B_SPLINE_SURFACE ( (
 ( 1.000000000000000000, 0.9238795325112867385, 1.000000000000000000, 0.9238795325112867385, 1.000000000000000000, 0.9238795325112867385, 1.000000000000000000, 0.9238795325112867385, 1.000000000000000000, 0.9238795325112867385, 1.000000000000000000, 0.9238795325112867385, 1.000000000000000000, 0.9238795325112867385, 1.000000000000000000, 0.9238795325112867385, 1.000000000000000000, 0.9238795325112867385, 1.000000000000000000, 0.9238795325112867385, 1.000000000000000000, 0.9238795325112867385, 1.000000000000000000, 0.9238795325112867385, 1.000000000000000000, 0.9238795325112867385, 1.000000000000000000, 0.9238795325112867385, 1.000000000000000000, 0.9238795325112867385, 1.000000000000000000, 0.9238795325112867385, 1.000000000000000000, 0.9238795325112867385, 1.000000000000000000, 0.9238795325112867385, 1.000000000000000000, 0.9238795325112867385, 1.000000000000000000, 0.9238795325112867385, 1.000000000000000000, 0.9238795325112867385, 1.000000000000000000, 0.9238795325112867385, 1.000000000000000000, 0.9238795325112867385, 1.000000000000000000, 0.9238795325112867385, 1.000000000000000000, 0.9238795325112867385, 1.000000000000000000, 0.9238795325112867385, 1.000000000000000000, 0.9238795325112867385, 1.000000000000000000, 0.9238795325112867385, 1.000000000000000000, 0.9238795325112867385, 1.000000000000000000, 0.9238795325112867385, 1.000000000000000000, 0.9238795325112867385, 1.000000000000000000, 0.9238795325112867385, 1.000000000000000000, 0.9238795325112867385, 1.000000000000000000, 0.9238795325112867385, 1.000000000000000000, 0.9238795325112867385, 1.000000000000000000, 0.9238795325112867385, 1.000000000000000000, 0.9238795325112867385, 1.000000000000000000, 0.9238795325112867385, 1.000000000000000000, 0.9238795325112867385, 1.000000000000000000, 0.9238795325112867385, 1.000000000000000000, 0.9238795325112867385, 1.000000000000000000, 0.9238795325112867385, 1.000000000000000000, 0.9238795325112867385, 1.000000000000000000, 0.9238795325112867385, 1.000000000000000000, 0.9238795325112867385, 1.000000000000000000, 0.9238795325112867385, 1.000000000000000000, 0.9238795325112867385, 1.000000000000000000, 0.9238795325112867385, 1.000000000000000000, 0.9238795325112867385, 1.000000000000000000, 0.9238795325112867385, 1.000000000000000000),
 ( 1.000000000000000000, 0.9238795325112867385, 1.000000000000000000, 0.9238795325112867385, 1.000000000000000000, 0.9238795325112867385, 1.000000000000000000, 0.9238795325112867385, 1.000000000000000000, 0.9238795325112867385, 1.000000000000000000, 0.9238795325112867385, 1.000000000000000000, 0.9238795325112867385, 1.000000000000000000, 0.9238795325112867385, 1.000000000000000000, 0.9238795325112867385, 1.000000000000000000, 0.9238795325112867385, 1.000000000000000000, 0.9238795325112867385, 1.000000000000000000, 0.9238795325112867385, 1.000000000000000000, 0.9238795325112867385, 1.000000000000000000, 0.9238795325112867385, 1.000000000000000000, 0.9238795325112867385, 1.000000000000000000, 0.9238795325112867385, 1.000000000000000000, 0.9238795325112867385, 1.000000000000000000, 0.9238795325112867385, 1.000000000000000000, 0.9238795325112867385, 1.000000000000000000, 0.9238795325112867385, 1.000000000000000000, 0.9238795325112867385, 1.000000000000000000, 0.9238795325112867385, 1.000000000000000000, 0.9238795325112867385, 1.000000000000000000, 0.9238795325112867385, 1.000000000000000000, 0.9238795325112867385, 1.000000000000000000, 0.9238795325112867385, 1.000000000000000000, 0.9238795325112867385, 1.000000000000000000, 0.9238795325112867385, 1.000000000000000000, 0.9238795325112867385, 1.000000000000000000, 0.9238795325112867385, 1.000000000000000000, 0.9238795325112867385, 1.000000000000000000, 0.9238795325112867385, 1.000000000000000000, 0.9238795325112867385, 1.000000000000000000, 0.9238795325112867385, 1.000000000000000000, 0.9238795325112867385, 1.000000000000000000, 0.9238795325112867385, 1.000000000000000000, 0.9238795325112867385, 1.000000000000000000, 0.9238795325112867385, 1.000000000000000000, 0.9238795325112867385, 1.000000000000000000, 0.9238795325112867385, 1.000000000000000000, 0.9238795325112867385, 1.000000000000000000, 0.9238795325112867385, 1.000000000000000000, 0.9238795325112867385, 1.000000000000000000, 0.9238795325112867385, 1.000000000000000000, 0.9238795325112867385, 1.000000000000000000, 0.9238795325112867385, 1.000000000000000000, 0.9238795325112867385, 1.000000000000000000, 0.9238795325112867385, 1.000000000000000000, 0.9238795325112867385, 1.000000000000000000, 0.9238795325112867385, 1.000000000000000000) ) ) 
 REPRESENTATION_ITEM ( '' )  SURFACE ( )  );
#10598=CARTESIAN_POINT ( 'NONE',  ( -2.500000000000000444, 189.0499999978150356, 5.964466094067261359 ) ) ;
#10604=CARTESIAN_POINT ( 'NONE',  ( 2.500000000000000444, 187.9699999975965738, 7.000000000000000000 ) ) ;
#10605=CARTESIAN_POINT ( 'NONE',  ( 2.733135974173155791, 227.6887743597950760, 8.502598298417593625 ) ) ;
#10609=CARTESIAN_POINT ( 'NONE',  ( -1.767766952966369542, 185.9999999978150527, 8.767766952966368876 ) ) ;
#10627=CARTESIAN_POINT ( 'NONE',  ( -2.500000000000000444, 188.3499999999999943, 5.964466094067261359 ) ) ;
#10629=CARTESIAN_POINT ( 'NONE',  ( 0.6320692372082544752, 228.2335842258707430, 10.10492066627648988 ) ) ;
#10632=CARTESIAN_POINT ( 'NONE',  ( 1.767766952966368432, 188.7000000000000171, 8.767766952966368876 ) ) ;
#10639=CARTESIAN_POINT ( 'NONE',  ( -2.585318580472420802, 226.7961291864880877, 5.874574987694232142 ) ) ;
#10641=CARTESIAN_POINT ( 'NONE',  ( 2.500000000000000444, 183.9300000002185129, 7.000000000000000000 ) ) ;
#10643=CARTESIAN_POINT ( 'NONE',  ( 1.884974866327016940, 228.4701649684375866, 7.597254102066775872 ) ) ;
#10648=CARTESIAN_POINT ( 'NONE',  ( 2.066987300000000527, 187.4499999989075150, 7.000000000000000000 ) ) ;
#10652=CARTESIAN_POINT ( 'NONE',  ( 1.767766952966368432, 186.2999999999999829, 8.767766952966368876 ) ) ;
#10657=CARTESIAN_POINT ( 'NONE',  ( 2.066987300000000527, 185.0999999989075206, 6.143825827087054492 ) ) ;
#10661=CARTESIAN_POINT ( 'NONE',  ( 5.999999999999999112, 201.6409668649147022, 13.30942870683726120 ) ) ;
#10662=CARTESIAN_POINT ( 'NONE',  ( 1.767766952966369098, 188.7999999978150356, 5.232233047033630235 ) ) ;
#10672=CARTESIAN_POINT ( 'NONE',  ( 0.5202723921993107625, 228.8949738520769586, 8.824126387528728799 ) ) ;
#10678=CARTESIAN_POINT ( 'NONE',  ( -2.066987300000000083, 186.4499999989075150, 7.000000000000000000 ) ) ;
#10680=( BOUNDED_CURVE ( )  B_SPLINE_CURVE ( 2, ( #728, #4399, #9253, #14087, #12894, #6332, #710, #11169, #3920 ),
 .UNSPECIFIED., .F., .F. ) 
 B_SPLINE_CURVE_WITH_KNOTS ( ( 3, 2, 2, 2, 3 ),
 ( 0.1428571428571428492, 0.1607142857142857539, 0.1785714285714286031, 0.1964285714285714524, 0.2142857142857143293 ),
 .UNSPECIFIED. ) 
 CURVE ( )  GEOMETRIC_REPRESENTATION_ITEM ( )  RATIONAL_B_SPLINE_CURVE ( ( 1.000000000000000000, 0.9238795325112867385, 1.000000000000000000, 0.9238795325112867385, 1.000000000000000000, 0.9238795325112867385, 1.000000000000000000, 0.9238795325112865164, 1.000000000000000222 ) ) 
 REPRESENTATION_ITEM ( '' )  );
#10685=CARTESIAN_POINT ( 'NONE',  ( 1.980782313704909203, 226.5644727820218520, 5.192016377768971402 ) ) ;
#10688=CARTESIAN_POINT ( 'NONE',  ( 1.035533905932738419, 186.1499999978150584, 9.500000000000000000 ) ) ;
#10705=CARTESIAN_POINT ( 'NONE',  ( -1.035533905932737975, 186.5499999978150640, 4.500000000000000888 ) ) ;
#10706=CARTESIAN_POINT ( 'NONE',  ( 1.583222688839772019, 228.1098062731747689, 9.740983991995673108 ) ) ;
#10708=CARTESIAN_POINT ( 'NONE',  ( -1.398763622202980894, 189.4255937783873094, 4.329173634885357558 ) ) ;
#10720=CARTESIAN_POINT ( 'NONE',  ( -2.999416585479811381, 227.3092116331243631, 7.385563965123170149 ) ) ;
#10722=CARTESIAN_POINT ( 'NONE',  ( 1.767766952966369320, 185.6300000002185016, 5.232233047033630235 ) ) ;
#10723=CARTESIAN_POINT ( 'NONE',  ( -0.0007128680628333008105, 227.6089742637946642, 5.110086227958842819 ) ) ;
#10724=CARTESIAN_POINT ( 'NONE',  ( 0.9965032137571403492, 227.6963699622695287, 5.362489989878645780 ) ) ;
#10731=CARTESIAN_POINT ( 'NONE',  ( 2.066987300000000971, 185.8999999989075036, 6.143825827087054492 ) ) ;
#10738=CARTESIAN_POINT ( 'NONE',  ( 0.000000000000000000, 186.0499999989075093, 4.933012699999999029 ) ) ;
#10742=CARTESIAN_POINT ( 'NONE',  ( 0.07162589071487505954, 189.0001276426230561, 4.501026264287848910 ) ) ;
#10744=CARTESIAN_POINT ( 'NONE',  ( 1.767766952966368654, 185.3999999978150584, 8.767766952966368876 ) ) ;
#10754=EDGE_CURVE ( 'NONE', #12097, #15371, #8467, .T. ) ;
#10757=CARTESIAN_POINT ( 'NONE',  ( 2.066987299999999639, 187.5999999989075491, 7.856174172912946396 ) ) ;
#10758=VECTOR ( 'NONE', #1113, 1000.000000000000000 ) ;
#10765=CARTESIAN_POINT ( 'NONE',  ( 0.1966278158245924057, 226.3267328078643459, 4.491244098638222937 ) ) ;
#10769=CARTESIAN_POINT ( 'NONE',  ( -2.500000000000001776, 188.3499999978150470, 8.035533905932737753 ) ) ;
#10770=VERTEX_POINT ( 'NONE', #10295 ) ;
#10783=CARTESIAN_POINT ( 'NONE',  ( -2.500000000000000444, 186.7499999978150242, 8.035533905932737753 ) ) ;
#10784=CARTESIAN_POINT ( 'NONE',  ( 2.975657739721877970, 227.4162173224905530, 7.700537803285528504 ) ) ;
#10792=CARTESIAN_POINT ( 'NONE',  ( 2.682774040342114308, 226.8574465069323765, 6.055224137038854870 ) ) ;
#10796=CARTESIAN_POINT ( 'NONE',  ( -2.891600564906900317, 227.0306417089624347, 6.565254640817405729 ) ) ;
#10799=CARTESIAN_POINT ( 'NONE',  ( -1.767766952966369320, 188.2300000002184959, 5.232233047033630235 ) ) ;
#10801=CARTESIAN_POINT ( 'NONE',  ( -1.288813234857717038, 227.7638191499166851, 5.557287090853593625 ) ) ;
#10807=CARTESIAN_POINT ( 'NONE',  ( -1.461580736456473240, 188.5499999989075093, 5.538419263543526760 ) ) ;
#10808=CARTESIAN_POINT ( 'NONE',  ( 0.8561741729129457301, 186.7999999989074809, 4.933012699999999029 ) ) ;
#10816=CARTESIAN_POINT ( 'NONE',  ( -0.8561741729129470624, 187.9999999989075263, 9.066987300000000971 ) ) ;
#10818=CARTESIAN_POINT ( 'NONE',  ( 0.6408967059908734498, 188.9999999999627391, 9.420550830048384228 ) ) ;
#10825=ORIENTED_EDGE ( 'NONE', *, *, #923, .F. ) ;
#10827=CARTESIAN_POINT ( 'NONE',  ( 1.938790558398429731, 228.4312510197253800, 7.484868398679935808 ) ) ;
#10833=CARTESIAN_POINT ( 'NONE',  ( -2.066987300000000971, 186.4999999989075263, 7.856174172912944620 ) ) ;
#10839=CARTESIAN_POINT ( 'NONE',  ( -2.842542329930219491, 227.5997332721124451, 8.240608773874100734 ) ) ;
#10843=CARTESIAN_POINT ( 'NONE',  ( -1.767766952966369765, 188.3999999978150584, 8.767766952966368876 ) ) ;
#10859=CARTESIAN_POINT ( 'NONE',  ( -1.767766952966369765, 188.3999999978150584, 8.767766952966368876 ) ) ;
#10860=CARTESIAN_POINT ( 'NONE',  ( 0.1966278158245924057, 226.3267328078643459, 4.491244098638222937 ) ) ;
#10864=AXIS2_PLACEMENT_3D ( 'NONE', #13370, #7416, #7490 ) ;
#10865=ADVANCED_FACE ( 'NONE', ( #1497 ), #3569, .T. ) ;
#10866=CARTESIAN_POINT ( 'NONE',  ( -0.8324916443616545703, 189.0000000018762307, 4.635459683989287427 ) ) ;
#10870=DIRECTION ( 'NONE',  ( -6.123233995736766036E-17, 1.000000000000000000, 0.000000000000000000 ) ) ;
#10873=DIRECTION ( 'NONE',  ( 0.000000000000000000, 0.9449569463142380998, -0.3271946967975951637 ) ) ;
#10879=CARTESIAN_POINT ( 'NONE',  ( -0.001074311305641557088, 226.3251817249170017, 4.486671161788877704 ) ) ;
#10882=CARTESIAN_POINT ( 'NONE',  ( 1.767766952966369098, 188.8300000002184902, 5.232233047033630235 ) ) ;
#10884=CARTESIAN_POINT ( 'NONE',  ( 1.940097806574041073, 228.1129668193434838, 6.565645474235799917 ) ) ;
#10886=B_SPLINE_CURVE_WITH_KNOTS ( 'NONE', 1,
 ( #11656, #8164 ),
 .UNSPECIFIED., .F., .F.,
 ( 2, 2 ),
 ( 0.000000000000000000, 1.000000000000000000 ),
 .UNSPECIFIED. ) ;
#10889=CARTESIAN_POINT ( 'NONE',  ( 0.8561741729129456191, 188.3999999989075036, 4.933012699999999029 ) ) ;
#10891=CARTESIAN_POINT ( 'NONE',  ( -0.8561741729129471734, 187.1999999989075434, 9.066987300000000971 ) ) ;
#10899=CARTESIAN_POINT ( 'NONE',  ( -1.461580736456473906, 188.7499999989075263, 8.461580736456474128 ) ) ;
#10902=CARTESIAN_POINT ( 'NONE',  ( 1.038438449965593646, 189.0000000004559979, 9.278652163284620613 ) ) ;
#10911=EDGE_CURVE ( 'NONE', #3363, #7505, #6248, .T. ) ;
#10913=VERTEX_POINT ( 'NONE', #8183 ) ;
#10918=CARTESIAN_POINT ( 'NONE',  ( -2.066987300000000971, 185.6999999989075434, 7.856174172912944620 ) ) ;
#10922=CARTESIAN_POINT ( 'NONE',  ( -2.932912173331216898, 227.0860177055994882, 6.728427774621575708 ) ) ;
#10941=CARTESIAN_POINT ( 'NONE',  ( -2.500000000000000888, 188.2999999978150356, 7.000000000000000000 ) ) ;
#10942=CARTESIAN_POINT ( 'NONE',  ( 2.999966428792078865, 227.3061007205240571, 7.376404775963534277 ) ) ;
#10944=CARTESIAN_POINT ( 'NONE',  ( -2.088929602433466037, 189.4018337869057405, 4.846696350498261197 ) ) ;
#10948=CARTESIAN_POINT ( 'NONE',  ( 1.035533905932738197, 187.8500000000000227, 9.500000000000000000 ) ) ;
#10951=CARTESIAN_POINT ( 'NONE',  ( 0.000000000000000000, 228.2633636156256216, 6.999999999969752196 ) ) ;
#10957=CARTESIAN_POINT ( 'NONE',  ( 1.767766952966369098, 188.0300000002185072, 5.232233047033630235 ) ) ;
#10960=CARTESIAN_POINT ( 'NONE',  ( 1.452733574390970395, 228.7063250495755540, 8.279297886081021574 ) ) ;
#10965=CARTESIAN_POINT ( 'NONE',  ( 1.461580736456473240, 189.1499999989075036, 5.538419263543526760 ) ) ;
#10966=CARTESIAN_POINT ( 'NONE',  ( -2.066987300000000971, 186.9999999989074979, 6.143825827087054492 ) ) ;
#10971=CARTESIAN_POINT ( 'NONE',  ( -2.500000000000000444, 184.0000000000000000, 7.000000000000000000 ) ) ;
#10974=CARTESIAN_POINT ( 'NONE',  ( -0.8561741729129458411, 188.4999999989075263, 4.933012699999999029 ) ) ;
#10976=CARTESIAN_POINT ( 'NONE',  ( -0.07135113763453347635, 189.0441085615117345, 10.18309864254113961 ) ) ;
#10988=ORIENTED_EDGE ( 'NONE', *, *, #13811, .T. ) ;
#10993=CARTESIAN_POINT ( 'NONE',  ( -1.768703179866833342, 189.0000639513403939, 5.233169770031948609 ) ) ;
#10994=CARTESIAN_POINT ( 'NONE',  ( 2.066987299999999639, 188.4499999989075150, 7.000000000000000000 ) ) ;
#11000=CIRCLE ( 'NONE', #4135, 1.000000000000000888 ) ;
#11002=CARTESIAN_POINT ( 'NONE',  ( -1.942272232823049061, 226.5542875158922129, 5.161998670295230518 ) ) ;
#11007=CARTESIAN_POINT ( 'NONE',  ( -0.05280746222630467585, 189.0001365486126303, 9.499442212161147481 ) ) ;
#11015=CYLINDRICAL_SURFACE ( 'NONE', #6942, 2.500000000000000444 ) ;
#11017=B_SPLINE_CURVE_WITH_KNOTS ( 'NONE', 3,
 ( #5092, #13584, #537, #4203, #3009 ),
 .UNSPECIFIED., .F., .F.,
 ( 4, 1, 4 ),
 ( 0.009490796809568564224, 0.009530342151606398249, 0.009569887493644234008 ),
 .UNSPECIFIED. ) ;
#11018=CARTESIAN_POINT ( 'NONE',  ( -2.500000000000000888, 189.0999999978150470, 7.000000000000000000 ) ) ;
#11019=CARTESIAN_POINT ( 'NONE',  ( 1.980782313704909203, 226.5644727820218520, 5.192016377768971402 ) ) ;
#11022=CARTESIAN_POINT ( 'NONE',  ( -2.084265404442477987, 189.7627086689134330, 9.536083203068468350 ) ) ;
#11029=CARTESIAN_POINT ( 'NONE',  ( 1.487915498575067774, 226.4497023322808218, 4.853725831513067135 ) ) ;
#11035=CARTESIAN_POINT ( 'NONE',  ( 2.500000000000000444, 186.3800000002185016, 5.964466094067262247 ) ) ;
#11037=CARTESIAN_POINT ( 'NONE',  ( 1.986724198295925836, 228.2179917342068052, 6.868963418589798309 ) ) ;
#11042=CARTESIAN_POINT ( 'NONE',  ( 2.066987300000000083, 185.7999999989075093, 7.856174172912946396 ) ) ;
#11044=CARTESIAN_POINT ( 'NONE',  ( 1.461580736456472573, 185.1499999989075320, 8.461580736456474128 ) ) ;
#11045=ORIENTED_EDGE ( 'NONE', *, *, #210, .T. ) ;
#11046=ADVANCED_FACE ( 'NONE', ( #12147 ), #14699, .T. ) ;
#11050=CARTESIAN_POINT ( 'NONE',  ( 0.000000000000000000, 187.2933328889893687, 9.583808270834989429 ) ) ;
#11051=CARTESIAN_POINT ( 'NONE',  ( -2.273135563902617839, 189.0000000000000568, 8.047421711106334641 ) ) ;
#11063=ORIENTED_EDGE ( 'NONE', *, *, #15629, .F. ) ;
#11078=CARTESIAN_POINT ( 'NONE',  ( -2.994031302066835654, 227.3524127508109132, 7.512731884239616242 ) ) ;
#11096=CARTESIAN_POINT ( 'NONE',  ( -2.500000000000000444, 185.1199999975965511, 5.964466094067261359 ) ) ;
#11097=CARTESIAN_POINT ( 'NONE',  ( -1.580027211161896261, 227.8635840621947182, 5.845413847729996171 ) ) ;
#11098=CARTESIAN_POINT ( 'NONE',  ( 2.990158053860457077, 227.3692281962998436, 7.562228658338257858 ) ) ;
#11099=CARTESIAN_POINT ( 'NONE',  ( -0.07135113763453279634, 189.0441085615118197, 10.18309864254113073 ) ) ;
#11112=CARTESIAN_POINT ( 'NONE',  ( -1.767766952966369320, 186.6300000002185016, 5.232233047033630235 ) ) ;
#11115=CARTESIAN_POINT ( 'NONE',  ( 1.851056454904606685, 228.5003429013454763, 7.684409693542115782 ) ) ;
#11120=CARTESIAN_POINT ( 'NONE',  ( 2.500000000000000444, 185.5999999999999943, 7.000000000000000000 ) ) ;
#11122=CARTESIAN_POINT ( 'NONE',  ( 2.066987299999999639, 185.9999999989074979, 7.856174172912946396 ) ) ;
#11138=CARTESIAN_POINT ( 'NONE',  ( -2.500000000000000444, 187.5499999999999829, 5.964466094067261359 ) ) ;
#11140=CARTESIAN_POINT ( 'NONE',  ( 2.066987299999999639, 187.5999999989075491, 7.856174172912946396 ) ) ;
#11148=CARTESIAN_POINT ( 'NONE',  ( -0.2771997073367608033, 189.6983012903869223, 10.38340820118765961 ) ) ;
#11156=CARTESIAN_POINT ( 'NONE',  ( -2.191791664054325572, 227.9495085101182781, 9.269582106420829248 ) ) ;
#11163=CARTESIAN_POINT ( 'NONE',  ( 2.504072367983524394, 189.0000000000000284, 7.091356059880736140 ) ) ;
#11168=CARTESIAN_POINT ( 'NONE',  ( 1.035533905932738197, 187.7499999978150527, 9.500000000000003553 ) ) ;
#11169=CARTESIAN_POINT ( 'NONE',  ( -2.500000000000003109, 185.1499999999999773, 5.964466094067263136 ) ) ;
#11173=CARTESIAN_POINT ( 'NONE',  ( 2.500000000000000444, 186.3699999975965511, 7.000000000000000000 ) ) ;
#11174=CARTESIAN_POINT ( 'NONE',  ( 0.2606415164794526063, 227.6142277459897230, 5.125258584176975774 ) ) ;
#11175=CARTESIAN_POINT ( 'NONE',  ( -0.6817270424356797198, 226.3498696214933545, 4.559454910794151772 ) ) ;
#11176=CARTESIAN_POINT ( 'NONE',  ( -2.967000931369979000, 189.2639667020261243, 7.657867365370162993 ) ) ;
#11184=CARTESIAN_POINT ( 'NONE',  ( 2.151094780193339773, 227.9624926137814498, 9.307769045389981954 ) ) ;
#11192=CARTESIAN_POINT ( 'NONE',  ( -1.767766952966369320, 186.7000000000000171, 5.232233047033630235 ) ) ;
#11196=EDGE_CURVE ( 'NONE', #15449, #9005, #317, .T. ) ;
#11199=CARTESIAN_POINT ( 'NONE',  ( 1.461580736456473240, 189.1499999989075036, 5.538419263543526760 ) ) ;
#11200=CARTESIAN_POINT ( 'NONE',  ( 1.767766952966369098, 187.1999999978150697, 5.232233047033630235 ) ) ;
#11201=CARTESIAN_POINT ( 'NONE',  ( -2.066987300000000527, 188.8499999989074922, 7.000000000000000000 ) ) ;
#11208=CARTESIAN_POINT ( 'NONE',  ( 2.833833435690741531, 189.2310187018060788, 8.166587331077602485 ) ) ;
#11209=CARTESIAN_POINT ( 'NONE',  ( 1.767766952966369098, 187.9999999978150527, 5.232233047033630235 ) ) ;
#11215=CARTESIAN_POINT ( 'NONE',  ( 2.066987299999999639, 185.9999999989074979, 7.856174172912946396 ) ) ;
#11225=CARTESIAN_POINT ( 'NONE',  ( -1.101860293008299907, 228.1876483704662633, 9.969866227122023972 ) ) ;
#11228=CARTESIAN_POINT ( 'NONE',  ( 0.000000000000000000, 195.7865323290426716, 12.30567995348059007 ) ) ;
#11238=CARTESIAN_POINT ( 'NONE',  ( 2.493490695362371667, 189.0000000000000000, 6.752556055000679791 ) ) ;
#11245=CARTESIAN_POINT ( 'NONE',  ( 2.500000000000000444, 184.6999999978150697, 7.000000000000000000 ) ) ;
#11251=CARTESIAN_POINT ( 'NONE',  ( -5.421010862427522170E-16, 185.3699999975965511, 9.500000000000001776 ) ) ;
#11252=CARTESIAN_POINT ( 'NONE',  ( -1.814481855529834764, 227.9916279875985765, 6.215212007442850961 ) ) ;
#11253=CARTESIAN_POINT ( 'NONE',  ( -2.899241975612990352, 227.5395701600909888, 8.063569561630318461 ) ) ;
#11255=CARTESIAN_POINT ( 'NONE',  ( -1.612690174612901650, 189.7356689584554204, 9.916675524984150059 ) ) ;
#11263=CARTESIAN_POINT ( 'NONE',  ( 2.999303574923353644, 227.2680296707977163, 7.264325765249956213 ) ) ;
#11269=CARTESIAN_POINT ( 'NONE',  ( 9.147955830346443662E-17, 185.0000000000000000, 4.500000000000000000 ) ) ;
#11271=CARTESIAN_POINT ( 'NONE',  ( -1.673363231402341000, 227.9073979391035891, 5.971950823222174520 ) ) ;
#11276=CARTESIAN_POINT ( 'NONE',  ( -2.500000000000000444, 184.4499999999999886, 8.035533905932737753 ) ) ;
#11278=CARTESIAN_POINT ( 'NONE',  ( 2.066987300000000083, 187.6999999989075150, 6.143825827087054492 ) ) ;
#11280=CARTESIAN_POINT ( 'NONE',  ( 2.500000000000000000, 188.0000000000000000, 7.000000000000000000 ) ) ;
#11283=SHAPE_REPRESENTATION ( 'finger', ( #14201 ), #4310 ) ;
#11286=CARTESIAN_POINT ( 'NONE',  ( 2.278945590441513236, 189.0000000008205916, 8.040059661612891873 ) ) ;
#11288=CARTESIAN_POINT ( 'NONE',  ( 0.4782965142628293753, 190.0842368319956961, 4.234201933446612109 ) ) ;
#11291=CARTESIAN_POINT ( 'NONE',  ( -1.537640463591734230, 189.0000000000000284, 5.001843613985847092 ) ) ;
#11293=CARTESIAN_POINT ( 'NONE',  ( -5.895349312889930360E-16, 187.4499999989075150, 9.066987300000000971 ) ) ;
#11300=CARTESIAN_POINT ( 'NONE',  ( 2.500000000000000444, 185.6500000000000057, 5.964466094067262247 ) ) ;
#11304=CARTESIAN_POINT ( 'NONE',  ( -0.8596577831047461649, 189.7079546061267479, 10.26809000054746868 ) ) ;
#11317=CARTESIAN_POINT ( 'NONE',  ( 1.292454556065922411, 189.0000000000001137, 9.144800992884551505 ) ) ;
#11326=CARTESIAN_POINT ( 'NONE',  ( -2.500000000000000444, 185.0499999978150640, 5.964466094067261359 ) ) ;
#11330=CARTESIAN_POINT ( 'NONE',  ( -2.500000000000000444, 187.6199999975965511, 8.035533905932737753 ) ) ;
#11331=CARTESIAN_POINT ( 'NONE',  ( -2.710505431213761085E-17, 228.2551366889530016, 10.16828399152529983 ) ) ;
#11332=CARTESIAN_POINT ( 'NONE',  ( -2.932912173331216898, 227.0860177055994882, 6.728427774621575708 ) ) ;
#11334=CARTESIAN_POINT ( 'NONE',  ( -2.749342815197933554, 189.8200872727807393, 8.555607185862969644 ) ) ;
#11340=CARTESIAN_POINT ( 'NONE',  ( 2.995459646452805380, 227.2354604000217932, 7.168427219998267041 ) ) ;
#11343=CARTESIAN_POINT ( 'NONE',  ( -1.767766952966369765, 188.5000000000000000, 8.767766952966368876 ) ) ;
#11346=CARTESIAN_POINT ( 'NONE',  ( -1.035533905932737975, 186.6500000000000057, 4.500000000000000888 ) ) ;
#11348=CARTESIAN_POINT ( 'NONE',  ( -0.8231351400649619121, 227.6668932001845462, 5.277359419731677548 ) ) ;
#11353=CARTESIAN_POINT ( 'NONE',  ( 2.500000000000000444, 184.8499999999999943, 5.964466094067262247 ) ) ;
#11355=CARTESIAN_POINT ( 'NONE',  ( 1.461580736456472795, 189.3499999989074922, 5.538419263543527649 ) ) ;
#11360=CARTESIAN_POINT ( 'NONE',  ( 3.659182332138577465E-16, 195.9172377311516016, 6.220370292208427188 ) ) ;
#11361=CARTESIAN_POINT ( 'NONE',  ( 2.973431353044737602, 189.8579570988357546, 7.753557815461304514 ) ) ;
#11363=CARTESIAN_POINT ( 'NONE',  ( 0.3969367148316809146, 189.6994987093958684, 10.36945981054583044 ) ) ;
#11368=CARTESIAN_POINT ( 'NONE',  ( -0.8561741729129467293, 186.5999999989075206, 9.066987299999999195 ) ) ;
#11375=CARTESIAN_POINT ( 'NONE',  ( 0.000000000000000000, 184.0000000000000000, 7.000000000000000000 ) ) ;
#11395=CARTESIAN_POINT ( 'NONE',  ( 2.500000000000000000, 188.6999999978150697, 7.000000000000000000 ) ) ;
#11401=CARTESIAN_POINT ( 'NONE',  ( 1.035533905932737975, 186.4499999978150697, 4.500000000000000888 ) ) ;
#11405=CARTESIAN_POINT ( 'NONE',  ( 2.500000000000000444, 187.9199999975965625, 8.035533905932739529 ) ) ;
#11406=CARTESIAN_POINT ( 'NONE',  ( -1.454385272030960907, 228.7057613863525489, 8.277669994545302501 ) ) ;
#11407=CARTESIAN_POINT ( 'NONE',  ( -2.691043998642291157, 227.7164964219492163, 8.584158233643494285 ) ) ;
#11416=CARTESIAN_POINT ( 'NONE',  ( 1.815926964132193566, 228.0606537879605469, 9.596472842544713444 ) ) ;
#11418=SURFACE_SIDE_STYLE ('',( #4341 ) ) ;
#11422=CARTESIAN_POINT ( 'NONE',  ( 1.767766952966369098, 188.8999999999999773, 5.232233047033630235 ) ) ;
#11423=CARTESIAN_POINT ( 'NONE',  ( 1.767766952966368654, 184.7000000000000171, 8.767766952966368876 ) ) ;
#11425=CARTESIAN_POINT ( 'NONE',  ( 1.620240533814224060, 227.8813442971431016, 5.896706419237646379 ) ) ;
#11429=CARTESIAN_POINT ( 'NONE',  ( -1.767766952966369098, 185.0999999999999943, 5.232233047033630235 ) ) ;
#11431=CARTESIAN_POINT ( 'NONE',  ( -6.877907531704918753E-16, 189.0499999989075093, 9.066987300000000971 ) ) ;
#11434=EDGE_CURVE ( 'NONE', #1738, #8762, #10886, .T. ) ;
#11437=CARTESIAN_POINT ( 'NONE',  ( 0.000000000000000000, 194.5935680195190116, 12.11154058223188201 ) ) ;
#11438=CARTESIAN_POINT ( 'NONE',  ( 2.504072369575190748, 189.0000000010835208, 7.091356059128075096 ) ) ;
#11446=CARTESIAN_POINT ( 'NONE',  ( 1.461580736456472351, 188.3499999989074922, 8.461580736456474128 ) ) ;
#11451=CARTESIAN_POINT ( 'NONE',  ( -2.500000000000000444, 186.0000000000000000, 7.000000000000000000 ) ) ;
#11452=B_SPLINE_CURVE_WITH_KNOTS ( 'NONE', 3,
 ( #1995, #10286, #14085, #8053, #6869, #13932 ),
 .UNSPECIFIED., .F., .F.,
 ( 4, 2, 4 ),
 ( 0.05507452630550478678, 0.5261283886372931651, 0.9743590206738933501 ),
 .UNSPECIFIED. ) ;
#11461=CARTESIAN_POINT ( 'NONE',  ( 1.035533905932738197, 187.0499999999999829, 9.500000000000000000 ) ) ;
#11474=CARTESIAN_POINT ( 'NONE',  ( -4.743384504624081899E-17, 187.2999999978150356, 4.500000000000000000 ) ) ;
#11480=CARTESIAN_POINT ( 'NONE',  ( 1.035533905932738197, 188.6199999975965511, 9.500000000000003553 ) ) ;
#11481=CARTESIAN_POINT ( 'NONE',  ( 2.349311747835623354, 227.8901172732836642, 9.094898149752092209 ) ) ;
#11483=CARTESIAN_POINT ( 'NONE',  ( -2.923025936753522291, 227.5090509392885281, 7.973756422523831766 ) ) ;
#11488=CARTESIAN_POINT ( 'NONE',  ( 2.500000000000000000, 189.4499999978150697, 8.035533905932739529 ) ) ;
#11498=CARTESIAN_POINT ( 'NONE',  ( 2.500000000000000444, 185.6500000000000341, 5.964466094067262247 ) ) ;
#11499=CARTESIAN_POINT ( 'NONE',  ( 1.725625307041983136, 227.9349420198840903, 6.051499699527947307 ) ) ;
#11505=CARTESIAN_POINT ( 'NONE',  ( -6.911788849595090767E-16, 187.7999999999999829, 9.500000000000001776 ) ) ;
#11507=CARTESIAN_POINT ( 'NONE',  ( -0.8561741729129469514, 187.3999999989075889, 9.066987299999999195 ) ) ;
#11513=DIRECTION ( 'NONE',  ( 0.000000000000000000, 0.000000000000000000, 1.000000000000000000 ) ) ;
#11514=CARTESIAN_POINT ( 'NONE',  ( 2.046085423705328310, 189.0000000012578028, 8.444739455527990657 ) ) ;
#11517=CARTESIAN_POINT ( 'NONE',  ( 1.964981070171530675, 228.3669111765908895, 7.299051262003229290 ) ) ;
#11522=CARTESIAN_POINT ( 'NONE',  ( -2.066987300000000971, 186.1999999989075150, 6.143825827087054492 ) ) ;
#11534=CARTESIAN_POINT ( 'NONE',  ( -0.001074311305641557088, 226.3251817249170017, 4.486671161788877704 ) ) ;
#11535=CARTESIAN_POINT ( 'NONE',  ( 1.767766952966368432, 187.0999999999999943, 8.767766952966368876 ) ) ;
#11537=CARTESIAN_POINT ( 'NONE',  ( -1.767766952966369320, 186.5999999978150754, 5.232233047033630235 ) ) ;
#11553=CARTESIAN_POINT ( 'NONE',  ( 8.809142651444723526E-17, 184.6499999989075320, 4.933012699999999029 ) ) ;
#11558=CARTESIAN_POINT ( 'NONE',  ( 1.767766952966368432, 189.4699999975965738, 8.767766952966368876 ) ) ;
#11559=CARTESIAN_POINT ( 'NONE',  ( 0.6804430692981219275, 228.2300923459994237, 10.09465452691961751 ) ) ;
#11561=ORIENTED_EDGE ( 'NONE', *, *, #9159, .F. ) ;
#11574=CARTESIAN_POINT ( 'NONE',  ( 1.035533905932738197, 188.6499999999999773, 9.500000000000000000 ) ) ;
#11577=CARTESIAN_POINT ( 'NONE',  ( 2.500000000000000444, 186.2999999978150356, 7.000000000000000000 ) ) ;
#11579=CARTESIAN_POINT ( 'NONE',  ( -1.990672364496464342, 228.2390692824501457, 6.929836580100483090 ) ) ;
#11583=CARTESIAN_POINT ( 'NONE',  ( 2.500000000000000000, 188.7999999999999829, 7.000000000000000000 ) ) ;
#11590=CARTESIAN_POINT ( 'NONE',  ( -1.579607963155742922, 189.7340877847497325, 9.937618139430700381 ) ) ;
#11591=CARTESIAN_POINT ( 'NONE',  ( 0.9527618732035531002, 189.4347749068571432, 4.132041495851004775 ) ) ;
#11592=CARTESIAN_POINT ( 'NONE',  ( 2.500000000000000444, 184.6800000002185129, 8.035533905932739529 ) ) ;
#11595=CARTESIAN_POINT ( 'NONE',  ( 1.990661649217015494, 228.2715988311494471, 7.023783772108481038 ) ) ;
#11596=CARTESIAN_POINT ( 'NONE',  ( 2.066987300000000527, 184.2499999989074979, 7.000000000000000000 ) ) ;
#11600=CARTESIAN_POINT ( 'NONE',  ( -4.811147140404425926E-16, 185.6499999989075320, 9.066987300000000971 ) ) ;
#11611=CARTESIAN_POINT ( 'NONE',  ( -1.461580736456473018, 184.5499999989075093, 5.538419263543526760 ) ) ;
#11615=CARTESIAN_POINT ( 'NONE',  ( 5.999999999999999112, 215.0542865858234336, 7.296348638370669271 ) ) ;
#11617=CARTESIAN_POINT ( 'NONE',  ( 2.500000000000000444, 187.1499999999999773, 8.035533905932739529 ) ) ;
#11633=CARTESIAN_POINT ( 'NONE',  ( -1.767766952966369765, 188.3999999978150584, 8.767766952966368876 ) ) ;
#11636=CARTESIAN_POINT ( 'NONE',  ( -2.500000000000000444, 185.8499999978150754, 5.964466094067261359 ) ) ;
#11639=CARTESIAN_POINT ( 'NONE',  ( -0.1300625424525254092, 228.9108363453237303, 8.869938172763147222 ) ) ;
#11642=EDGE_LOOP ( 'NONE', ( #14354, #2883, #1196, #4433, #7095 ) ) ;
#11647=CARTESIAN_POINT ( 'NONE',  ( -1.767766952966369765, 189.1999999978150697, 8.767766952966368876 ) ) ;
#11652=DIRECTION ( 'NONE',  ( -0.8660254037844266062, -0.5000000000000208722, 0.000000000000000000 ) ) ;
#11656=CARTESIAN_POINT ( 'NONE',  ( -0.0007128680628333008105, 227.6089742637946642, 5.110086227958842819 ) ) ;
#11657=CARTESIAN_POINT ( 'NONE',  ( 1.767766952966369098, 188.8999999999999773, 5.232233047033630235 ) ) ;
#11658=CARTESIAN_POINT ( 'NONE',  ( -1.580502612156455822, 228.6570661798589299, 8.137035460797768849 ) ) ;
#11665=CARTESIAN_POINT ( 'NONE',  ( -2.500000000000000888, 187.5999999999999943, 7.000000000000000000 ) ) ;
#11676=DIRECTION ( 'NONE',  ( -1.000000000000000000, 0.000000000000000000, 0.000000000000000000 ) ) ;
#11678=CARTESIAN_POINT ( 'NONE',  ( -1.035533905932737753, 184.9800000002184959, 4.500000000000000888 ) ) ;
#11680=CARTESIAN_POINT ( 'NONE',  ( 1.814481968427068992, 227.9916212483514641, 6.215192544112370321 ) ) ;
#11685=CARTESIAN_POINT ( 'NONE',  ( -4.302927372051845722E-16, 184.8499999989074922, 9.066987300000000971 ) ) ;
#11690=CARTESIAN_POINT ( 'NONE',  ( -1.461580736456473240, 184.9499999989075150, 8.461580736456472351 ) ) ;
#11692=CARTESIAN_POINT ( 'NONE',  ( -4.743384504624081899E-17, 186.8499999989074922, 4.933012699999999029 ) ) ;
#11696=CARTESIAN_POINT ( 'NONE',  ( 5.999999999999999112, 185.8606548077538321, 9.048340948986950849 ) ) ;
#11697=CARTESIAN_POINT ( 'NONE',  ( 2.500000000000000444, 188.7499999978150527, 5.964466094067262247 ) ) ;
#11710=CARTESIAN_POINT ( 'NONE',  ( 1.461580736456472573, 185.1499999989075320, 8.461580736456474128 ) ) ;
#11715=CARTESIAN_POINT ( 'NONE',  ( -2.500000000000000888, 189.1699999975965341, 7.000000000000000000 ) ) ;
#11716=CARTESIAN_POINT ( 'NONE',  ( 2.923059718105053051, 227.5089953743221258, 7.973592892444406388 ) ) ;
#11721=EDGE_CURVE ( 'NONE', #9483, #12468, #823, .T. ) ;
#11734=CARTESIAN_POINT ( 'NONE',  ( -2.500000000000000888, 188.4500000000000171, 8.035533905932737753 ) ) ;
#11736=CARTESIAN_POINT ( 'NONE',  ( -0.9967757174687167376, 228.8247258804818216, 8.621246238880397428 ) ) ;
#11740=CARTESIAN_POINT ( 'NONE',  ( 0.05969309337805784460, 188.9999999999999432, 4.500684243071288115 ) ) ;
#11742=CARTESIAN_POINT ( 'NONE',  ( 1.035533905932738197, 186.2500000000000000, 9.500000000000003553 ) ) ;
#11749=CARTESIAN_POINT ( 'NONE',  ( -2.660650785759065329, 227.7358070380394963, 8.640981985597708359 ) ) ;
#11750=CARTESIAN_POINT ( 'NONE',  ( 0.8841844500102366000, 190.0747139113696846, 4.330645362478406923 ) ) ;
#11751=CARTESIAN_POINT ( 'NONE',  ( 1.767766952966368654, 185.4300000002185129, 8.767766952966368876 ) ) ;
#11753=CARTESIAN_POINT ( 'NONE',  ( 1.692341931978252223, 227.9167330860961442, 5.998911260178718230 ) ) ;
#11758=CARTESIAN_POINT ( 'NONE',  ( 1.461580736456473462, 184.3499999989074922, 5.538419263543526760 ) ) ;
#11762=CARTESIAN_POINT ( 'NONE',  ( 1.035533905932738197, 186.2500000000000000, 9.500000000000000000 ) ) ;
#11763=CARTESIAN_POINT ( 'NONE',  ( -1.461580736456472795, 184.7499999989074979, 5.538419263543527649 ) ) ;
#11765=CARTESIAN_POINT ( 'NONE',  ( 0.8561741729129456191, 187.5999999989074922, 4.933012699999999029 ) ) ;
#11769=CARTESIAN_POINT ( 'NONE',  ( 5.999999999999999112, 187.2933328889893403, 9.583808270834989429 ) ) ;
#11777=CARTESIAN_POINT ( 'NONE',  ( 1.461580736456473018, 184.5499999989075093, 5.538419263543527649 ) ) ;
#11778=CARTESIAN_POINT ( 'NONE',  ( 1.221831151830281126, 228.7817678443040563, 8.497180980233151715 ) ) ;
#11784=CARTESIAN_POINT ( 'NONE',  ( 2.066987300000000083, 184.4499999989075150, 7.000000000000000000 ) ) ;
#11791=CARTESIAN_POINT ( 'NONE',  ( 0.6843230633849453071, 226.3504559366005537, 4.561183366923295068 ) ) ;
#11799=EDGE_LOOP ( 'NONE', ( #15650, #12991, #6128, #2407, #4471, #5224, #1859 ) ) ;
#11807=CARTESIAN_POINT ( 'NONE',  ( 2.500000000000000444, 188.8499999999999659, 5.964466094067262247 ) ) ;
#11809=CARTESIAN_POINT ( 'NONE',  ( -1.973877840180719989, 228.3455757694837303, 7.237433389386023208 ) ) ;
#11811=CARTESIAN_POINT ( 'NONE',  ( -1.929793783875213720, 189.4086015753950960, 4.698290738201920114 ) ) ;
#11812=CARTESIAN_POINT ( 'NONE',  ( 1.767766952966369098, 186.5000000000000000, 5.232233047033630235 ) ) ;
#11818=CARTESIAN_POINT ( 'NONE',  ( -2.990970242699510173, 227.3667325949381564, 7.554906020068777650 ) ) ;
#11820=CARTESIAN_POINT ( 'NONE',  ( 0.2560036892252900986, 189.0000000000580371, 4.506310952893917587 ) ) ;
#11821=CARTESIAN_POINT ( 'NONE',  ( -2.500000000000000444, 185.9300000002185129, 7.000000000000000000 ) ) ;
#11824=CARTESIAN_POINT ( 'NONE',  ( 1.989829716803914739, 228.2822890550965553, 7.054657748597916722 ) ) ;
#11829=CARTESIAN_POINT ( 'NONE',  ( 2.066987300000000971, 185.8999999989075036, 6.143825827087054492 ) ) ;
#11830=CARTESIAN_POINT ( 'NONE',  ( -2.500000000000000444, 184.4000000000000057, 7.000000000000000000 ) ) ;
#11837=CARTESIAN_POINT ( 'NONE',  ( 2.066987299999999639, 188.1999999989075150, 7.856174172912946396 ) ) ;
#11840=DIRECTION ( 'NONE',  ( 6.123233995736603333E-17, -1.000000000000000000, 3.749399456655569780E-33 ) ) ;
#11841=CARTESIAN_POINT ( 'NONE',  ( 5.999999999999999112, 194.5935680195190116, 12.11154058223188379 ) ) ;
#11845=ORIENTED_EDGE ( 'NONE', *, *, #13677, .T. ) ;
#11846=EDGE_LOOP ( 'NONE', ( #14311, #15547, #9704, #4398 ) ) ;
#11851=EDGE_CURVE ( 'NONE', #14331, #7444, #10081, .T. ) ;
#11856=CARTESIAN_POINT ( 'NONE',  ( 2.500000000000000444, 187.9499999978150697, 5.964466094067262247 ) ) ;
#11864=CARTESIAN_POINT ( 'NONE',  ( 2.993808330938719564, 227.3535049858431591, 7.515946948957763496 ) ) ;
#11870=EDGE_LOOP ( 'NONE', ( #7002, #9084, #14964, #5415 ) ) ;
#11874=CARTESIAN_POINT ( 'NONE',  ( 1.035533905932738419, 185.4500000000000171, 9.500000000000000000 ) ) ;
#11885=CARTESIAN_POINT ( 'NONE',  ( 9.825582188149883933E-17, 184.8999999978150584, 4.500000000000000000 ) ) ;
#11887=CARTESIAN_POINT ( 'NONE',  ( 1.326034168411047265, 228.1562120337857777, 9.877435289762864556 ) ) ;
#11889=CARTESIAN_POINT ( 'NONE',  ( -1.482782158083479018, 190.0495907483965823, 4.595143857422339551 ) ) ;
#11895=ORIENTED_EDGE ( 'NONE', *, *, #1627, .T. ) ;
#11902=CARTESIAN_POINT ( 'NONE',  ( -2.148870826313457716, 226.6164604241740506, 5.345220325073331225 ) ) ;
#11904=CARTESIAN_POINT ( 'NONE',  ( -1.767766952966369098, 184.2300000002184959, 5.232233047033630235 ) ) ;
#11905=CARTESIAN_POINT ( 'NONE',  ( -0.5214357632711458246, 228.8948738370037290, 8.823837538292856664 ) ) ;
#11906=CARTESIAN_POINT ( 'NONE',  ( -0.9962072163307928996, 227.6960174938032537, 5.361472040843871412 ) ) ;
#11912=CARTESIAN_POINT ( 'NONE',  ( -1.461580736456473240, 187.7499999989075263, 5.538419263543526760 ) ) ;
#11919=CARTESIAN_POINT ( 'NONE',  ( 0.8561741729129456191, 184.5999999989075206, 4.933012699999999029 ) ) ;
#11922=CARTESIAN_POINT ( 'NONE',  ( -5.285485590866834116E-16, 186.4499999989075150, 9.066987300000000971 ) ) ;
#11927=CARTESIAN_POINT ( 'NONE',  ( 0.000000000000000000, 215.3885876087883275, 13.29602556813378733 ) ) ;
#11928=CARTESIAN_POINT ( 'NONE',  ( -1.767766952966369542, 185.1999999978150697, 8.767766952966368876 ) ) ;
#11935=CARTESIAN_POINT ( 'NONE',  ( -1.461580736456472795, 185.5499999989075093, 5.538419263543527649 ) ) ;
#11942=CARTESIAN_POINT ( 'NONE',  ( -0.8561741729129456191, 187.8999999989075320, 4.933012699999999029 ) ) ;
#11949=CARTESIAN_POINT ( 'NONE',  ( 2.550395957922052759, 226.7806086135062458, 5.828878098564913124 ) ) ;
#11969=CARTESIAN_POINT ( 'NONE',  ( 2.500000000000000000, 188.6499999978150584, 8.035533905932739529 ) ) ;
#11970=CARTESIAN_POINT ( 'NONE',  ( 2.994032664863047533, 227.2266946368854690, 7.142638454998203379 ) ) ;
#11972=CARTESIAN_POINT ( 'NONE',  ( -0.6578658431935565654, 189.0000000007884466, 4.581181184014819330 ) ) ;
#11977=ORIENTED_EDGE ( 'NONE', *, *, #12988, .T. ) ;
#11980=CARTESIAN_POINT ( 'NONE',  ( 2.583669522491375936, 226.7981340924959852, 5.880482682298685759 ) ) ;
#11984=CARTESIAN_POINT ( 'NONE',  ( -2.799739712504301092, 226.9429308982220164, 6.307020443959882705 ) ) ;
#11987=CARTESIAN_POINT ( 'NONE',  ( 1.035533905932737753, 186.4800000002185243, 4.500000000000000888 ) ) ;
#11989=CARTESIAN_POINT ( 'NONE',  ( 1.214181464861975757, 227.7437454098885041, 5.499312984720448938 ) ) ;
#11995=CARTESIAN_POINT ( 'NONE',  ( -1.461580736456473906, 187.1499999989075320, 8.461580736456474128 ) ) ;
#11997=CARTESIAN_POINT ( 'NONE',  ( -2.066987300000000527, 187.0499999989075093, 7.000000000000000000 ) ) ;
#12005=CARTESIAN_POINT ( 'NONE',  ( 0.8561741729129460632, 188.0999999989074922, 9.066987300000000971 ) ) ;
#12014=VERTEX_POINT ( 'NONE', #11596 ) ;
#12015=VECTOR ( 'NONE', #875, 1000.000000000000000 ) ;
#12025=CARTESIAN_POINT ( 'NONE',  ( -1.461580736456473462, 186.5499999989075093, 8.461580736456472351 ) ) ;
#12032=CARTESIAN_POINT ( 'NONE',  ( 1.458867243353906273, 226.4466662005724800, 4.844797864602860216 ) ) ;
#12051=CARTESIAN_POINT ( 'NONE',  ( -1.035533905932739751, 187.6499999978150584, 9.500000000000003553 ) ) ;
#12052=CARTESIAN_POINT ( 'NONE',  ( 0.09803033623910094307, 226.3251703050289336, 4.486637493502143137 ) ) ;
#12057=CARTESIAN_POINT ( 'NONE',  ( -2.940898392866930777E-15, 228.9118723800512498, 8.872930300147352511 ) ) ;
#12066=CARTESIAN_POINT ( 'NONE',  ( -2.947655337591893687, 227.4717885095516863, 7.864163344551670320 ) ) ;
#12068=CARTESIAN_POINT ( 'NONE',  ( 2.500000000000000444, 187.1800000002184845, 5.964466094067262247 ) ) ;
#12071=CARTESIAN_POINT ( 'NONE',  ( -0.5154556838971166011, 227.6308307018634025, 5.173208867712369319 ) ) ;
#12072=CARTESIAN_POINT ( 'NONE',  ( 1.050562149602352946, 228.8138732705275231, 8.589903282340008772 ) ) ;
#12076=CARTESIAN_POINT ( 'NONE',  ( -2.066987300000001415, 187.0999999989075206, 7.856174172912944620 ) ) ;
#12077=CARTESIAN_POINT ( 'NONE',  ( 2.066987300000000527, 185.8499999989074922, 7.000000000000000000 ) ) ;
#12084=CARTESIAN_POINT ( 'NONE',  ( -2.321326423937577488, 189.0000000000000000, 7.936319443449496802 ) ) ;
#12086=CARTESIAN_POINT ( 'NONE',  ( 0.9085682364751954676, 189.0000000000368345, 9.333306381950002617 ) ) ;
#12093=EDGE_LOOP ( 'NONE', ( #1684, #14206, #11845, #13308 ) ) ;
#12096=CARTESIAN_POINT ( 'NONE',  ( 0.2612504972992927277, 227.6131741670932342, 5.122215788231598843 ) ) ;
#12097=VERTEX_POINT ( 'NONE', #7153 ) ;
#12101=CARTESIAN_POINT ( 'NONE',  ( 2.066987299999999639, 186.7999999989074809, 7.856174172912946396 ) ) ;
#12107=CARTESIAN_POINT ( 'NONE',  ( -2.976076845141470972, 227.1639356932526539, 6.957862568523350610 ) ) ;
#12112=CARTESIAN_POINT ( 'NONE',  ( 1.767766952966368432, 188.5999999978150470, 8.767766952966368876 ) ) ;
#12123=CARTESIAN_POINT ( 'NONE',  ( -1.965116437629976787E-16, 189.6999999978150697, 4.500000000000000000 ) ) ;
#12126=CARTESIAN_POINT ( 'NONE',  ( -1.035533905932737975, 188.2500000000000000, 4.500000000000001776 ) ) ;
#12129=CARTESIAN_POINT ( 'NONE',  ( 1.035533905932737753, 188.8499999978150470, 4.500000000000000888 ) ) ;
#12131=CARTESIAN_POINT ( 'NONE',  ( 2.733135974173155791, 227.6887743597950760, 8.502598298417593625 ) ) ;
#12134=CARTESIAN_POINT ( 'NONE',  ( -1.585779675826979984, 189.4204380473234721, 4.440511949549013515 ) ) ;
#12147=FACE_OUTER_BOUND ( 'NONE', #12093, .T. ) ;
#12148=CARTESIAN_POINT ( 'NONE',  ( 1.767766952966369098, 186.4300000002185129, 5.232233047033630235 ) ) ;
#12150=CARTESIAN_POINT ( 'NONE',  ( 1.990661649217015494, 228.2715988311494471, 7.023783772108481038 ) ) ;
#12154=CARTESIAN_POINT ( 'NONE',  ( -2.066987300000001415, 188.5999999989074922, 6.143825827087054492 ) ) ;
#12156=CARTESIAN_POINT ( 'NONE',  ( 0.000000000000000000, 186.0499999989075093, 4.933012699999999029 ) ) ;
#12163=CARTESIAN_POINT ( 'NONE',  ( 0.000000000000000000, 222.7460571280668091, 12.08513476933103625 ) ) ;
#12164=CARTESIAN_POINT ( 'NONE',  ( 2.066987300000000083, 189.0999999989075206, 6.143825827087054492 ) ) ;
#12173=CARTESIAN_POINT ( 'NONE',  ( -5.421010862427522170E-17, 187.4000000000000057, 4.500000000000000000 ) ) ;
#12183=CARTESIAN_POINT ( 'NONE',  ( 0.8561741729129458411, 188.2999999989075093, 9.066987299999999195 ) ) ;
#12188=CARTESIAN_POINT ( 'NONE',  ( 0.000000000000000000, 184.0000000000000000, 7.000000000000000000 ) ) ;
#12189=CARTESIAN_POINT ( 'NONE',  ( -2.898051746902431614, 227.0396595591786308, 6.591911377507474690 ) ) ;
#12195=CARTESIAN_POINT ( 'NONE',  ( 1.038438454217461615, 189.0000000000000284, 9.278652157609089457 ) ) ;
#12200=CARTESIAN_POINT ( 'NONE',  ( -2.500000000000000444, 184.0000000000000000, 7.000000000000000000 ) ) ;
#12205=FACE_OUTER_BOUND ( 'NONE', #104, .T. ) ;
#12207=CARTESIAN_POINT ( 'NONE',  ( -1.767766952966369765, 189.1999999978150697, 8.767766952966368876 ) ) ;
#12208=CARTESIAN_POINT ( 'NONE',  ( 2.438651006298347301, 227.8520175407923034, 8.982830694042164055 ) ) ;
#12210=ADVANCED_FACE ( 'NONE', ( #4763 ), #14378, .T. ) ;
#12211=CARTESIAN_POINT ( 'NONE',  ( -2.928701478272802472, 189.8468539625636424, 7.998593929295510385 ) ) ;
#12217=CARTESIAN_POINT ( 'NONE',  ( 0.1880867857842616064, 226.3251816858397092, 4.486670972203318009 ) ) ;
#12222=DIRECTION ( 'NONE',  ( -6.123233995736766036E-17, 1.000000000000000000, 0.000000000000000000 ) ) ;
#12223=CARTESIAN_POINT ( 'NONE',  ( 1.423015351387224570E-16, 184.1999999999999886, 4.500000000000000000 ) ) ;
#12226=CARTESIAN_POINT ( 'NONE',  ( 0.4194150275617615775, 228.8973402254239033, 8.830960608724256033 ) ) ;
#12231=CARTESIAN_POINT ( 'NONE',  ( -0.8561741729129458411, 187.6999999989075150, 4.933012699999999029 ) ) ;
#12233=CARTESIAN_POINT ( 'NONE',  ( -2.066987300000000083, 184.8499999989075206, 7.000000000000000000 ) ) ;
#12240=CARTESIAN_POINT ( 'NONE',  ( -2.402303367210822049, 189.0000000000000284, 7.702985774066552160 ) ) ;
#12251=VERTEX_POINT ( 'NONE', #14101 ) ;
#12268=CARTESIAN_POINT ( 'NONE',  ( -2.668764612700158079, 227.7307401636093687, 8.626063590916809076 ) ) ;
#12269=ORIENTED_EDGE ( 'NONE', *, *, #4732, .F. ) ;
#12282=DIRECTION ( 'NONE',  ( -0.02708880405685116718, 0.000000000000000000, 0.9996330310142664821 ) ) ;
#12284=CARTESIAN_POINT ( 'NONE',  ( -2.500000000000000444, 189.0499999978150356, 5.964466094067261359 ) ) ;
#12285=CARTESIAN_POINT ( 'NONE',  ( 2.809728313654571430, 226.9499418402095046, 6.327683296853605199 ) ) ;
#12287=CARTESIAN_POINT ( 'NONE',  ( -3.003665301663284826, 189.8729084552422535, 7.414818630636749397 ) ) ;
#12293=CARTESIAN_POINT ( 'NONE',  ( 2.104503138662575878, 226.6021308763587285, 5.302993367608996422 ) ) ;
#12299=( BOUNDED_CURVE ( )  B_SPLINE_CURVE ( 2, ( #630, #4300, #15280, #9163, #7960, #12800, #11611, #12876, #1902, #13997, #4382, #6776, #9237, #12357, #1982, #13550, #1454, #10657, #10578, #4537, #14476, #946, #791, #15517, #4616, #8444, #15438, #3253, #8120, #14300, #4456, #8280, #9469, #13114, #15360, #9551, #10738, #2215, #3409, #7085, #10504, #9311, #14389, #1027, #11922, #2379, #13280, #9388, #5813, #4778, #3573, #14226, #11692, #5891, #3493, #15598, #14151, #15677, #12958, #13203, #4699, #8363, #3333, #8201, #5658, #2058, #6934, #11765, #867, #13037, #5734, #2134, #7006, #5972, #2297, #10816, #7167, #12005, #1108, #11837, #9633, #3728, #14554, #9716, #5168, #10974, #13586, #8527, #8754, #2461, #10899, #231, #2697, #2619, #150, #8606, #3808, #12164, #7246, #13356, #13440 ),
 .UNSPECIFIED., .F., .F. ) 
 B_SPLINE_CURVE_WITH_KNOTS ( ( 3, 2, 2, 2, 2, 2, 2, 2, 2, 2, 2, 2, 2, 2, 2, 2, 2, 2, 2, 2, 2, 2, 2, 2, 2, 2, 2, 2, 2, 2, 2, 2, 2, 2, 2, 2, 2, 2, 2, 2, 2, 2, 2, 2, 2, 2, 2, 2, 2, 2, 3 ),
 ( 0.000000000000000000, 0.01785714285714285615, 0.03571428571428571230, 0.05357142857142856845, 0.07142857142857142461, 0.08928571428571428770, 0.1071428571428571369, 0.1250000000000000000, 0.1428571428571428492, 0.1607142857142857262, 0.1785714285714285754, 0.1964285714285714246, 0.2142857142857142738, 0.2321428571428571508, 0.2500000000000000000, 0.2678571428571428492, 0.2857142857142856984, 0.3035714285714285476, 0.3214285714285714524, 0.3392857142857143016, 0.3571428571428571508, 0.3750000000000000000, 0.3928571428571428492, 0.4107142857142856984, 0.4285714285714285476, 0.4464285714285714524, 0.4642857142857143016, 0.4821428571428571508, 0.5000000000000000000, 0.5178571428571429047, 0.5357142857142856984, 0.5535714285714286031, 0.5714285714285713969, 0.5892857142857143016, 0.6071428571428570953, 0.6250000000000000000, 0.6428571428571429047, 0.6607142857142856984, 0.6785714285714286031, 0.6964285714285715079, 0.7142857142857143016, 0.7321428571428570953, 0.7500000000000000000, 0.7678571428571429047, 0.7857142857142856984, 0.8035714285714286031, 0.8214285714285713969, 0.8392857142857143016, 0.8571428571428570953, 0.8750000000000000000, 0.8928571428571429047 ),
 .UNSPECIFIED. ) 
 CURVE ( )  GEOMETRIC_REPRESENTATION_ITEM ( )  RATIONAL_B_SPLINE_CURVE ( ( 1.000000000000000000, 0.9238795325112867385, 1.000000000000000000, 0.9238795325112867385, 1.000000000000000000, 0.9238795325112867385, 1.000000000000000000, 0.9238795325112867385, 1.000000000000000000, 0.9238795325112867385, 1.000000000000000000, 0.9238795325112867385, 1.000000000000000000, 0.9238795325112867385, 1.000000000000000000, 0.9238795325112867385, 1.000000000000000000, 0.9238795325112867385, 1.000000000000000000, 0.9238795325112867385, 1.000000000000000000, 0.9238795325112867385, 1.000000000000000000, 0.9238795325112867385, 1.000000000000000000, 0.9238795325112867385, 1.000000000000000000, 0.9238795325112867385, 1.000000000000000000, 0.9238795325112867385, 1.000000000000000000, 0.9238795325112867385, 1.000000000000000000, 0.9238795325112867385, 1.000000000000000000, 0.9238795325112867385, 1.000000000000000000, 0.9238795325112867385, 1.000000000000000000, 0.9238795325112867385, 1.000000000000000000, 0.9238795325112867385, 1.000000000000000000, 0.9238795325112867385, 1.000000000000000000, 0.9238795325112867385, 1.000000000000000000, 0.9238795325112867385, 1.000000000000000000, 0.9238795325112867385, 1.000000000000000000, 0.9238795325112867385, 1.000000000000000000, 0.9238795325112867385, 1.000000000000000000, 0.9238795325112867385, 1.000000000000000000, 0.9238795325112867385, 1.000000000000000000, 0.9238795325112867385, 1.000000000000000000, 0.9238795325112867385, 1.000000000000000000, 0.9238795325112867385, 1.000000000000000000, 0.9238795325112867385, 1.000000000000000000, 0.9238795325112867385, 1.000000000000000000, 0.9238795325112867385, 1.000000000000000000, 0.9238795325112867385, 1.000000000000000000, 0.9238795325112867385, 1.000000000000000000, 0.9238795325112867385, 1.000000000000000000, 0.9238795325112867385, 1.000000000000000000, 0.9238795325112867385, 1.000000000000000000, 0.9238795325112867385, 1.000000000000000000, 0.9238795325112867385, 1.000000000000000000, 0.9238795325112867385, 1.000000000000000000, 0.9238795325112867385, 1.000000000000000000, 0.9238795325112867385, 1.000000000000000000, 0.9238795325112867385, 1.000000000000000000, 0.9238795325112867385, 1.000000000000000000, 0.9238795325112867385, 1.000000000000000000, 0.9238795325112867385, 1.000000000000000000, 0.9238795325112867385, 1.000000000000000000 ) ) 
 REPRESENTATION_ITEM ( '' )  );
#12300=CARTESIAN_POINT ( 'NONE',  ( -3.388131789017201356E-18, 186.5300000002185072, 4.500000000000000000 ) ) ;
#12307=CARTESIAN_POINT ( 'NONE',  ( -1.461580736456473684, 184.7499999989074979, 8.461580736456474128 ) ) ;
#12310=CARTESIAN_POINT ( 'NONE',  ( 1.461580736456472573, 185.9499999989075150, 8.461580736456474128 ) ) ;
#12318=CARTESIAN_POINT ( 'NONE',  ( 3.659182332138577465E-16, 187.9952603975225713, 3.440894205938198613 ) ) ;
#12319=CARTESIAN_POINT ( 'NONE',  ( -0.2693458344851792918, 189.0000000000000284, 9.494867214852071413 ) ) ;
#12323=CARTESIAN_POINT ( 'NONE',  ( 1.340391840173529081, 189.7235632956260361, 10.07394016998248887 ) ) ;
#12329=CARTESIAN_POINT ( 'NONE',  ( 1.461580736456472795, 187.7499999989075263, 5.538419263543527649 ) ) ;
#12337=CARTESIAN_POINT ( 'NONE',  ( -1.992790919479760392, 190.0169567515527262, 4.969246669617095158 ) ) ;
#12346=CARTESIAN_POINT ( 'NONE',  ( -2.440032737085090275, 227.8520529458832300, 8.982935890751354790 ) ) ;
#12352=CARTESIAN_POINT ( 'NONE',  ( 2.278945589504768776, 189.0000000000000568, 8.040059659319428675 ) ) ;
#12356=CARTESIAN_POINT ( 'NONE',  ( -1.035533905932739529, 186.0499999978150356, 9.500000000000003553 ) ) ;
#12357=CARTESIAN_POINT ( 'NONE',  ( 0.8561741729129461742, 184.8999999989075320, 9.066987300000000971 ) ) ;
#12358=ADVANCED_FACE ( 'NONE', ( #14668 ), #9575, .T. ) ;
#12362=CARTESIAN_POINT ( 'NONE',  ( -2.500000000000000444, 187.5699999975965397, 7.000000000000000000 ) ) ;
#12363=CARTESIAN_POINT ( 'NONE',  ( -1.990672364496464342, 228.2390692824501457, 6.929836580100483090 ) ) ;
#12364=CARTESIAN_POINT ( 'NONE',  ( -2.995192278888715975, 227.2265329420484647, 7.142163989385624134 ) ) ;
#12365=CARTESIAN_POINT ( 'NONE',  ( -2.324167314932467310, 189.0000000021436222, 7.935049049248011244 ) ) ;
#12372=CARTESIAN_POINT ( 'NONE',  ( 2.782695181561366304, 227.6502397201549570, 8.389219295768896245 ) ) ;
#12378=CARTESIAN_POINT ( 'NONE',  ( 1.767766952966368432, 186.2999999999999829, 8.767766952966368876 ) ) ;
#12381=CARTESIAN_POINT ( 'NONE',  ( 0.8212144138252523984, 228.8542370555972809, 8.706476195820313180 ) ) ;
#12385=CARTESIAN_POINT ( 'NONE',  ( -2.066987300000000971, 188.6499999989075036, 7.000000000000000000 ) ) ;
#12388=CARTESIAN_POINT ( 'NONE',  ( -1.461580736456473018, 186.3499999989075206, 5.538419263543527649 ) ) ;
#12402=CARTESIAN_POINT ( 'NONE',  ( 2.500000000000000444, 185.4999999978150527, 7.000000000000000000 ) ) ;
#12406=CARTESIAN_POINT ( 'NONE',  ( 1.461580736456472351, 187.5499999989075093, 8.461580736456474128 ) ) ;
#12410=ORIENTED_EDGE ( 'NONE', *, *, #557, .F. ) ;
#12417=CARTESIAN_POINT ( 'NONE',  ( -2.604939343947620500, 189.9599476955858393, 5.742039956245639232 ) ) ;
#12424=CARTESIAN_POINT ( 'NONE',  ( -2.734462099041327310, 226.8914831935726966, 6.155496219900511434 ) ) ;
#12431=CARTESIAN_POINT ( 'NONE',  ( 0.08806441522324243154, 188.9999999999999716, 9.502418536650717229 ) ) ;
#12433=CARTESIAN_POINT ( 'NONE',  ( 2.500000000000000000, 188.7999999999999829, 7.000000000000000000 ) ) ;
#12438=CARTESIAN_POINT ( 'NONE',  ( -1.767766952966369098, 185.7999999978150356, 5.232233047033630235 ) ) ;
#12443=CARTESIAN_POINT ( 'NONE',  ( 2.500000000000000444, 184.7699999975965568, 7.000000000000000000 ) ) ;
#12444=CARTESIAN_POINT ( 'NONE',  ( 0.4220225674029139951, 227.6236908799334344, 5.152588654748359254 ) ) ;
#12445=CARTESIAN_POINT ( 'NONE',  ( -1.501309217710235622, 226.4539600517547910, 4.866297710963618073 ) ) ;
#12446=CARTESIAN_POINT ( 'NONE',  ( -2.260484549978974744, 188.9999999992296296, 8.078936515875282609 ) ) ;
#12453=CARTESIAN_POINT ( 'NONE',  ( 2.753714765446583446, 226.9066926092818051, 6.200293790039342667 ) ) ;
#12459=CARTESIAN_POINT ( 'NONE',  ( 4.404571325722361763E-17, 185.7999999999999829, 4.500000000000000000 ) ) ;
#12461=CARTESIAN_POINT ( 'NONE',  ( 0.6422548253168780530, 227.6434438162357878, 5.209636261422765813 ) ) ;
#12465=CARTESIAN_POINT ( 'NONE',  ( -1.461580736456473240, 188.5499999989075093, 5.538419263543526760 ) ) ;
#12467=CARTESIAN_POINT ( 'NONE',  ( -6.098637220230962441E-17, 187.0499999989075093, 4.933012699999999029 ) ) ;
#12468=VERTEX_POINT ( 'NONE', #2321 ) ;
#12471=CARTESIAN_POINT ( 'NONE',  ( -6.369687763352338550E-16, 186.8999999978150584, 9.500000000000001776 ) ) ;
#12472=CARTESIAN_POINT ( 'NONE',  ( 3.659182332138577465E-16, 202.3202208672780102, 7.308763624242801349 ) ) ;
#12475=CARTESIAN_POINT ( 'NONE',  ( 2.894817532740828536, 189.8405166879407489, 8.135858506145497770 ) ) ;
#12483=CARTESIAN_POINT ( 'NONE',  ( -2.066987300000000083, 185.5999999989075775, 6.143825827087054492 ) ) ;
#12487=PLANE ( 'NONE',  #13668 ) ;
#12494=CARTESIAN_POINT ( 'NONE',  ( -2.843530175656467041, 189.9274080437028829, 6.285367726569456970 ) ) ;
#12505=ORIENTED_EDGE ( 'NONE', *, *, #15149, .T. ) ;
#12508=CARTESIAN_POINT ( 'NONE',  ( -0.05280746222630467585, 189.0001365486126303, 9.499442212161147481 ) ) ;
#12515=CARTESIAN_POINT ( 'NONE',  ( 2.500000000000000444, 186.2499999978150527, 8.035533905932739529 ) ) ;
#12520=CARTESIAN_POINT ( 'NONE',  ( 2.500000000000000444, 185.5199999975965852, 8.035533905932739529 ) ) ;
#12521=CARTESIAN_POINT ( 'NONE',  ( -1.939606487604890850, 228.4085856529902117, 7.419409526801750587 ) ) ;
#12523=CARTESIAN_POINT ( 'NONE',  ( -2.734462099041327310, 226.8914831935726966, 6.155496219900511434 ) ) ;
#12524=CARTESIAN_POINT ( 'NONE',  ( -1.967390401563962055, 189.1241570952389850, 9.449926551978856892 ) ) ;
#12539=CARTESIAN_POINT ( 'NONE',  ( -2.500000000000000444, 185.9500000000000455, 5.964466094067261359 ) ) ;
#12541=CARTESIAN_POINT ( 'NONE',  ( 0.4540882845019501568, 227.6260587419843091, 5.159427175404782240 ) ) ;
#12546=CARTESIAN_POINT ( 'NONE',  ( -0.8561741729129471734, 187.9999999989075263, 9.066987300000000971 ) ) ;
#12548=CARTESIAN_POINT ( 'NONE',  ( 2.066987299999999639, 189.2499999989075263, 7.000000000000000000 ) ) ;
#12552=CARTESIAN_POINT ( 'NONE',  ( -5.999999999999999112, 202.3202208672780102, 7.308763624254441815 ) ) ;
#12553=ADVANCED_FACE ( 'NONE', ( #14298 ), #9476, .T. ) ;
#12554=CARTESIAN_POINT ( 'NONE',  ( 2.939309742956421889, 189.2553574017071867, 7.797426251816824916 ) ) ;
#12560=CARTESIAN_POINT ( 'NONE',  ( -1.262974410557502258, 189.0000000000000000, 4.817524377743032993 ) ) ;
#12562=CARTESIAN_POINT ( 'NONE',  ( 0.8561741729129452860, 187.7999999989075093, 4.933012699999999029 ) ) ;
#12572=CARTESIAN_POINT ( 'NONE',  ( 2.066987299999999639, 189.2999999989075377, 6.143825827087054492 ) ) ;
#12580=CARTESIAN_POINT ( 'NONE',  ( -2.500000000000000444, 186.6999999978150697, 7.000000000000000000 ) ) ;
#12582=ORIENTED_EDGE ( 'NONE', *, *, #13392, .T. ) ;
#12591=CARTESIAN_POINT ( 'NONE',  ( -2.500000000000000444, 187.4999999978150527, 7.000000000000000000 ) ) ;
#12594=CARTESIAN_POINT ( 'NONE',  ( -1.035533905932739529, 185.3199999975965682, 9.500000000000003553 ) ) ;
#12595=CARTESIAN_POINT ( 'NONE',  ( 1.237590631448066469, 228.1696616696178808, 9.916980740552745033 ) ) ;
#12597=CARTESIAN_POINT ( 'NONE',  ( -2.999982576790682476, 227.2579145021288696, 7.234552515775640735 ) ) ;
#12607=CARTESIAN_POINT ( 'NONE',  ( 0.3830661952130403614, 228.2493291729371094, 10.15124818647456451 ) ) ;
#12615=CARTESIAN_POINT ( 'NONE',  ( -2.500000000000000444, 186.7999999999999829, 7.000000000000000000 ) ) ;
#12616=CARTESIAN_POINT ( 'NONE',  ( -0.5154556838971166011, 227.6308307018634025, 5.173208867712369319 ) ) ;
#12622=CARTESIAN_POINT ( 'NONE',  ( -1.035533905932737753, 185.0499999999999829, 4.500000000000000888 ) ) ;
#12624=CARTESIAN_POINT ( 'NONE',  ( -2.066987300000000527, 188.0499999989075093, 7.000000000000000000 ) ) ;
#12627=CARTESIAN_POINT ( 'NONE',  ( 2.500000000000000444, 187.0499999978150356, 8.035533905932739529 ) ) ;
#12628=AXIS2_PLACEMENT_3D ( 'NONE', #380, #5330, #3956 ) ;
#12629=CARTESIAN_POINT ( 'NONE',  ( 3.659182332138577465E-16, 215.0542865858234336, 7.296348638359030581 ) ) ;
#12630=CARTESIAN_POINT ( 'NONE',  ( 2.493490693894865551, 188.9999999989163655, 6.752556059726261495 ) ) ;
#12633=CARTESIAN_POINT ( 'NONE',  ( 2.451648050241212129, 189.9784261975811717, 5.460752168824765107 ) ) ;
#12639=CARTESIAN_POINT ( 'NONE',  ( -0.8561741729129469514, 188.1999999989075150, 9.066987299999999195 ) ) ;
#12640=DIRECTION ( 'NONE',  ( 0.000000000000000000, 0.3271946967975951637, 0.9449569463142382109 ) ) ;
#12641=EDGE_LOOP ( 'NONE', ( #13907, #14844, #569, #7145 ) ) ;
#12646=CARTESIAN_POINT ( 'NONE',  ( -1.035533905932737975, 185.8500000000000227, 4.500000000000001776 ) ) ;
#12655=AXIS2_PLACEMENT_3D ( 'NONE', #13980, #3390, #10560 ) ;
#12672=CARTESIAN_POINT ( 'NONE',  ( 1.767766952966369098, 187.1999999978150697, 5.232233047033630235 ) ) ;
#12677=CARTESIAN_POINT ( 'NONE',  ( 1.035533905932737753, 189.7199999975965738, 4.500000000000000888 ) ) ;
#12678=CARTESIAN_POINT ( 'NONE',  ( 0.1954887924997270876, 228.2535971796124556, 10.16375797564445804 ) ) ;
#12679=CARTESIAN_POINT ( 'NONE',  ( -1.865818183961493126, 226.5341093703536899, 5.102530190813160615 ) ) ;
#12685=CARTESIAN_POINT ( 'NONE',  ( 1.035533905932737753, 189.6499999978150584, 4.500000000000001776 ) ) ;
#12688=CARTESIAN_POINT ( 'NONE',  ( 2.587737285089668493, 227.7819843651293183, 8.776849827616773680 ) ) ;
#12694=CARTESIAN_POINT ( 'NONE',  ( 1.035533905932738419, 185.4499999999999886, 9.500000000000003553 ) ) ;
#12696=CARTESIAN_POINT ( 'NONE',  ( 1.498060502294345175, 227.8308734224802095, 5.750943654540091821 ) ) ;
#12701=CARTESIAN_POINT ( 'NONE',  ( -2.500000000000000888, 188.3999999999999773, 7.000000000000000000 ) ) ;
#12703=CARTESIAN_POINT ( 'NONE',  ( -2.066987300000000527, 186.4999999989074695, 7.856174172912944620 ) ) ;
#12708=EDGE_CURVE ( 'NONE', #8865, #9005, #1547, .T. ) ;
#12709=CARTESIAN_POINT ( 'NONE',  ( 1.482061430985168737, 189.7295665886300924, 9.997153617204970644 ) ) ;
#12712=CARTESIAN_POINT ( 'NONE',  ( 1.724621985266778568, 228.5864789591000488, 7.933175541215780946 ) ) ;
#12717=CARTESIAN_POINT ( 'NONE',  ( -0.8561741729129470624, 186.3999999989075320, 9.066987300000000971 ) ) ;
#12738=EDGE_LOOP ( 'NONE', ( #4467, #8054, #13762, #981 ) ) ;
#12743=CARTESIAN_POINT ( 'NONE',  ( 1.035533905932738197, 189.3499999978150754, 9.500000000000003553 ) ) ;
#12748=CARTESIAN_POINT ( 'NONE',  ( -0.5160604560792059203, 228.8899596144369752, 8.809644983231040172 ) ) ;
#12756=CARTESIAN_POINT ( 'NONE',  ( 9.825582188149883933E-17, 184.4499999989075150, 4.933012699999999029 ) ) ;
#12761=DIRECTION ( 'NONE',  ( -1.000000000000000000, 0.000000000000000000, 0.000000000000000000 ) ) ;
#12764=CARTESIAN_POINT ( 'NONE',  ( -2.500000000000000444, 185.8499999978150754, 5.964466094067261359 ) ) ;
#12765=ADVANCED_FACE ( 'NONE', ( #9600 ), #15471, .T. ) ;
#12766=CARTESIAN_POINT ( 'NONE',  ( -1.159640499634989608, 227.7308148186401979, 5.461968699681960082 ) ) ;
#12771=CARTESIAN_POINT ( 'NONE',  ( 1.035533905932738197, 187.0499999999999829, 9.500000000000003553 ) ) ;
#12779=CARTESIAN_POINT ( 'NONE',  ( -2.639974099233850957, 189.8080084944625128, 8.785674123968128413 ) ) ;
#12781=CARTESIAN_POINT ( 'NONE',  ( 2.662764147438232865, 189.9529664242985518, 5.851057665551680387 ) ) ;
#12784=CARTESIAN_POINT ( 'NONE',  ( 0.5151998000674417044, 228.8897689535086784, 8.809094343595948118 ) ) ;
#12789=CARTESIAN_POINT ( 'NONE',  ( -0.8561741729129470624, 188.9999999989074979, 9.066987299999999195 ) ) ;
#12794=CARTESIAN_POINT ( 'NONE',  ( 2.500000000000000444, 184.0000000000000000, 7.000000000000000000 ) ) ;
#12796=CARTESIAN_POINT ( 'NONE',  ( -1.767766952966369320, 185.9000000000000057, 5.232233047033630235 ) ) ;
#12798=CARTESIAN_POINT ( 'NONE',  ( -0.8561741729129452860, 184.6999999989075150, 4.933012699999999029 ) ) ;
#12800=CARTESIAN_POINT ( 'NONE',  ( -0.8561741729129456191, 184.4999999989074979, 4.933012699999999029 ) ) ;
#12804=CARTESIAN_POINT ( 'NONE',  ( 0.000000000000000000, 229.2449477060184222, 9.834870838912449287 ) ) ;
#12809=EDGE_LOOP ( 'NONE', ( #3584, #12881, #1939, #14316 ) ) ;
#12820=CARTESIAN_POINT ( 'NONE',  ( 1.461580736456473018, 185.3499999989075206, 5.538419263543527649 ) ) ;
#12826=CARTESIAN_POINT ( 'NONE',  ( -1.923824245924939058, 228.4291822535419954, 7.478893683947804405 ) ) ;
#12838=FACE_OUTER_BOUND ( 'NONE', #4374, .T. ) ;
#12846=CARTESIAN_POINT ( 'NONE',  ( -1.035533905932737753, 184.9499999978150413, 4.500000000000000888 ) ) ;
#12847=CARTESIAN_POINT ( 'NONE',  ( 1.865071889996124055, 228.0459258470066857, 9.553136980667057188 ) ) ;
#12851=CARTESIAN_POINT ( 'NONE',  ( -6.437450399132682577E-16, 187.0000000000000000, 9.500000000000001776 ) ) ;
#12854=EDGE_LOOP ( 'NONE', ( #13106, #5616, #13796, #15311 ) ) ;
#12855=CARTESIAN_POINT ( 'NONE',  ( 2.500000000000000444, 185.4999999978150527, 7.000000000000000000 ) ) ;
#12857=CARTESIAN_POINT ( 'NONE',  ( -2.057242982682720100, 227.9923142528441815, 9.395475597852444238 ) ) ;
#12859=CARTESIAN_POINT ( 'NONE',  ( 1.456896669277396583E-16, 184.1300000002185016, 4.500000000000000000 ) ) ;
#12862=CARTESIAN_POINT ( 'NONE',  ( 1.862843374206504254, 228.4903663355887318, 7.655596802610238782 ) ) ;
#12867=CARTESIAN_POINT ( 'NONE',  ( 1.461580736456473462, 185.9499999989075150, 5.538419263543526760 ) ) ;
#12875=CARTESIAN_POINT ( 'NONE',  ( -2.500000000000000444, 184.0000000000000000, 7.000000000000000000 ) ) ;
#12876=CARTESIAN_POINT ( 'NONE',  ( -2.066987300000000527, 184.5999999989074922, 6.143825827087054492 ) ) ;
#12880=CARTESIAN_POINT ( 'NONE',  ( 0.000000000000000000, 185.8606548077538321, 9.048340948986950849 ) ) ;
#12881=ORIENTED_EDGE ( 'NONE', *, *, #11434, .T. ) ;
#12882=CARTESIAN_POINT ( 'NONE',  ( -2.500000000000000444, 186.8499999999999943, 8.035533905932737753 ) ) ;
#12894=CARTESIAN_POINT ( 'NONE',  ( 9.147955830346443662E-17, 185.0000000000000000, 4.500000000000000000 ) ) ;
#12898=CARTESIAN_POINT ( 'NONE',  ( -1.965116437629976787E-16, 189.2499999989075263, 4.933012699999999029 ) ) ;
#12901=CARTESIAN_POINT ( 'NONE',  ( 1.035533905932738197, 188.5499999978150356, 9.500000000000003553 ) ) ;
#12904=CARTESIAN_POINT ( 'NONE',  ( 1.767766952966369320, 185.5999999978150754, 5.232233047033630235 ) ) ;
#12907=CARTESIAN_POINT ( 'NONE',  ( -1.035533905932739751, 188.5199999975965852, 9.500000000000003553 ) ) ;
#12908=CARTESIAN_POINT ( 'NONE',  ( -1.104351905119298705, 226.3927175376774699, 4.685770134608635118 ) ) ;
#12915=CARTESIAN_POINT ( 'NONE',  ( -1.035533905932739751, 189.2499999978150811, 9.500000000000000000 ) ) ;
#12926=CARTESIAN_POINT ( 'NONE',  ( -1.767766952966369098, 185.7999999978150356, 5.232233047033630235 ) ) ;
#12927=CARTESIAN_POINT ( 'NONE',  ( -1.977913707823687250, 228.3348771801055364, 7.206535253053350409 ) ) ;
#12933=CARTESIAN_POINT ( 'NONE',  ( 1.767766952966369098, 188.0999999999999943, 5.232233047033630235 ) ) ;
#12935=EDGE_CURVE ( 'NONE', #2406, #2326, #6236, .T. ) ;
#12938=CARTESIAN_POINT ( 'NONE',  ( -2.500000000000000444, 184.0000000000000000, 7.000000000000000000 ) ) ;
#12939=CARTESIAN_POINT ( 'NONE',  ( -1.767766952966369320, 186.7000000000000171, 5.232233047033630235 ) ) ;
#12940=CARTESIAN_POINT ( 'NONE',  ( -1.296916486773226129, 226.4196734319506845, 4.765225606315626194 ) ) ;
#12942=CARTESIAN_POINT ( 'NONE',  ( 0.07962153170104048494, 190.0874092006666274, 4.202769577405792489 ) ) ;
#12945=CARTESIAN_POINT ( 'NONE',  ( -1.977662132812563645, 228.3460237620419093, 7.238727217445813267 ) ) ;
#12946=CARTESIAN_POINT ( 'NONE',  ( 1.620240533814224060, 227.8813442971431016, 5.896706419237646379 ) ) ;
#12951=CARTESIAN_POINT ( 'NONE',  ( 0.8561741729129457301, 185.9999999989074979, 4.933012699999999029 ) ) ;
#12957=DIRECTION ( 'NONE',  ( -6.123233995736766036E-17, 1.000000000000000000, 0.000000000000000000 ) ) ;
#12958=CARTESIAN_POINT ( 'NONE',  ( -1.461580736456473906, 187.1499999989075320, 8.461580736456474128 ) ) ;
#12962=CARTESIAN_POINT ( 'NONE',  ( -1.016439536705160407E-17, 228.2551366889529731, 10.16828399152529272 ) ) ;
#12967=ORIENTED_EDGE ( 'NONE', *, *, #488, .F. ) ;
#12969=CARTESIAN_POINT ( 'NONE',  ( 1.461580736456473018, 186.1499999989075320, 5.538419263543527649 ) ) ;
#12970=CARTESIAN_POINT ( 'NONE',  ( 1.990928271447991671, 228.1755604520575957, 6.746419455620825012 ) ) ;
#12976=CARTESIAN_POINT ( 'NONE',  ( 2.066987300000000083, 184.4999999989074979, 6.143825827087054492 ) ) ;
#12981=CARTESIAN_POINT ( 'NONE',  ( -7.386127300057498957E-16, 188.5699999975965397, 9.500000000000001776 ) ) ;
#12982=CARTESIAN_POINT ( 'NONE',  ( 2.599042177021809508, 227.7726851971488315, 8.749463102108622437 ) ) ;
#12983=CARTESIAN_POINT ( 'NONE',  ( -0.4907341119409533992, 228.2426455014340263, 10.13156071145469639 ) ) ;
#12988=EDGE_CURVE ( 'NONE', #14887, #14331, #13325, .T. ) ;
#12991=ORIENTED_EDGE ( 'NONE', *, *, #12708, .T. ) ;
#13002=PRODUCT ( 'finger', 'finger', '', ( #5604 ) ) ;
#13003=CARTESIAN_POINT ( 'NONE',  ( 2.500000000000000444, 186.2499999978150527, 8.035533905932739529 ) ) ;
#13004=CARTESIAN_POINT ( 'NONE',  ( 0.09789622041826544219, 228.2551367208810689, 10.16828408546989237 ) ) ;
#13008=B_SPLINE_CURVE_WITH_KNOTS ( 'NONE', 3,
 ( #13334, #12217, #4915, #4754, #13174, #3705, #6191, #8583, #5948, #13413, #2521, #3782, #11029, #15652, #4992, #9843, #14692, #13490, #7449, #12293, #6267, #4674, #2274, #7144, #11980, #1087, #10792, #7683, #8732, #12453, #6660, #7841, #13564, #9921, #10076, #6430, #437, #517, #14774, #1631, #11340, #10157, #11263, #5147, #283, #7526, #1553, #2674, #3860, #14926, #363, #5311, #5387, #12372, #6507, #15011, #1470, #6350, #12688, #8811, #5229, #4017, #5069, #1785, #11184, #4102, #8894, #10001, #11416, #13729, #4179, #15085, #8972, #9050, #13639, #14849, #208, #3935, #12607, #10234, #13876 ),
 .UNSPECIFIED., .F., .F.,
 ( 4, 2, 2, 2, 2, 2, 2, 2, 1, 1, 2, 2, 2, 2, 2, 1, 1, 1, 2, 2, 2, 2, 2, 1, 2, 2, 2, 2, 2, 1, 1, 2, 2, 2, 2, 1, 1, 2, 2, 2, 2, 1, 2, 2, 2, 4 ),
 ( 0.5000594734819727716, 0.5313057563892789048, 0.5469288978429318604, 0.5547404685697585602, 0.5586462539331716881, 0.5625520392965847050, 0.5937983222038856201, 0.6094214636575364663, 0.6172330343843618339, 0.6211388197477740736, 0.6230917124294802489, 0.6250446051111864243, 0.6562908880184755711, 0.6719140294721206441, 0.6797256001989425700, 0.6836313855623541436, 0.6855842782440593197, 0.6865607245849124629, 0.6870489477553389790, 0.6875371709257654951, 0.7187834538332094070, 0.7344065952869320846, 0.7422181660137933124, 0.7461239513772234266, 0.7480768440589389279, 0.7500297367406544291, 0.7812760196480968977, 0.7968991611018190202, 0.8047107318286800259, 0.8086165171921106953, 0.8105694098738263076, 0.8115458562146828925, 0.8125223025555396994, 0.8437685854629449755, 0.8593917269166470030, 0.8672032976434982388, 0.8711090830069236901, 0.8730619756886366378, 0.8750148683703494745, 0.9062611512777616340, 0.9218842927314683244, 0.9296958634583216696, 0.9336016488217482312, 0.9375074341851749038, 0.9687537170925875074, 1.000000000000000000 ),
 .UNSPECIFIED. ) ;
#13011=CARTESIAN_POINT ( 'NONE',  ( -2.500000000000000888, 187.6500000000000341, 8.035533905932737753 ) ) ;
#13018=CARTESIAN_POINT ( 'NONE',  ( -0.9654633820239412190, 226.3742042613716308, 4.631196276447603566 ) ) ;
#13021=CARTESIAN_POINT ( 'NONE',  ( 2.500000000000000444, 185.4800000002184959, 8.035533905932739529 ) ) ;
#13023=CARTESIAN_POINT ( 'NONE',  ( 1.786693786749917301, 227.9723819745098865, 6.159628423921897244 ) ) ;
#13028=CARTESIAN_POINT ( 'NONE',  ( -2.066987300000000971, 185.3999999989075604, 6.143825827087054492 ) ) ;
#13037=CARTESIAN_POINT ( 'NONE',  ( -0.8561741729129458411, 187.6999999989075150, 4.933012699999999029 ) ) ;
#13041=CARTESIAN_POINT ( 'NONE',  ( -5.999999999999999112, 195.9172377311516016, 6.220370292208425411 ) ) ;
#13049=CARTESIAN_POINT ( 'NONE',  ( -4.438452643612533777E-16, 185.0499999989075093, 9.066987300000000971 ) ) ;
#13050=CARTESIAN_POINT ( 'NONE',  ( 1.582883885363333798, 228.6577406203711575, 8.138983283465440977 ) ) ;
#13055=CARTESIAN_POINT ( 'NONE',  ( 2.500000000000000444, 188.7499999978150527, 5.964466094067262247 ) ) ;
#13062=CARTESIAN_POINT ( 'NONE',  ( 2.692585213447247661, 226.8629897650803855, 6.071564533969844746 ) ) ;
#13066=ORIENTED_EDGE ( 'NONE', *, *, #3180, .T. ) ;
#13071=ORIENTED_EDGE ( 'NONE', *, *, #534, .T. ) ;
#13080=CARTESIAN_POINT ( 'NONE',  ( -1.524659305057740610E-16, 189.0000000000000000, 4.500000000000000000 ) ) ;
#13082=CARTESIAN_POINT ( 'NONE',  ( 1.057043591443594943, 228.1937260751906820, 9.987734910156856216 ) ) ;
#13097=CARTESIAN_POINT ( 'NONE',  ( -2.272721100113404447, 226.6597439602984139, 5.472753651262165064 ) ) ;
#13098=CARTESIAN_POINT ( 'NONE',  ( 0.2845864031260020854, 190.0868499456632605, 4.208331950485010964 ) ) ;
#13099=CARTESIAN_POINT ( 'NONE',  ( 1.767766952966368654, 184.6300000002185016, 8.767766952966368876 ) ) ;
#13101=CARTESIAN_POINT ( 'NONE',  ( 0.4540882845019501568, 227.6260587419843091, 5.159427175404782240 ) ) ;
#13106=ORIENTED_EDGE ( 'NONE', *, *, #1079, .F. ) ;
#13107=CARTESIAN_POINT ( 'NONE',  ( -5.793705359219414319E-16, 187.2499999989075263, 9.066987300000000971 ) ) ;
#13114=CARTESIAN_POINT ( 'NONE',  ( 2.066987300000000527, 185.8999999989075320, 6.143825827087054492 ) ) ;
#13118=CARTESIAN_POINT ( 'NONE',  ( -5.999999999999999112, 222.7460571280668091, 12.08513476933103448 ) ) ;
#13120=CARTESIAN_POINT ( 'NONE',  ( -5.387129544537350156E-16, 185.2999999978150356, 9.500000000000001776 ) ) ;
#13127=CARTESIAN_POINT ( 'NONE',  ( -0.8561741729129455081, 184.6999999989075150, 4.933012699999999029 ) ) ;
#13128=CARTESIAN_POINT ( 'NONE',  ( 0.1295330668958723785, 227.6089706593652693, 5.110075818160935590 ) ) ;
#13136=CARTESIAN_POINT ( 'NONE',  ( 2.066987300000000083, 186.8499999989075206, 7.000000000000000000 ) ) ;
#13141=CARTESIAN_POINT ( 'NONE',  ( 2.691218579993890803, 227.7172414894967858, 8.586351398698511161 ) ) ;
#13163=CARTESIAN_POINT ( 'NONE',  ( 1.767766952966369098, 187.1999999978150697, 5.232233047033630235 ) ) ;
#13164=CARTESIAN_POINT ( 'NONE',  ( 0.6804430692981219275, 228.2300923459994237, 10.09465452691961751 ) ) ;
#13166=CARTESIAN_POINT ( 'NONE',  ( -1.170841281832480263, 188.9999999981235703, 4.783420672645316785 ) ) ;
#13171=CARTESIAN_POINT ( 'NONE',  ( 2.500000000000000000, 187.9500000000000455, 8.035533905932739529 ) ) ;
#13174=CARTESIAN_POINT ( 'NONE',  ( 0.7722673575711334060, 226.3571150073143770, 4.580780788055321295 ) ) ;
#13179=CARTESIAN_POINT ( 'NONE',  ( -2.826874103312618569, 227.6159703306986444, 8.288388193239365265 ) ) ;
#13182=CARTESIAN_POINT ( 'NONE',  ( -6.877907531704918753E-16, 187.7300000002184959, 9.500000000000001776 ) ) ;
#13185=CARTESIAN_POINT ( 'NONE',  ( -0.1316767729515891938, 227.6100531710845587, 5.113202173749356483 ) ) ;
#13189=DIRECTION ( 'NONE',  ( -6.123233995736766036E-17, 1.000000000000000000, 0.000000000000000000 ) ) ;
#13191=CARTESIAN_POINT ( 'NONE',  ( 0.8561741729129458411, 188.8999999989074752, 9.066987300000000971 ) ) ;
#13192=CARTESIAN_POINT ( 'NONE',  ( 2.066987300000000083, 186.5999999989074922, 7.856174172912946396 ) ) ;
#13199=B_SPLINE_CURVE_WITH_KNOTS ( 'NONE', 3,
 ( #7646, #774, #4360, #3977, #5187, #5562, #2796, #2717, #12337, #13765, #15258, #12417, #3899, #12494, #2874, #1962, #327, #13605, #1593, #14054, #6391, #5637, #12779, #10487, #7938, #9293, #1883, #11590, #6471, #6758, #11304, #10119, #11148, #14891 ),
 .UNSPECIFIED., .F., .F.,
 ( 4, 2, 2, 2, 2, 2, 2, 2, 2, 2, 2, 2, 2, 2, 2, 2, 4 ),
 ( 0.009569887493644234008, 0.01016303449442789927, 0.01075618149521156454, 0.01134932849599522980, 0.01194247549677889680, 0.01253562249756256207, 0.01312876949834622733, 0.01372191649912989260, 0.01431506349991355787, 0.01490821050069722487, 0.01550135750148089187, 0.01609450450226455887, 0.01668765150304822587, 0.01728079850383189287, 0.01787394550461555986, 0.01846709250539923033, 0.01906023950618289733 ),
 .UNSPECIFIED. ) ;
#13203=CARTESIAN_POINT ( 'NONE',  ( -0.8561741729129470624, 187.1999999989075434, 9.066987300000000971 ) ) ;
#13216=CARTESIAN_POINT ( 'NONE',  ( -2.940898392866930777E-15, 228.9118723800512498, 8.872930300147352511 ) ) ;
#13221=CARTESIAN_POINT ( 'NONE',  ( -1.016439536705160407E-17, 186.2499999989074979, 4.933012699999999029 ) ) ;
#13228=CARTESIAN_POINT ( 'NONE',  ( 1.501755279530002651, 226.4544816774725575, 4.867834892302488115 ) ) ;
#13246=CARTESIAN_POINT ( 'NONE',  ( 1.035533905932738197, 186.9499999978150413, 9.500000000000003553 ) ) ;
#13247=CARTESIAN_POINT ( 'NONE',  ( 0.4902782441471901231, 226.3376063806459513, 4.523301387120397088 ) ) ;
#13249=CARTESIAN_POINT ( 'NONE',  ( -0.2987180493634195022, 188.9999999992114397, 4.511177095514812940 ) ) ;
#13258=PLANE ( 'NONE',  #9938 ) ;
#13261=CARTESIAN_POINT ( 'NONE',  ( -0.7719220162881343938, 226.3554759578498476, 4.575941956958391899 ) ) ;
#13263=CARTESIAN_POINT ( 'NONE',  ( 2.500000000000000444, 187.0800000002184618, 8.035533905932739529 ) ) ;
#13265=CARTESIAN_POINT ( 'NONE',  ( 0.06504883222449296676, 227.6089665442046339, 5.110063933342379627 ) ) ;
#13266=CARTESIAN_POINT ( 'NONE',  ( 1.813601955701626300, 228.5298646585827385, 7.769670212251800656 ) ) ;
#13272=CARTESIAN_POINT ( 'NONE',  ( 0.8561741729129460632, 187.2999999989075661, 9.066987300000000971 ) ) ;
#13280=CARTESIAN_POINT ( 'NONE',  ( 1.461580736456472573, 186.5499999989075093, 8.461580736456474128 ) ) ;
#13283=CARTESIAN_POINT ( 'NONE',  ( 0.000000000000000000, 184.0000000000000000, 7.000000000000000000 ) ) ;
#13288=EDGE_CURVE ( 'NONE', #5259, #320, #9070, .T. ) ;
#13299=CARTESIAN_POINT ( 'NONE',  ( -0.8561741729129469514, 187.3999999989075889, 9.066987299999999195 ) ) ;
#13305=CARTESIAN_POINT ( 'NONE',  ( -2.974673115704016713, 227.4156934420934419, 7.698994310615434600 ) ) ;
#13308=ORIENTED_EDGE ( 'NONE', *, *, #8079, .F. ) ;
#13309=ORIENTED_EDGE ( 'NONE', *, *, #8379, .F. ) ;
#13313=CARTESIAN_POINT ( 'NONE',  ( -2.500000000000000444, 185.2000000000000171, 7.000000000000000000 ) ) ;
#13315=UNCERTAINTY_MEASURE_WITH_UNIT (LENGTH_MEASURE( 1.000000000000000082E-05 ), #7998, 'distance_accuracy_value', 'NONE');
#13322=CARTESIAN_POINT ( 'NONE',  ( 2.500000000000000444, 188.7499999978150527, 5.964466094067262247 ) ) ;
#13323=CARTESIAN_POINT ( 'NONE',  ( 2.050915569729614862, 227.9948459642048419, 9.402920486592190485 ) ) ;
#13325=( BOUNDED_CURVE ( )  B_SPLINE_CURVE ( 2, ( #5923, #10769, #10843, #15470, #15706, #7276, #12112, #9340, #14181 ),
 .UNSPECIFIED., .F., .F. ) 
 B_SPLINE_CURVE_WITH_KNOTS ( ( 3, 2, 2, 2, 3 ),
 ( 0.6428571428571429047, 0.6607142857142856984, 0.6785714285714286031, 0.6964285714285713969, 0.7142857142857143016 ),
 .UNSPECIFIED. ) 
 CURVE ( )  GEOMETRIC_REPRESENTATION_ITEM ( )  RATIONAL_B_SPLINE_CURVE ( ( 1.000000000000000000, 0.9238795325112867385, 1.000000000000000000, 0.9238795325112867385, 1.000000000000000000, 0.9238795325112867385, 1.000000000000000000, 0.9238795325112867385, 1.000000000000000000 ) ) 
 REPRESENTATION_ITEM ( '' )  );
#13326=CARTESIAN_POINT ( 'NONE',  ( -2.375777824384393888, 189.9842224717010879, 5.389868150937594748 ) ) ;
#13334=CARTESIAN_POINT ( 'NONE',  ( -5.385276659965230388E-16, 226.3251816629291966, 4.486670979098442480 ) ) ;
#13341=CARTESIAN_POINT ( 'NONE',  ( -2.500000000000000888, 188.3800000002185016, 8.035533905932737753 ) ) ;
#13342=CARTESIAN_POINT ( 'NONE',  ( -1.223735324759350984, 228.7813039559728168, 8.495841244274044968 ) ) ;
#13343=CARTESIAN_POINT ( 'NONE',  ( 1.691241850060078322, 228.6046986201012601, 7.985794961368397615 ) ) ;
#13347=CARTESIAN_POINT ( 'NONE',  ( 2.066987300000000971, 186.6999999989075150, 6.143825827087054492 ) ) ;
#13348=CARTESIAN_POINT ( 'NONE',  ( -0.8561741729129457301, 185.2999999989075377, 4.933012699999999029 ) ) ;
#13355=FACE_OUTER_BOUND ( 'NONE', #14547, .T. ) ;
#13356=CARTESIAN_POINT ( 'NONE',  ( 0.8561741729129455081, 189.1999999989075434, 4.933012699999999029 ) ) ;
#13363=CARTESIAN_POINT ( 'NONE',  ( 1.035533905932737753, 187.3499999999999943, 4.500000000000001776 ) ) ;
#13370=CARTESIAN_POINT ( 'NONE',  ( 0.000000000000000000, 184.0000000000000000, 7.000000000000000000 ) ) ;
#13372=CARTESIAN_POINT ( 'NONE',  ( -6.403569081242510563E-16, 188.2499999989075263, 9.066987300000000971 ) ) ;
#13379=CARTESIAN_POINT ( 'NONE',  ( -2.692660167145737304, 226.8630334657495666, 6.071693271619351684 ) ) ;
#13392=EDGE_CURVE ( 'NONE', #9005, #1272, #8951, .T. ) ;
#13398=DIRECTION ( 'NONE',  ( -0.9996329569789847991, -0.0003848699982329016438, -0.02708880205058770627 ) ) ;
#13401=CARTESIAN_POINT ( 'NONE',  ( 1.035533905932738197, 187.7499999978150527, 9.500000000000003553 ) ) ;
#13402=CARTESIAN_POINT ( 'NONE',  ( 2.600554376340839635, 226.8075635770346139, 5.908288162427849599 ) ) ;
#13405=VECTOR ( 'NONE', #3181, 1000.000000000000000 ) ;
#13406=CARTESIAN_POINT ( 'NONE',  ( -2.990007448523356537, 189.8992274272603993, 6.832429650438955449 ) ) ;
#13413=CARTESIAN_POINT ( 'NONE',  ( 1.104763767215224401, 226.3928744374965447, 4.686231709593007722 ) ) ;
#13423=CARTESIAN_POINT ( 'NONE',  ( -2.500000000000000444, 184.3499999999999943, 5.964466094067261359 ) ) ;
#13425=CARTESIAN_POINT ( 'NONE',  ( 0.3231974900581740529, 228.9035839249116009, 8.848992768962338218 ) ) ;
#13430=CARTESIAN_POINT ( 'NONE',  ( -9.825582188149883933E-17, 187.6499999989075320, 4.933012699999999029 ) ) ;
#13432=CARTESIAN_POINT ( 'NONE',  ( -9.825582188149883933E-17, 187.6499999989075320, 4.933012699999999029 ) ) ;
#13439=CARTESIAN_POINT ( 'NONE',  ( 5.999999999999999112, 201.6409668649147022, 13.30942870683726120 ) ) ;
#13440=CARTESIAN_POINT ( 'NONE',  ( -1.965116437629976787E-16, 189.2499999989075263, 4.933012699999999029 ) ) ;
#13444=CYLINDRICAL_SURFACE ( 'NONE', #956, 2.500000000000000444 ) ;
#13447=CARTESIAN_POINT ( 'NONE',  ( -2.066760391300492827E-16, 189.4499999989075150, 4.933012699999999029 ) ) ;
#13458=CARTESIAN_POINT ( 'NONE',  ( 1.461580736456472795, 186.9499999989075150, 5.538419263543527649 ) ) ;
#13465=CARTESIAN_POINT ( 'NONE',  ( -2.439580969806472321, 226.7272467340407331, 5.671663139905907869 ) ) ;
#13467=VERTEX_POINT ( 'NONE', #7078 ) ;
#13480=CARTESIAN_POINT ( 'NONE',  ( -1.035533905932737975, 187.3499999978151038, 4.500000000000000888 ) ) ;
#13481=CARTESIAN_POINT ( 'NONE',  ( 3.000032282732917555, 227.2742683068891552, 7.282695486718367306 ) ) ;
#13483=CARTESIAN_POINT ( 'NONE',  ( -0.4481745786268478415, 189.0473500653932319, 10.15604835757928726 ) ) ;
#13484=VERTEX_POINT ( 'NONE', #9628 ) ;
#13490=CARTESIAN_POINT ( 'NONE',  ( 2.057832045933806420, 226.5876095930653094, 5.260198610313286061 ) ) ;
#13495=CARTESIAN_POINT ( 'NONE',  ( -2.500000000000000444, 184.4499999999999886, 8.035533905932737753 ) ) ;
#13497=CARTESIAN_POINT ( 'NONE',  ( 1.990705347729657237, 228.2501094229765215, 6.961721135629644230 ) ) ;
#13498=CARTESIAN_POINT ( 'NONE',  ( 0.000000000000000000, 184.0000000000000000, 7.000000000000000000 ) ) ;
#13503=CARTESIAN_POINT ( 'NONE',  ( -1.461580736456473240, 186.9499999989075150, 5.538419263543526760 ) ) ;
#13511=CARTESIAN_POINT ( 'NONE',  ( -0.8983937855600439004, 189.0000000000000284, 9.343143558360589296 ) ) ;
#13521=CARTESIAN_POINT ( 'NONE',  ( 0.8561741729129455081, 186.9999999989074979, 4.933012699999999029 ) ) ;
#13540=CARTESIAN_POINT ( 'NONE',  ( -1.329004440443209090, 226.4243434115648199, 4.778997713384572243 ) ) ;
#13549=CARTESIAN_POINT ( 'NONE',  ( -2.500000000000000444, 187.4499999978150981, 5.964466094067261359 ) ) ;
#13550=CARTESIAN_POINT ( 'NONE',  ( 2.066987300000000083, 184.9999999989074979, 7.856174172912946396 ) ) ;
#13554=CARTESIAN_POINT ( 'NONE',  ( -1.035533905932739751, 186.9199999975965625, 9.500000000000003553 ) ) ;
#13555=CARTESIAN_POINT ( 'NONE',  ( -1.132970084112051579, 227.7246690377758398, 5.444219334014433365 ) ) ;
#13556=CARTESIAN_POINT ( 'NONE',  ( 2.548737910730607403, 227.7996913757372397, 8.828908791204545636 ) ) ;
#13558=CARTESIAN_POINT ( 'NONE',  ( -3.024391221093167825, 189.3078535938050209, 6.878255494570371553 ) ) ;
#13564=CARTESIAN_POINT ( 'NONE',  ( 2.769757902222948154, 226.9188947913604295, 6.236235719881334738 ) ) ;
#13568=EDGE_CURVE ( 'NONE', #7504, #13484, #10175, .T. ) ;
#13570=CARTESIAN_POINT ( 'NONE',  ( -2.500000000000000444, 186.0500000000000114, 8.035533905932737753 ) ) ;
#13577=CARTESIAN_POINT ( 'NONE',  ( -6.268043809681822509E-16, 188.0499999989075093, 9.066987300000000971 ) ) ;
#13578=CARTESIAN_POINT ( 'NONE',  ( 1.035533905932737753, 187.2499999978150811, 4.500000000000001776 ) ) ;
#13579=CARTESIAN_POINT ( 'NONE',  ( -2.066987300000000971, 188.8999999989075320, 7.856174172912944620 ) ) ;
#13584=CARTESIAN_POINT ( 'NONE',  ( 0.06635618020083272617, 190.0874453959174275, 4.202409577918525763 ) ) ;
#13586=CARTESIAN_POINT ( 'NONE',  ( -1.461580736456473240, 188.5499999989075093, 5.538419263543526760 ) ) ;
#13588=CARTESIAN_POINT ( 'NONE',  ( 0.3313399881279415204, 189.6987757587769750, 10.37797768716739988 ) ) ;
#13590=CYLINDRICAL_SURFACE ( 'NONE', #8088, 2.500000000000000444 ) ;
#13591=CARTESIAN_POINT ( 'NONE',  ( -1.524659305057740610E-16, 189.0000000000000000, 4.500000000000000000 ) ) ;
#13596=ORIENTED_EDGE ( 'NONE', *, *, #13677, .F. ) ;
#13597=CARTESIAN_POINT ( 'NONE',  ( 1.461580736456472795, 188.5499999989075093, 5.538419263543527649 ) ) ;
#13605=CARTESIAN_POINT ( 'NONE',  ( -3.002032555434545280, 189.8710560290441265, 7.456578097359207291 ) ) ;
#13613=CARTESIAN_POINT ( 'NONE',  ( -1.826734563482391938, 226.5243062390148623, 5.073637952221710101 ) ) ;
#13619=CARTESIAN_POINT ( 'NONE',  ( 0.07162589071487505954, 189.0001276426230561, 4.501026264287848910 ) ) ;
#13625=CARTESIAN_POINT ( 'NONE',  ( -1.767766952966369098, 184.9999999978150527, 5.232233047033630235 ) ) ;
#13628=CARTESIAN_POINT ( 'NONE',  ( -1.050320854595332420E-16, 188.2000000000000171, 4.500000000000000000 ) ) ;
#13630=CARTESIAN_POINT ( 'NONE',  ( -5.929230630780102373E-16, 186.1699999975965625, 9.500000000000001776 ) ) ;
#13631=CARTESIAN_POINT ( 'NONE',  ( -1.724657202313207849, 227.9349080091615178, 6.051401474621576071 ) ) ;
#13632=CARTESIAN_POINT ( 'NONE',  ( -2.051698115976866355, 227.9946287341323057, 9.402281653761695779 ) ) ;
#13633=CARTESIAN_POINT ( 'NONE',  ( -2.022860936364483386, 188.9999999987646788, 8.476761716666477042 ) ) ;
#13639=CARTESIAN_POINT ( 'NONE',  ( 1.189709685105988513, 228.1759518697011231, 9.935475612313785732 ) ) ;
#13643=PRODUCT_DEFINITION_FORMATION_WITH_SPECIFIED_SOURCE ( 'ANY', '', #13002, .NOT_KNOWN. ) ;
#13645=CARTESIAN_POINT ( 'NONE',  ( -1.035533905932737975, 185.8500000000000227, 4.500000000000000888 ) ) ;
#13648=CARTESIAN_POINT ( 'NONE',  ( 0.3253281796544252868, 227.6173729869818771, 5.134342219554626219 ) ) ;
#13652=CARTESIAN_POINT ( 'NONE',  ( -1.767766952966369098, 184.2999999999999829, 5.232233047033630235 ) ) ;
#13655=CARTESIAN_POINT ( 'NONE',  ( 2.066987300000000083, 187.6499999989075320, 7.000000000000000000 ) ) ;
#13662=CARTESIAN_POINT ( 'NONE',  ( -5.999999999999999112, 195.9172377311516016, 6.220370292208425411 ) ) ;
#13665=CARTESIAN_POINT ( 'NONE',  ( 2.378934927046848724, 189.7843313986748512, 9.198200349355834859 ) ) ;
#13667=CARTESIAN_POINT ( 'NONE',  ( 2.605749592490243405, 189.8045552418427064, 8.848848054815309894 ) ) ;
#13668=AXIS2_PLACEMENT_3D ( 'NONE', #8694, #2556, #1353 ) ;
#13673=ORIENTED_EDGE ( 'NONE', *, *, #12988, .F. ) ;
#13674=CARTESIAN_POINT ( 'NONE',  ( -1.592421940838084637E-16, 188.6499999989075320, 4.933012699999999029 ) ) ;
#13677=EDGE_CURVE ( 'NONE', #14887, #13744, #10323, .T. ) ;
#13678=ORIENTED_EDGE ( 'NONE', *, *, #6410, .T. ) ;
#13680=CARTESIAN_POINT ( 'NONE',  ( 1.035533905932737975, 185.7500000000000000, 4.500000000000001776 ) ) ;
#13688=CARTESIAN_POINT ( 'NONE',  ( -6.877907531704918753E-16, 189.0499999989075093, 9.066987300000000971 ) ) ;
#13695=CARTESIAN_POINT ( 'NONE',  ( -0.7777163206635004933, 228.2226383035325057, 10.07273956871427956 ) ) ;
#13710=CARTESIAN_POINT ( 'NONE',  ( 2.500000000000000444, 187.0999999978150754, 7.000000000000000000 ) ) ;
#13717=CARTESIAN_POINT ( 'NONE',  ( -1.767766952966369765, 186.8699999975965511, 8.767766952966368876 ) ) ;
#13718=CARTESIAN_POINT ( 'NONE',  ( -0.7013870287959992345, 228.8704690996177646, 8.753355264767147759 ) ) ;
#13719=CARTESIAN_POINT ( 'NONE',  ( -2.976076845141470972, 227.1639356932526539, 6.957862568523350610 ) ) ;
#13720=CARTESIAN_POINT ( 'NONE',  ( -2.593495354050888491, 189.9612784629288456, 5.721711197761079504 ) ) ;
#13729=CARTESIAN_POINT ( 'NONE',  ( 1.569541343170871794, 228.1129751185468706, 9.750325026063840994 ) ) ;
#13733=CARTESIAN_POINT ( 'NONE',  ( -7.420008617947670970E-16, 188.5999999999999943, 9.500000000000001776 ) ) ;
#13735=CARTESIAN_POINT ( 'NONE',  ( 1.035533905932737753, 187.3499999999999659, 4.500000000000000888 ) ) ;
#13737=CARTESIAN_POINT ( 'NONE',  ( 0.4220225674029139951, 227.6236908799334344, 5.152588654748359254 ) ) ;
#13741=CARTESIAN_POINT ( 'NONE',  ( 2.500000000000000444, 184.7999999999999829, 7.000000000000000000 ) ) ;
#13743=CARTESIAN_POINT ( 'NONE',  ( -1.461580736456473018, 187.1499999989075320, 5.538419263543527649 ) ) ;
#13744=VERTEX_POINT ( 'NONE', #9443 ) ;
#13747=CARTESIAN_POINT ( 'NONE',  ( 0.000000000000000000, 229.2449477060184222, 9.834870838912449287 ) ) ;
#13749=CARTESIAN_POINT ( 'NONE',  ( 1.955037902524143778, 188.9999999998599378, 8.565347031248222720 ) ) ;
#13751=CARTESIAN_POINT ( 'NONE',  ( 0.7847739342500663628, 189.7061529762492569, 10.28987046638656544 ) ) ;
#13755=ORIENTED_EDGE ( 'NONE', *, *, #4732, .T. ) ;
#13756=CARTESIAN_POINT ( 'NONE',  ( -6.098637220230962441E-17, 187.0499999989075093, 4.933012699999999029 ) ) ;
#13762=ORIENTED_EDGE ( 'NONE', *, *, #14457, .T. ) ;
#13765=CARTESIAN_POINT ( 'NONE',  ( -2.267268076141566002, 189.9944061229849979, 5.253861789810808425 ) ) ;
#13771=CARTESIAN_POINT ( 'NONE',  ( -1.767766952966369765, 186.9000000000000057, 8.767766952966368876 ) ) ;
#13786=CARTESIAN_POINT ( 'NONE',  ( -2.500000000000000444, 187.5499999978150356, 8.035533905932737753 ) ) ;
#13791=CARTESIAN_POINT ( 'NONE',  ( -1.035533905932737753, 185.8199999975965682, 4.500000000000000888 ) ) ;
#13792=CARTESIAN_POINT ( 'NONE',  ( -1.964265005259087538, 228.3667458257928047, 7.298573719466742382 ) ) ;
#13793=CARTESIAN_POINT ( 'NONE',  ( -2.548338711267991386, 226.7802694665861338, 5.827877803219676522 ) ) ;
#13794=ORIENTED_EDGE ( 'NONE', *, *, #210, .F. ) ;
#13796=ORIENTED_EDGE ( 'NONE', *, *, #9412, .F. ) ;
#13800=CARTESIAN_POINT ( 'NONE',  ( -1.965116437629976787E-16, 189.6999999978150697, 4.500000000000000000 ) ) ;
#13807=CARTESIAN_POINT ( 'NONE',  ( 1.035533905932737753, 188.9500000000000171, 4.500000000000001776 ) ) ;
#13808=CARTESIAN_POINT ( 'NONE',  ( -1.767766952966369320, 187.5000000000000000, 5.232233047033630235 ) ) ;
#13809=CARTESIAN_POINT ( 'NONE',  ( -1.051851325171203388, 227.7069327454752283, 5.392995910236884960 ) ) ;
#13811=EDGE_CURVE ( 'NONE', #3723, #8478, #15195, .T. ) ;
#13814=CARTESIAN_POINT ( 'NONE',  ( 1.035533905932738419, 184.6500000000000057, 9.500000000000003553 ) ) ;
#13816=CARTESIAN_POINT ( 'NONE',  ( -1.016439536705160407E-17, 186.2499999989074979, 4.933012699999999029 ) ) ;
#13822=CARTESIAN_POINT ( 'NONE',  ( 0.000000000000000000, 215.7452399395091049, 13.29567785264566027 ) ) ;
#13823=CARTESIAN_POINT ( 'NONE',  ( 2.978694808295341279, 189.3199727616403720, 6.623693945629629987 ) ) ;
#13826=CARTESIAN_POINT ( 'NONE',  ( 0.000000000000000000, 189.6977690162252657, 10.38967773564543862 ) ) ;
#13831=CARTESIAN_POINT ( 'NONE',  ( -0.8561741729129455081, 185.4999999989075548, 4.933012699999999029 ) ) ;
#13860=CARTESIAN_POINT ( 'NONE',  ( 1.767766952966368432, 186.9999999978150527, 8.767766952966368876 ) ) ;
#13864=CARTESIAN_POINT ( 'NONE',  ( -2.500000000000000444, 186.8199999975965397, 8.035533905932737753 ) ) ;
#13865=CARTESIAN_POINT ( 'NONE',  ( -1.973877840180719989, 228.3455757694837303, 7.237433389386023208 ) ) ;
#13866=CARTESIAN_POINT ( 'NONE',  ( -0.4900172623563870955, 226.3376062179358996, 4.523300904952406221 ) ) ;
#13876=CARTESIAN_POINT ( 'NONE',  ( -1.016439536705160407E-17, 228.2551366889529731, 10.16828399152529272 ) ) ;
#13883=CARTESIAN_POINT ( 'NONE',  ( -2.500000000000000444, 186.0000000000000000, 7.000000000000000000 ) ) ;
#13884=CARTESIAN_POINT ( 'NONE',  ( -1.885954199498669270, 228.0508284750123664, 6.386186391668034368 ) ) ;
#13890=CARTESIAN_POINT ( 'NONE',  ( -5.454892180317694184E-16, 185.4000000000000057, 9.500000000000001776 ) ) ;
#13892=CARTESIAN_POINT ( 'NONE',  ( 0.8561741729129460632, 186.6999999989075150, 9.066987299999999195 ) ) ;
#13898=CARTESIAN_POINT ( 'NONE',  ( -5.999999999999999112, 222.7460571280668091, 12.08513476933103448 ) ) ;
#13900=CARTESIAN_POINT ( 'NONE',  ( 2.208001381734123747, 188.9999999987420836, 8.182568187628087131 ) ) ;
#13907=ORIENTED_EDGE ( 'NONE', *, *, #12935, .T. ) ;
#13908=CARTESIAN_POINT ( 'NONE',  ( -1.461580736456473240, 186.1499999989075320, 5.538419263543526760 ) ) ;
#13932=CARTESIAN_POINT ( 'NONE',  ( -5.385276659965230388E-16, 226.3251816629291966, 4.486670979098442480 ) ) ;
#13939=CARTESIAN_POINT ( 'NONE',  ( 1.767766952966368432, 188.5999999978150470, 8.767766952966368876 ) ) ;
#13946=CARTESIAN_POINT ( 'NONE',  ( -1.785671180686238868, 228.5485690224869586, 7.823689482036285447 ) ) ;
#13958=DIRECTION ( 'NONE',  ( -6.123233995736766036E-17, 1.000000000000000000, 0.000000000000000000 ) ) ;
#13964=CARTESIAN_POINT ( 'NONE',  ( -2.500000000000000444, 185.0999999978150754, 7.000000000000000000 ) ) ;
#13967=CARTESIAN_POINT ( 'NONE',  ( 1.692341931978252223, 227.9167330860961442, 5.998911260178718230 ) ) ;
#13973=CARTESIAN_POINT ( 'NONE',  ( -1.050320854595332420E-16, 188.2000000000000171, 4.500000000000000000 ) ) ;
#13980=CARTESIAN_POINT ( 'NONE',  ( 2.283493650000000486, 184.1249999994537632, 7.000000000000000000 ) ) ;
#13982=CARTESIAN_POINT ( 'NONE',  ( 2.832543757336219326, 189.3479566575481385, 6.034102192250282215 ) ) ;
#13985=CARTESIAN_POINT ( 'NONE',  ( 0.9660064634511277282, 228.8301302322938966, 8.636854315157751927 ) ) ;
#13990=CARTESIAN_POINT ( 'NONE',  ( -2.066760391300492827E-16, 189.4499999989075150, 4.933012699999999029 ) ) ;
#13997=CARTESIAN_POINT ( 'NONE',  ( -2.066987300000000971, 184.6999999989075150, 7.856174172912944620 ) ) ;
#14002=CARTESIAN_POINT ( 'NONE',  ( 3.659182332138577465E-16, 215.0542865858234336, 7.296348638359030581 ) ) ;
#14005=CARTESIAN_POINT ( 'NONE',  ( -0.6829126361173057935, 228.2303005364134094, 10.09526665386122346 ) ) ;
#14020=CARTESIAN_POINT ( 'NONE',  ( -0.8561741729129452860, 184.6999999989075150, 4.933012699999999029 ) ) ;
#14024=CARTESIAN_POINT ( 'NONE',  ( -1.524659305057740610E-16, 189.0000000000000000, 4.500000000000000000 ) ) ;
#14026=CARTESIAN_POINT ( 'NONE',  ( -2.500000000000000444, 189.1199999975965795, 5.964466094067261359 ) ) ;
#14027=CARTESIAN_POINT ( 'NONE',  ( 2.050915569729614862, 227.9948459642048419, 9.402920486592190485 ) ) ;
#14032=CARTESIAN_POINT ( 'NONE',  ( -1.768703179866833342, 189.0000639513403939, 5.233169770031948609 ) ) ;
#14042=CARTESIAN_POINT ( 'NONE',  ( 0.000000000000000000, 186.4999999978150527, 4.500000000000000000 ) ) ;
#14043=CARTESIAN_POINT ( 'NONE',  ( -1.939606487604890850, 228.4085856529902117, 7.419409526801750587 ) ) ;
#14047=CARTESIAN_POINT ( 'NONE',  ( -2.500000000000000444, 186.7500000000000000, 5.964466094067261359 ) ) ;
#14054=CARTESIAN_POINT ( 'NONE',  ( -2.917684139655223330, 189.8446451309251302, 8.046806756071347877 ) ) ;
#14057=CARTESIAN_POINT ( 'NONE',  ( -0.5227993896667307849, 227.6261285884132235, 5.159628895875891352 ) ) ;
#14058=CARTESIAN_POINT ( 'NONE',  ( 0.2588337889006175341, 228.9066910274044346, 8.857966258178848307 ) ) ;
#14064=CARTESIAN_POINT ( 'NONE',  ( 0.8561741729129457301, 185.1999999989075150, 4.933012699999999029 ) ) ;
#14066=EDGE_LOOP ( 'NONE', ( #11977, #10539, #2555, #13596 ) ) ;
#14076=CARTESIAN_POINT ( 'NONE',  ( 5.999999999999999112, 186.5669965222008670, 9.317226423031115701 ) ) ;
#14085=CARTESIAN_POINT ( 'NONE',  ( 3.659182332138577465E-16, 202.3580807015429457, 7.308726713069390257 ) ) ;
#14087=CARTESIAN_POINT ( 'NONE',  ( 1.035533905932737975, 184.9499999999999886, 4.500000000000001776 ) ) ;
#14092=CARTESIAN_POINT ( 'NONE',  ( -2.066987300000000083, 185.5999999989075775, 6.143825827087054492 ) ) ;
#14098=CARTESIAN_POINT ( 'NONE',  ( 1.767766952966368432, 188.6699999975965341, 8.767766952966368876 ) ) ;
#14099=CARTESIAN_POINT ( 'NONE',  ( 0.3927937339364459546, 226.3329534510998542, 4.509583726312986762 ) ) ;
#14101=CARTESIAN_POINT ( 'NONE',  ( -2.500000000000000444, 186.0000000000000000, 7.000000000000000000 ) ) ;
#14118=CARTESIAN_POINT ( 'NONE',  ( -5.387129544537350156E-16, 185.2999999978150356, 9.500000000000001776 ) ) ;
#14119=CARTESIAN_POINT ( 'NONE',  ( -1.984331290054332841, 228.3135221411288285, 7.144860682478253011 ) ) ;
#14123=CARTESIAN_POINT ( 'NONE',  ( -5.929230630780102373E-16, 186.2000000000000171, 9.500000000000001776 ) ) ;
#14130=CARTESIAN_POINT ( 'NONE',  ( -1.035533905932737975, 186.6500000000000057, 4.500000000000001776 ) ) ;
#14131=CARTESIAN_POINT ( 'NONE',  ( -2.761685261155654381, 227.6665753604594045, 8.437282647672972757 ) ) ;
#14132=FILL_AREA_STYLE_COLOUR ( '', #14982 ) ;
#14133=CARTESIAN_POINT ( 'NONE',  ( 1.155845512882874626, 189.4310859332073562, 4.210941953806538685 ) ) ;
#14134=CARTESIAN_POINT ( 'NONE',  ( -1.035533905932739529, 185.2800000002184504, 9.500000000000003553 ) ) ;
#14137=CARTESIAN_POINT ( 'NONE',  ( 0.1297182620452491941, 228.9108343529357228, 8.869932418632497928 ) ) ;
#14142=CARTESIAN_POINT ( 'NONE',  ( -1.461580736456473018, 184.5499999989075093, 5.538419263543526760 ) ) ;
#14146=CARTESIAN_POINT ( 'NONE',  ( -1.767766952966369765, 186.0999999999999943, 8.767766952966368876 ) ) ;
#14148=B_SPLINE_CURVE_WITH_KNOTS ( 'NONE', 3,
 ( #9218, #3162, #401, #5271, #4438, #8774, #690, #4062, #1515, #11225, #9963, #8932, #7491, #2638, #1434, #8019, #10041, #12857, #6838, #6311, #250, #5110, #14814, #15578, #4838, #11749, #9371, #3555, #5873, #15416, #14131, #15655, #8181, #13179, #4678, #12066, #3237, #1090, #11818, #9450, #6990, #10720, #1010, #2040, #14282, #5793, #10796, #8102, #3391, #9531, #11984, #4598, #851, #14452, #925, #4757, #2360, #8259, #10639, #4515, #15501, #13097, #7067, #2194, #11902, #14366, #3472, #8341, #5717, #6915, #1164, #2278, #7148, #12940, #5952, #9614, #8424, #13018, #13261, #7228, #6033, #10879 ),
 .UNSPECIFIED., .F., .F.,
 ( 4, 2, 2, 2, 2, 2, 2, 2, 1, 1, 2, 2, 2, 2, 2, 1, 1, 2, 2, 2, 2, 2, 1, 2, 2, 2, 2, 2, 1, 1, 1, 2, 2, 2, 2, 1, 1, 1, 2, 2, 2, 2, 1, 2, 2, 2, 4 ),
 ( 0.000000000000000000, 0.03125000000001913053, 0.04687500000002882417, 0.05468750000003370221, 0.05859375000003642919, 0.06250000000003916312, 0.09375000000006236678, 0.1093750000000735939, 0.1171875000000792005, 0.1210937500000814487, 0.1230468750000829475, 0.1250000000000844602, 0.1562500000001039724, 0.1718750000001137423, 0.1796875000001185163, 0.1835937500001208755, 0.1855468750001219302, 0.1865234375001218747, 0.1875000000001218192, 0.2187500000001719458, 0.2343750000001968703, 0.2421875000002100264, 0.2460937500002166600, 0.2480468750002199629, 0.2500000000002232659, 0.2812500000002847722, 0.2968750000003155254, 0.3046875000003299583, 0.3085937500003371192, 0.3105468750003417822, 0.3115234375003440581, 0.3120117187503441136, 0.3125000000003441136, 0.3437500000002909895, 0.3593750000002637890, 0.3671875000002502998, 0.3710937500002434719, 0.3730468750002405853, 0.3740234375002385314, 0.3750000000002364775, 0.4062500000001775247, 0.4218750000001476597, 0.4296875000001331157, 0.4335937500001255107, 0.4375000000001179057, 0.4687500000000588973, 0.5000000000000000000 ),
 .UNSPECIFIED. ) ;
#14149=CARTESIAN_POINT ( 'NONE',  ( 1.461580736456472573, 185.1499999989075320, 8.461580736456474128 ) ) ;
#14150=LINE ( 'NONE', #12875, #13405 ) ;
#14151=CARTESIAN_POINT ( 'NONE',  ( -2.066987300000000527, 187.0499999989075093, 7.000000000000000000 ) ) ;
#14155=CARTESIAN_POINT ( 'NONE',  ( 5.999999999999999112, 227.2817795252328210, 4.165129161027028459 ) ) ;
#14156=ORIENTED_EDGE ( 'NONE', *, *, #10754, .F. ) ;
#14172=CARTESIAN_POINT ( 'NONE',  ( -2.500000000000000888, 188.3499999978150186, 8.035533905932737753 ) ) ;
#14174=CARTESIAN_POINT ( 'NONE',  ( -1.035533905932737753, 185.7499999978150527, 4.500000000000001776 ) ) ;
#14176=CARTESIAN_POINT ( 'NONE',  ( -1.767766952966369320, 189.0699999975965397, 5.232233047033630235 ) ) ;
#14177=CARTESIAN_POINT ( 'NONE',  ( 2.998835045281009304, 227.2583357984985639, 7.235791215503737384 ) ) ;
#14181=CARTESIAN_POINT ( 'NONE',  ( 2.500000000000000000, 188.6999999978150697, 7.000000000000000000 ) ) ;
#14196=CARTESIAN_POINT ( 'NONE',  ( 1.767766952966369320, 185.5999999978150754, 5.232233047033630235 ) ) ;
#14197=CARTESIAN_POINT ( 'NONE',  ( -1.826974499845722466, 228.5193582813216153, 7.739327195479140720 ) ) ;
#14201=AXIS2_PLACEMENT_3D ( 'NONE', #6680, #11513, #1651 ) ;
#14203=CARTESIAN_POINT ( 'NONE',  ( -1.767766952966369765, 188.5000000000000000, 8.767766952966368876 ) ) ;
#14206=ORIENTED_EDGE ( 'NONE', *, *, #4080, .T. ) ;
#14208=CARTESIAN_POINT ( 'NONE',  ( 2.500000000000000444, 186.4500000000000171, 5.964466094067262247 ) ) ;
#14210=( NAMED_UNIT ( * ) PLANE_ANGLE_UNIT ( ) SI_UNIT ( $, .RADIAN. ) );
#14214=CARTESIAN_POINT ( 'NONE',  ( 0.5467140873060455375, 228.8869147685435053, 8.800851294624202126 ) ) ;
#14218=VERTEX_POINT ( 'NONE', #14673 ) ;
#14219=CARTESIAN_POINT ( 'NONE',  ( 1.461580736456472795, 184.9499999989075150, 8.461580736456474128 ) ) ;
#14224=CARTESIAN_POINT ( 'NONE',  ( -2.066987300000000083, 184.8499999989075206, 7.000000000000000000 ) ) ;
#14226=CARTESIAN_POINT ( 'NONE',  ( 0.8561741729129457301, 186.7999999989075093, 4.933012699999999029 ) ) ;
#14229=CARTESIAN_POINT ( 'NONE',  ( -1.558540622947912624E-16, 189.0624999997268390, 4.500000000000000000 ) ) ;
#14230=CARTESIAN_POINT ( 'NONE',  ( -5.999999999999999112, 227.2817795252328210, 4.165129161027028459 ) ) ;
#14237=CARTESIAN_POINT ( 'NONE',  ( 2.066987300000000083, 185.2499999989074979, 7.000000000000000000 ) ) ;
#14238=CARTESIAN_POINT ( 'NONE',  ( 1.003991088089927430, 227.6914879785015273, 5.348390542306004747 ) ) ;
#14244=CARTESIAN_POINT ( 'NONE',  ( -2.066987300000000083, 184.7999999989075093, 6.143825827087054492 ) ) ;
#14251=CARTESIAN_POINT ( 'NONE',  ( 2.961752869269595134, 227.1327854310254111, 6.866142280206398496 ) ) ;
#14258=CARTESIAN_POINT ( 'NONE',  ( 2.066987300000000083, 184.4499999989075150, 7.000000000000000000 ) ) ;
#14260=VERTEX_POINT ( 'NONE', #6483 ) ;
#14268=CARTESIAN_POINT ( 'NONE',  ( 2.500000000000000444, 184.7499999978150527, 5.964466094067262247 ) ) ;
#14269=CARTESIAN_POINT ( 'NONE',  ( -0.5160604560792059203, 228.8899596144369752, 8.809644983231040172 ) ) ;
#14271=CARTESIAN_POINT ( 'NONE',  ( 0.07962197837298144731, 190.0874091994478761, 4.202769589527701299 ) ) ;
#14273=CARTESIAN_POINT ( 'NONE',  ( 4.404571325722361763E-17, 185.7999999999999829, 4.500000000000000000 ) ) ;
#14278=EDGE_CURVE ( 'NONE', #25, #8865, #6541, .T. ) ;
#14282=CARTESIAN_POINT ( 'NONE',  ( -2.999949572879441639, 227.1989808014691903, 7.061061364497972725 ) ) ;
#14286=CARTESIAN_POINT ( 'NONE',  ( -1.767766952966369765, 186.0300000002184788, 8.767766952966368876 ) ) ;
#14289=CARTESIAN_POINT ( 'NONE',  ( 1.237586355860756271, 228.7707919832083689, 8.465482067366952634 ) ) ;
#14298=FACE_OUTER_BOUND ( 'NONE', #1158, .T. ) ;
#14300=CARTESIAN_POINT ( 'NONE',  ( 0.8561741729129461742, 185.6999999989075150, 9.066987300000000971 ) ) ;
#14304=CARTESIAN_POINT ( 'NONE',  ( 5.999999999999999112, 222.7460571280668091, 12.08513476933103448 ) ) ;
#14306=CARTESIAN_POINT ( 'NONE',  ( -2.500000000000000444, 185.0999999978150754, 7.000000000000000000 ) ) ;
#14311=ORIENTED_EDGE ( 'NONE', *, *, #2200, .T. ) ;
#14313=CARTESIAN_POINT ( 'NONE',  ( -2.066987300000000083, 184.7999999989075093, 6.143825827087054492 ) ) ;
#14316=ORIENTED_EDGE ( 'NONE', *, *, #13811, .F. ) ;
#14320=CARTESIAN_POINT ( 'NONE',  ( -2.066987300000000083, 186.3999999989075320, 6.143825827087054492 ) ) ;
#14328=CARTESIAN_POINT ( 'NONE',  ( 2.053141855112443626, 226.5855735425530497, 5.254201149538955562 ) ) ;
#14331=VERTEX_POINT ( 'NONE', #11395 ) ;
#14334=( BOUNDED_CURVE ( )  B_SPLINE_CURVE ( 2, ( #6708, #410, #5433, #7809, #15209, #1524, #11537, #14980, #12580 ),
 .UNSPECIFIED., .F., .F. ) 
 B_SPLINE_CURVE_WITH_KNOTS ( ( 3, 2, 2, 2, 3 ),
 ( 0.2857142857142856984, 0.3035714285714285476, 0.3214285714285715079, 0.3392857142857143571, 0.3571428571428572063 ),
 .UNSPECIFIED. ) 
 CURVE ( )  GEOMETRIC_REPRESENTATION_ITEM ( )  RATIONAL_B_SPLINE_CURVE ( ( 1.000000000000000000, 0.9238795325112867385, 1.000000000000000000, 0.9238795325112867385, 1.000000000000000000, 0.9238795325112867385, 1.000000000000000000, 0.9238795325112865164, 1.000000000000000222 ) ) 
 REPRESENTATION_ITEM ( '' )  );
#14338=AXIS2_PLACEMENT_3D ( 'NONE', #9496, #9661, #9745 ) ;
#14348=CARTESIAN_POINT ( 'NONE',  ( -1.035533905932739751, 189.2499999978150811, 9.500000000000003553 ) ) ;
#14350=CARTESIAN_POINT ( 'NONE',  ( 0.4870669733929915424, 228.2428440931186628, 10.13214456346285708 ) ) ;
#14354=ORIENTED_EDGE ( 'NONE', *, *, #8973, .T. ) ;
#14357=DIRECTION ( 'NONE',  ( -1.000000000000000000, 0.000000000000000000, 0.000000000000000000 ) ) ;
#14366=CARTESIAN_POINT ( 'NONE',  ( -2.137511978810349156, 226.6127469305739339, 5.334277523823343081 ) ) ;
#14370=CARTESIAN_POINT ( 'NONE',  ( 1.767766952966368432, 186.2300000002184959, 8.767766952966368876 ) ) ;
#14371=CARTESIAN_POINT ( 'NONE',  ( -1.001898788273069663, 228.8297312643339296, 8.635702072933472806 ) ) ;
#14372=CARTESIAN_POINT ( 'NONE',  ( -1.864073305829632599, 228.0308260764439297, 6.328418323741104246 ) ) ;
#14377=CARTESIAN_POINT ( 'NONE',  ( -2.066987300000000971, 188.6499999989075036, 7.000000000000000000 ) ) ;
#14378=B_SPLINE_SURFACE_WITH_KNOTS ( 'NONE', 1, 3, ( 
 ( #8429, #2601, #3791, #6200, #13425, #12226, #3561, #1249, #7534, #1480, #9853, #12381, #219, #9701, #4846, #12072, #6125, #7459, #1325, #6358, #7318, #2446, #9930, #10960, #9621, #5000, #6275, #14702, #1400, #13343, #3637, #14460, #13266, #11115, #5077, #14781, #2365, #3867, #7233, #8666, #9779, #8512, #1170, #7310, #12150, #13497, #57, #11037, #6039, #8741, #4924, #10884, #14625, #3714, #8591, #2529, #7384, #11499, #13967, #11425, #15018, #12696, #4268, #5318, #2845, #6439, #7691, #6746, #3073, #4110, #6589, #1638, #5155, #10241, #12461, #1871, #5239, #12541, #13737, #13648, #6515, #15093, #10316, #14936, #2997, #293, #14857, #8902, #12616, #15169, #9133, #8980, #1714, #11348, #7923, #2763, #13809, #10085, #12766, #10010, #4026, #3944, #525, #7852, #447, #1562, #7770, #5394, #7616, #11271, #8818, #4188, #9059, #371, #10163, #2920, #13884, #1792, #6668, #602, #5474, #5704, #15327, #761, #11579, #1950, #8090, #4502, #14119, #12927, #11809, #2027, #6977, #14043, #4347, #9517, #5781, #14197, #674, #912, #9283, #3379, #5626, #6824, #11658, #3225, #15405, #10397, #10473, #2181, #8247, #6903, #11736, #3459, #4426, #9358, #839, #14269, #7052, #8167, #8005, #8325, #9437, #3304 ),
 ( #10548, #13004, #2263, #9205, #14350, #10629, #13164, #15491, #5550, #4587, #13082, #2106, #11887, #996, #5859, #10706, #15563, #4665, #15247, #3152, #12847, #1231, #13323, #7366, #7441, #5937, #9835, #12208, #40, #13556, #3850, #15728, #12131, #196, #9913, #6019, #7134, #6100, #4984, #3696, #10784, #11098, #15643, #8651, #10942, #13481, #8573, #11970, #4744, #2345, #2513, #2585, #8723, #2424, #12285, #1151, #6181, #13402, #5060, #1076, #14684, #4825, #9595, #1305, #11019, #119, #3619, #8496, #3774, #14605, #14438, #7214, #9681, #1385, #7293, #14766, #6260, #3541, #8412, #13247, #14520, #10860, #12052, #4906, #9763, #508, #13866, #11175, #10224, #10301, #2902, #7675, #1545, #5138, #5219, #12445, #1696, #6420, #15002, #7518, #12679, #4008, #1777, #10069, #354, #1621, #4092, #8962, #2978, #585, #13793, #6497, #15075, #6650, #12523, #14918, #8803, #8887, #9116, #5454, #11332, #7751, #13719, #12364, #12597, #14840, #4248, #7597, #2826, #429, #276, #5300, #6572, #11483, #11253, #5378, #2665, #1461, #10148, #11407, #15153, #6339, #4169, #9041, #7829, #9991, #3926, #13632, #2746, #5840, #4644, #3134, #7907, #9337, #893, #7988, #15227, #5685, #10532, #12983, #15387, #4411, #5764, #4331 ) ),
 .UNSPECIFIED., .F., .T., .F.,
 ( 2, 2 ),
 ( 4, 2, 2, 2, 2, 2, 2, 2, 2, 2, 2, 2, 2, 2, 2, 2, 2, 2, 2, 2, 2, 2, 2, 2, 2, 2, 2, 2, 2, 2, 2, 2, 2, 2, 2, 2, 2, 2, 2, 2, 2, 2, 2, 2, 2, 2, 2, 2, 2, 2, 2, 2, 2, 2, 2, 2, 2, 2, 2, 2, 2, 2, 2, 2, 2, 2, 2, 2, 2, 2, 2, 2, 2, 2, 2, 2, 2, 2, 2, 2, 2, 4 ),
 ( 0.000000000000000000, 1.000000000000000000 ),
 ( 0.0002080168337970193793, 0.0004025046291346534252, 0.0005969924244722874711, 0.0006942363221411045754, 0.0007914802198099215712, 0.0009859680151475555630, 0.001180455810485189772, 0.001277699708154006767, 0.001374943605822823763, 0.001472187503491640759, 0.001569431401160457755, 0.001763919196498091747, 0.001958406991835725738, 0.002055650889504542951, 0.002152894787173360164, 0.002347382582510994155, 0.002541870377848628147, 0.002639114275517445360, 0.002736358173186262139, 0.002930845968523896131, 0.003125333763861530122, 0.003222577661530346901, 0.003319821559199164114, 0.003417065456867981327, 0.003514309354536798539, 0.003708797149874432531, 0.003903284945212066523, 0.004097772740549700948, 0.004292260535887335374, 0.004486748331224968932, 0.004681236126562602490, 0.004875723921900236915, 0.005070211717237871341, 0.005264699512575504899, 0.005361943410244322111, 0.005459187307913138457, 0.005653675103250772882, 0.005848162898588407307, 0.005945406796257223653, 0.006042650693926040865, 0.006237138489263674423, 0.006431626284601308849, 0.006626114079938943274, 0.006820601875276577700, 0.007015089670614212125, 0.007112333568283028470, 0.007209577465951845683, 0.007404065261289479241, 0.007598553056627113667, 0.007695796954295930879, 0.007793040851964748092, 0.007890284749633564437, 0.007987528647302382517, 0.008182016442640016943, 0.008376504237977651368, 0.008473748135646467713, 0.008570992033315284059, 0.008765479828652918484, 0.008959967623990552910, 0.009057211521659369255, 0.009154455419328185600, 0.009348943214665820026, 0.009543431010003454451, 0.009640674907672272531, 0.009737918805341088876, 0.009835162703009905222, 0.009932406600678723302, 0.01012689439601635599, 0.01032138219135399042, 0.01041862608902280676, 0.01051586998669162484, 0.01071035778202925753, 0.01090484557736689196, 0.01109933337270452638, 0.01129382116804216081, 0.01148830896337979524, 0.01168279675871742793, 0.01187728455405506235, 0.01207177234939269678, 0.01226626014473032947, 0.01246074794006796389, 0.01265523573540559832 ),
 .UNSPECIFIED. ) ;
#14379=CARTESIAN_POINT ( 'NONE',  ( 1.461580736456472795, 184.9499999989075150, 8.461580736456474128 ) ) ;
#14387=CARTESIAN_POINT ( 'NONE',  ( 5.999999999999999112, 222.7460571280668091, 12.08513476933103448 ) ) ;
#14389=CARTESIAN_POINT ( 'NONE',  ( -1.461580736456473906, 186.3499999989074922, 8.461580736456474128 ) ) ;
#14393=CARTESIAN_POINT ( 'NONE',  ( 1.423015351387224570E-16, 184.1999999999999886, 4.500000000000000000 ) ) ;
#14409=CARTESIAN_POINT ( 'NONE',  ( 2.066987299999999639, 188.4999999989074979, 6.143825827087054492 ) ) ;
#14415=CARTESIAN_POINT ( 'NONE',  ( -0.4900172623563870955, 226.3376062179358996, 4.523300904952406221 ) ) ;
#14425=EDGE_CURVE ( 'NONE', #13467, #10770, #11452, .T. ) ;
#14437=CARTESIAN_POINT ( 'NONE',  ( 1.035533905932737753, 187.2499999978151095, 4.500000000000000888 ) ) ;
#14438=CARTESIAN_POINT ( 'NONE',  ( 1.458867243353906273, 226.4466662005724800, 4.844797864602860216 ) ) ;
#14452=CARTESIAN_POINT ( 'NONE',  ( -2.776549226834668538, 226.9241846788892190, 6.251816468300146035 ) ) ;
#14455=CARTESIAN_POINT ( 'NONE',  ( 1.035533905932738197, 188.5800000002184902, 9.500000000000003553 ) ) ;
#14457=EDGE_CURVE ( 'NONE', #2406, #12251, #10, .T. ) ;
#14458=CARTESIAN_POINT ( 'NONE',  ( -0.4523656679209748233, 227.6256624317788635, 5.158282608927489576 ) ) ;
#14459=STYLED_ITEM ( 'NONE', ( #926 ), #8222 ) ;
#14460=CARTESIAN_POINT ( 'NONE',  ( 1.785787022451674089, 228.5490719641819908, 7.825142006337427070 ) ) ;
#14464=EDGE_CURVE ( 'NONE', #3723, #1738, #9941, .T. ) ;
#14467=CARTESIAN_POINT ( 'NONE',  ( 0.8561741729129461742, 186.4999999989075263, 9.066987300000000971 ) ) ;
#14476=CARTESIAN_POINT ( 'NONE',  ( 5.082197683525802034E-17, 185.2499999989074979, 4.933012699999999029 ) ) ;
#14478=CARTESIAN_POINT ( 'NONE',  ( 0.2265647620681634500, 189.0000000000732996, 9.493607781726925765 ) ) ;
#14480=CARTESIAN_POINT ( 'NONE',  ( -1.767766952966369098, 184.2999999999999829, 5.232233047033630235 ) ) ;
#14494=CARTESIAN_POINT ( 'NONE',  ( -2.066987300000000971, 188.7999999989075093, 6.143825827087054492 ) ) ;
#14501=CARTESIAN_POINT ( 'NONE',  ( -1.707413668510289861, 226.4963546398602148, 4.991255295473766118 ) ) ;
#14519=CARTESIAN_POINT ( 'NONE',  ( -2.500000000000000444, 187.4999999978150527, 7.000000000000000000 ) ) ;
#14520=CARTESIAN_POINT ( 'NONE',  ( 0.3927937339364459546, 226.3329534510998542, 4.509583726312986762 ) ) ;
#14529=LINE ( 'NONE', #9690, #15533 ) ;
#14537=CARTESIAN_POINT ( 'NONE',  ( 1.035533905932737753, 188.8800000002185016, 4.500000000000000888 ) ) ;
#14544=CARTESIAN_POINT ( 'NONE',  ( 0.8561741729129456191, 187.5999999989074922, 4.933012699999999029 ) ) ;
#14545=CARTESIAN_POINT ( 'NONE',  ( 5.082197683525802034E-17, 185.2499999989074979, 4.933012699999999029 ) ) ;
#14547=EDGE_LOOP ( 'NONE', ( #7657, #5281, #7100, #9539, #1192, #5823 ) ) ;
#14549=DIRECTION ( 'NONE',  ( 0.02819803676014390886, 0.000000000000000000, -0.9996023563011813273 ) ) ;
#14554=CARTESIAN_POINT ( 'NONE',  ( 1.461580736456473240, 188.3499999989074922, 5.538419263543526760 ) ) ;
#14573=CARTESIAN_POINT ( 'NONE',  ( -2.066987300000000083, 187.2499999989075263, 7.000000000000000000 ) ) ;
#14581=CARTESIAN_POINT ( 'NONE',  ( -2.381136272098726803, 226.7019369474745361, 5.597090573316407358 ) ) ;
#14590=CARTESIAN_POINT ( 'NONE',  ( 2.500000000000000444, 185.5500000000000114, 8.035533905932739529 ) ) ;
#14591=ADVANCED_FACE ( 'NONE', ( #3895 ), #12487, .F. ) ;
#14596=DIRECTION ( 'NONE',  ( -6.123233995736766036E-17, 1.000000000000000000, 0.000000000000000000 ) ) ;
#14602=CARTESIAN_POINT ( 'NONE',  ( -0.05144838531732269515, 189.9979265964238948, 9.435094243585153251 ) ) ;
#14604=CARTESIAN_POINT ( 'NONE',  ( -2.500000000000000888, 189.1499999978150868, 8.035533905932737753 ) ) ;
#14605=CARTESIAN_POINT ( 'NONE',  ( 1.501755279530002651, 226.4544816774725575, 4.867834892302488115 ) ) ;
#14608=CARTESIAN_POINT ( 'NONE',  ( -0.9261565315117185060, 190.0733590023996555, 4.344097979414469179 ) ) ;
#14622=DIRECTION ( 'NONE',  ( -1.000000000000000000, 0.000000000000000000, 0.000000000000000000 ) ) ;
#14623=CARTESIAN_POINT ( 'NONE',  ( 2.500000000000000000, 188.6800000002185129, 8.035533905932739529 ) ) ;
#14625=CARTESIAN_POINT ( 'NONE',  ( 1.924362066950147332, 228.0923243445923276, 6.506028829785237555 ) ) ;
#14629=CARTESIAN_POINT ( 'NONE',  ( -2.066987300000000971, 186.9999999989074979, 6.143825827087054492 ) ) ;
#14630=CARTESIAN_POINT ( 'NONE',  ( 0.8561741729129456191, 187.5999999989074922, 4.933012699999999029 ) ) ;
#14632=CIRCLE ( 'NONE', #7763, 2.500000000000000444 ) ;
#14633=CARTESIAN_POINT ( 'NONE',  ( 1.461580736456473018, 185.3499999989075206, 5.538419263543527649 ) ) ;
#14639=CARTESIAN_POINT ( 'NONE',  ( 5.999999999999999112, 194.5935680195190116, 12.11154058223188379 ) ) ;
#14642=CARTESIAN_POINT ( 'NONE',  ( 0.1286560605739063556, 189.6973959400375520, 10.39407231488526762 ) ) ;
#14659=CARTESIAN_POINT ( 'NONE',  ( -2.066987300000000971, 187.2999999989075661, 7.856174172912944620 ) ) ;
#14666=CARTESIAN_POINT ( 'NONE',  ( -2.999982576790682476, 227.2579145021288696, 7.234552515775640735 ) ) ;
#14668=FACE_OUTER_BOUND ( 'NONE', #12854, .T. ) ;
#14673=CARTESIAN_POINT ( 'NONE',  ( 0.000000000000000000, 189.6977690162252657, 10.38967773564543862 ) ) ;
#14677=FACE_OUTER_BOUND ( 'NONE', #3757, .T. ) ;
#14683=CARTESIAN_POINT ( 'NONE',  ( 1.035533905932738197, 189.3499999978150754, 9.500000000000003553 ) ) ;
#14684=CARTESIAN_POINT ( 'NONE',  ( 2.383228694455616914, 226.7027912316577556, 5.599607710487992662 ) ) ;
#14686=CARTESIAN_POINT ( 'NONE',  ( -2.909494418114037195, 189.9181870229658671, 6.441359701375095170 ) ) ;
#14690=EDGE_CURVE ( 'NONE', #5418, #7973, #1665, .T. ) ;
#14692=CARTESIAN_POINT ( 'NONE',  ( 1.991469598915552641, 226.5678560613478680, 5.201980668966470489 ) ) ;
#14699=CYLINDRICAL_SURFACE ( 'NONE', #1881, 2.500000000000000444 ) ;
#14700=CARTESIAN_POINT ( 'NONE',  ( -1.767766952966369098, 184.2999999999999829, 5.232233047033630235 ) ) ;
#14702=CARTESIAN_POINT ( 'NONE',  ( 1.618192118698865700, 228.6399984490590214, 8.087742880769061671 ) ) ;
#14710=CARTESIAN_POINT ( 'NONE',  ( -0.8561741729129457301, 186.8999999989075036, 4.933012699999999029 ) ) ;
#14718=CARTESIAN_POINT ( 'NONE',  ( 5.999999999999999112, 187.9952603975225429, 3.440894205938198613 ) ) ;
#14719=CARTESIAN_POINT ( 'NONE',  ( -1.768703179866833342, 189.0000639513403939, 5.233169770031948609 ) ) ;
#14724=DIRECTION ( 'NONE',  ( -1.000000000000000000, 0.000000000000000000, 0.000000000000000000 ) ) ;
#14747=CARTESIAN_POINT ( 'NONE',  ( -2.548643141829932901, 227.7997363639018147, 8.829041127271985090 ) ) ;
#14751=ORIENTED_EDGE ( 'NONE', *, *, #15149, .F. ) ;
#14753=CARTESIAN_POINT ( 'NONE',  ( 2.328196544889883590, 189.0000000000000284, 6.072157969751945217 ) ) ;
#14759=CARTESIAN_POINT ( 'NONE',  ( 2.500000000000000444, 186.2999999978150356, 7.000000000000000000 ) ) ;
#14764=CARTESIAN_POINT ( 'NONE',  ( 1.767766952966368432, 187.0699999975965397, 8.767766952966368876 ) ) ;
#14765=CARTESIAN_POINT ( 'NONE',  ( -0.8231351400649619121, 227.6668932001845462, 5.277359419731677548 ) ) ;
#14766=CARTESIAN_POINT ( 'NONE',  ( 0.8272382227408706656, 226.3624115040579738, 4.596429122765971265 ) ) ;
#14767=CARTESIAN_POINT ( 'NONE',  ( -2.495860339748324108, 189.0000000026251712, 6.620890110190097211 ) ) ;
#14773=CARTESIAN_POINT ( 'NONE',  ( -0.07717340183324797320, 189.6978550888158281, 10.38866401756451552 ) ) ;
#14774=CARTESIAN_POINT ( 'NONE',  ( 2.982602392329962715, 227.1840276311630475, 7.016963325779705052 ) ) ;
#14779=CARTESIAN_POINT ( 'NONE',  ( 1.767766952966369320, 184.9000000000000057, 5.232233047033630235 ) ) ;
#14781=CARTESIAN_POINT ( 'NONE',  ( 1.884974866327016940, 228.4701649684375866, 7.597254102066775872 ) ) ;
#14786=CARTESIAN_POINT ( 'NONE',  ( 2.066987300000000083, 189.0499999989075093, 7.000000000000000000 ) ) ;
#14787=CARTESIAN_POINT ( 'NONE',  ( 2.500000000000000444, 187.1499999978150584, 5.964466094067262247 ) ) ;
#14788=CARTESIAN_POINT ( 'NONE',  ( 2.066987300000000083, 186.0999999989075206, 6.143825827087054492 ) ) ;
#14794=CARTESIAN_POINT ( 'NONE',  ( -5.999999999999999112, 187.2933328889893403, 9.583808270834989429 ) ) ;
#14795=CARTESIAN_POINT ( 'NONE',  ( -2.445702039570965436, 189.0000000000000284, 6.417294754563008574 ) ) ;
#14800=CARTESIAN_POINT ( 'NONE',  ( 2.900815891035680938, 189.8415453012541718, 8.113821064254620907 ) ) ;
#14804=ORIENTED_EDGE ( 'NONE', *, *, #2925, .T. ) ;
#14805=CARTESIAN_POINT ( 'NONE',  ( 2.066987299999999639, 188.4499999989075150, 7.000000000000000000 ) ) ;
#14809=AXIS2_PLACEMENT_3D ( 'NONE', #3069, #2993, #12761 ) ;
#14814=CARTESIAN_POINT ( 'NONE',  ( -2.367857196298859268, 227.8856709934939317, 9.081849937883657020 ) ) ;
#14823=CARTESIAN_POINT ( 'NONE',  ( -1.978640506925948062, 228.0159251728749155, 9.464911921216582869 ) ) ;
#14826=ORIENTED_EDGE ( 'NONE', *, *, #8880, .T. ) ;
#14828=CARTESIAN_POINT ( 'NONE',  ( 0.7947751898797416059, 188.9999999999999716, 4.622669033327397869 ) ) ;
#14834=CARTESIAN_POINT ( 'NONE',  ( 2.500000000000000444, 185.5499999978150640, 5.964466094067262247 ) ) ;
#14838=CARTESIAN_POINT ( 'NONE',  ( 2.500000000000000444, 186.4199999975966193, 5.964466094067262247 ) ) ;
#14839=CARTESIAN_POINT ( 'NONE',  ( -1.690976820968455474, 227.9165037442230926, 5.998248907768082283 ) ) ;
#14840=CARTESIAN_POINT ( 'NONE',  ( -3.000008639299222235, 227.3051114066062155, 7.373492455173472848 ) ) ;
#14843=CARTESIAN_POINT ( 'NONE',  ( -2.694542719975550948, 189.3631562369849064, 5.701170958452144610 ) ) ;
#14844=ORIENTED_EDGE ( 'NONE', *, *, #5021, .T. ) ;
#14849=CARTESIAN_POINT ( 'NONE',  ( 1.170086215019673359, 228.1786594689324659, 9.943436085668160729 ) ) ;
#14854=CARTESIAN_POINT ( 'NONE',  ( 1.035533905932738197, 187.0499999999999829, 9.500000000000003553 ) ) ;
#14857=CARTESIAN_POINT ( 'NONE',  ( -0.3251550031287174236, 227.6173728764936186, 5.134341900458684549 ) ) ;
#14861=CARTESIAN_POINT ( 'NONE',  ( -1.035533905932737753, 184.2500000000000000, 4.500000000000000888 ) ) ;
#14864=CARTESIAN_POINT ( 'NONE',  ( -1.461580736456473462, 188.9499999989075150, 8.461580736456472351 ) ) ;
#14868=CARTESIAN_POINT ( 'NONE',  ( -5.999999999999999112, 188.6555110544239824, 3.692234042171783415 ) ) ;
#14871=CARTESIAN_POINT ( 'NONE',  ( 1.934702460432737414, 190.0213251105361962, 4.917537802262033964 ) ) ;
#14879=CARTESIAN_POINT ( 'NONE',  ( -2.066987300000000971, 187.2999999989075661, 7.856174172912944620 ) ) ;
#14886=DIRECTION ( 'NONE',  ( -6.123233995736766036E-17, 1.000000000000000000, 0.000000000000000000 ) ) ;
#14887=VERTEX_POINT ( 'NONE', #15275 ) ;
#14891=CARTESIAN_POINT ( 'NONE',  ( -0.07717340183324797320, 189.6978550888158281, 10.38866401756451552 ) ) ;
#14909=CARTESIAN_POINT ( 'NONE',  ( -2.500000000000000444, 187.5499999978150356, 8.035533905932737753 ) ) ;
#14910=CARTESIAN_POINT ( 'NONE',  ( -1.767766952966369320, 186.5999999978150754, 5.232233047033630235 ) ) ;
#14916=CARTESIAN_POINT ( 'NONE',  ( -1.767766952966369320, 187.4699999975965454, 5.232233047033630235 ) ) ;
#14917=CARTESIAN_POINT ( 'NONE',  ( -1.813734975128623139, 228.5291423394705532, 7.767584113458720019 ) ) ;
#14918=CARTESIAN_POINT ( 'NONE',  ( -2.809196860006122787, 226.9495188873497966, 6.326437523183426670 ) ) ;
#14919=CARTESIAN_POINT ( 'NONE',  ( -1.819594887494103475, 189.1119032262050439, 9.571239929234401700 ) ) ;
#14926=CARTESIAN_POINT ( 'NONE',  ( 2.839005933515748925, 227.6017802382847037, 8.246656694154813394 ) ) ;
#14932=CARTESIAN_POINT ( 'NONE',  ( 2.500000000000000444, 187.2500000000000000, 5.964466094067262247 ) ) ;
#14935=AXIS2_PLACEMENT_3D ( 'NONE', #3766, #3688, #8643 ) ;
#14936=CARTESIAN_POINT ( 'NONE',  ( -0.06647456835015956578, 227.6089819833846093, 5.110108522575333545 ) ) ;
#14939=CARTESIAN_POINT ( 'NONE',  ( -4.946672411965113980E-16, 184.5999999999999943, 9.500000000000001776 ) ) ;
#14942=CARTESIAN_POINT ( 'NONE',  ( 1.461580736456472795, 188.5499999989075093, 5.538419263543527649 ) ) ;
#14949=CARTESIAN_POINT ( 'NONE',  ( 0.000000000000000000, 186.5669965222008386, 9.317226423031119253 ) ) ;
#14952=CARTESIAN_POINT ( 'NONE',  ( 2.252723718013021958, 189.7744973743064918, 9.355516826583022194 ) ) ;
#14962=CARTESIAN_POINT ( 'NONE',  ( -1.461580736456473018, 186.3499999989075206, 5.538419263543527649 ) ) ;
#14963=( BOUNDED_CURVE ( )  B_SPLINE_CURVE ( 2, ( #10061, #14909, #4163, #2737, #15146, #3049, #1844, #5131, #3918 ),
 .UNSPECIFIED., .F., .F. ) 
 B_SPLINE_CURVE_WITH_KNOTS ( ( 3, 2, 2, 2, 3 ),
 ( 0.5000000000000000000, 0.5178571428571429047, 0.5357142857142856984, 0.5535714285714286031, 0.5714285714285713969 ),
 .UNSPECIFIED. ) 
 CURVE ( )  GEOMETRIC_REPRESENTATION_ITEM ( )  RATIONAL_B_SPLINE_CURVE ( ( 1.000000000000000000, 0.9238795325112867385, 1.000000000000000000, 0.9238795325112867385, 1.000000000000000000, 0.9238795325112867385, 1.000000000000000000, 0.9238795325112867385, 1.000000000000000000 ) ) 
 REPRESENTATION_ITEM ( '' )  );
#14964=ORIENTED_EDGE ( 'NONE', *, *, #15367, .F. ) ;
#14974=( BOUNDED_SURFACE ( )  B_SPLINE_SURFACE ( 1, 2, ( 
 ( #10641, #5639, #3239, #777, #12859, #9295, #11904, #5720, #3164, #928, #1013, #9452, #1886, #4363, #13099, #11592, #5875, #8262, #15503, #4601, #2044, #11678, #1964, #7942, #8022, #4441, #4518, #14134, #6917, #8184, #11751, #13021, #15261, #5566, #10722, #2120, #6992, #9223, #4682, #15580, #11821, #5795, #14286, #3393, #2198, #9533, #14370, #8426, #9850, #11035, #12148, #11987, #12300, #1397, #11112, #6273, #133, #217, #55, #15658, #5076, #1322, #2281, #13263, #4922, #12068, #9928, #7230, #7455, #3788, #8859, #3558, #2598, #3474, #8344, #8588, #13182, #2526, #4998, #3635, #7150, #1168, #10957, #1092, #4843, #5955, #10799, #4759, #9616, #13341, #9699, #3712, #8664, #14455, #9777, #14623, #2362, #6036, #10882, #14537, #6198 ),
 ( #8511, #2444, #1247, #7308, #12223, #6122, #14700, #13423, #7382, #13495, #8738, #7850, #15092, #6587, #11423, #8900, #2761, #3941, #14779, #5153, #11269, #7689, #1560, #369, #15017, #5236, #10162, #1478, #7532, #12694, #8979, #1635, #3865, #11498, #1791, #2918, #12459, #13645, #4109, #12539, #13883, #13570, #8816, #5393, #523, #6513, #12378, #6667, #601, #5472, #2680, #10240, #6356, #11346, #11192, #291, #12615, #10008, #7613, #444, #6437, #14854, #10082, #2996, #4186, #14932, #4024, #13735, #2843, #5317, #13808, #7769, #1711, #9058, #10471, #8246, #8003, #2025, #3071, #6822, #995, #2179, #7922, #4267, #4425, #759, #10547, #10627, #9132, #11734, #5702, #6744, #673, #7051, #3151, #15325, #3378, #11807, #11657, #9355, #13080 ),
 ( #9281, #14268, #9436, #837, #11885, #12846, #9203, #10315, #13964, #6975, #5780, #15168, #14118, #15404, #1949, #5624, #3223, #911, #14196, #5548, #8087, #6902, #12926, #12764, #15490, #4501, #4586, #1870, #3302, #8165, #10396, #13003, #11577, #15245, #2104, #4345, #14042, #10705, #39, #2262, #7440, #10783, #8411, #3540, #3457, #13246, #2344, #3695, #7292, #4905, #13163, #14437, #1303, #13480, #4983, #9834, #14519, #2423, #15641, #12051, #8572, #13401, #7212, #2511, #6018, #5936, #15562, #1230, #7365, #4743, #9680, #1150, #10941, #9593, #10859, #1075, #15726, #6180, #3618, #11969, #4824, #13322, #8495, #12129, #2584, #6099, #9762, #12284, #11018, #14604, #12207, #14348, #118, #14683, #3773, #8650, #5858, #4664, #9516, #8324, #7133 ),
 ( #12443, #6337, #1459, #8721, #2744, #6258, #2976, #11096, #7673, #1543, #9910, #12594, #11251, #5375, #506, #12520, #10222, #9989, #273, #1383, #194, #13791, #1694, #15073, #6418, #1619, #8801, #4090, #13630, #5136, #3848, #3924, #11173, #14838, #7595, #8885, #4006, #5057, #9039, #4167, #8960, #13864, #13717, #13554, #7827, #14999, #14764, #352, #2824, #5217, #2663, #10067, #7516, #6570, #14916, #6495, #12362, #11330, #427, #5298, #10146, #2900, #7749, #11405, #10604, #10375, #4409, #5452, #9186, #3358, #4565, #10299, #6648, #6803, #3132, #12907, #12981, #11480, #14098, #8065, #9114, #3054, #9415, #5527, #1929, #5761, #14176, #14026, #11715, #15463, #7985, #1851, #7905, #583, #11558, #6725, #15225, #4328, #3206, #12677, #15151 ) ),
 .UNSPECIFIED., .F., .F., .F. ) 
 B_SPLINE_SURFACE_WITH_KNOTS ( ( 2, 1, 1, 2 ),
 ( 3, 2, 2, 2, 2, 2, 2, 2, 2, 2, 2, 2, 2, 2, 2, 2, 2, 2, 2, 2, 2, 2, 2, 2, 2, 2, 2, 2, 2, 2, 2, 2, 2, 2, 2, 2, 2, 2, 2, 2, 2, 2, 2, 2, 2, 2, 2, 2, 2, 2, 3 ),
 ( -0.1000000000000000056, 0.000000000000000000, 1.000000000000000000, 1.100000000000000089 ),
 ( 0.000000000000000000, 0.01785714285714285615, 0.03571428571428571230, 0.05357142857142856845, 0.07142857142857142461, 0.08928571428571428770, 0.1071428571428571369, 0.1250000000000000000, 0.1428571428571428492, 0.1607142857142857262, 0.1785714285714285754, 0.1964285714285714246, 0.2142857142857142738, 0.2321428571428571508, 0.2500000000000000000, 0.2678571428571428492, 0.2857142857142856984, 0.3035714285714285476, 0.3214285714285714524, 0.3392857142857143016, 0.3571428571428571508, 0.3750000000000000000, 0.3928571428571428492, 0.4107142857142856984, 0.4285714285714285476, 0.4464285714285714524, 0.4642857142857143016, 0.4821428571428571508, 0.5000000000000000000, 0.5178571428571429047, 0.5357142857142856984, 0.5535714285714286031, 0.5714285714285713969, 0.5892857142857143016, 0.6071428571428570953, 0.6250000000000000000, 0.6428571428571429047, 0.6607142857142856984, 0.6785714285714286031, 0.6964285714285713969, 0.7142857142857143016, 0.7321428571428570953, 0.7500000000000000000, 0.7678571428571429047, 0.7857142857142856984, 0.8035714285714286031, 0.8214285714285713969, 0.8392857142857143016, 0.8571428571428570953, 0.8750000000000000000, 0.8928571428571429047 ),
 .UNSPECIFIED. ) 
 GEOMETRIC_REPRESENTATION_ITEM ( )  RATIONAL_B_SPLINE_SURFACE ( (
 ( 1.000000000000000000, 0.9238795325112867385, 1.000000000000000000, 0.9238795325112867385, 1.000000000000000000, 0.9238795325112867385, 1.000000000000000000, 0.9238795325112867385, 1.000000000000000000, 0.9238795325112867385, 1.000000000000000000, 0.9238795325112867385, 1.000000000000000000, 0.9238795325112867385, 1.000000000000000000, 0.9238795325112867385, 1.000000000000000000, 0.9238795325112867385, 1.000000000000000000, 0.9238795325112867385, 1.000000000000000000, 0.9238795325112867385, 1.000000000000000000, 0.9238795325112867385, 1.000000000000000000, 0.9238795325112867385, 1.000000000000000000, 0.9238795325112867385, 1.000000000000000000, 0.9238795325112867385, 1.000000000000000000, 0.9238795325112867385, 1.000000000000000000, 0.9238795325112867385, 1.000000000000000000, 0.9238795325112867385, 1.000000000000000000, 0.9238795325112867385, 1.000000000000000000, 0.9238795325112867385, 1.000000000000000000, 0.9238795325112867385, 1.000000000000000000, 0.9238795325112867385, 1.000000000000000000, 0.9238795325112867385, 1.000000000000000000, 0.9238795325112867385, 1.000000000000000000, 0.9238795325112867385, 1.000000000000000000, 0.9238795325112867385, 1.000000000000000000, 0.9238795325112867385, 1.000000000000000000, 0.9238795325112867385, 1.000000000000000000, 0.9238795325112867385, 1.000000000000000000, 0.9238795325112867385, 1.000000000000000000, 0.9238795325112867385, 1.000000000000000000, 0.9238795325112867385, 1.000000000000000000, 0.9238795325112867385, 1.000000000000000000, 0.9238795325112867385, 1.000000000000000000, 0.9238795325112867385, 1.000000000000000000, 0.9238795325112867385, 1.000000000000000000, 0.9238795325112867385, 1.000000000000000000, 0.9238795325112867385, 1.000000000000000000, 0.9238795325112867385, 1.000000000000000000, 0.9238795325112867385, 1.000000000000000000, 0.9238795325112867385, 1.000000000000000000, 0.9238795325112867385, 1.000000000000000000, 0.9238795325112867385, 1.000000000000000000, 0.9238795325112867385, 1.000000000000000000, 0.9238795325112867385, 1.000000000000000000, 0.9238795325112867385, 1.000000000000000000, 0.9238795325112867385, 1.000000000000000000, 0.9238795325112867385, 1.000000000000000000, 0.9238795325112867385, 1.000000000000000000, 0.9238795325112867385, 1.000000000000000000),
 ( 1.000000000000000000, 0.9238795325112867385, 1.000000000000000000, 0.9238795325112867385, 1.000000000000000000, 0.9238795325112867385, 1.000000000000000000, 0.9238795325112867385, 1.000000000000000000, 0.9238795325112867385, 1.000000000000000000, 0.9238795325112867385, 1.000000000000000000, 0.9238795325112867385, 1.000000000000000000, 0.9238795325112867385, 1.000000000000000000, 0.9238795325112867385, 1.000000000000000000, 0.9238795325112867385, 1.000000000000000000, 0.9238795325112867385, 1.000000000000000000, 0.9238795325112867385, 1.000000000000000000, 0.9238795325112867385, 1.000000000000000000, 0.9238795325112867385, 1.000000000000000000, 0.9238795325112867385, 1.000000000000000000, 0.9238795325112867385, 1.000000000000000000, 0.9238795325112867385, 1.000000000000000000, 0.9238795325112867385, 1.000000000000000000, 0.9238795325112867385, 1.000000000000000000, 0.9238795325112867385, 1.000000000000000000, 0.9238795325112867385, 1.000000000000000000, 0.9238795325112867385, 1.000000000000000000, 0.9238795325112867385, 1.000000000000000000, 0.9238795325112867385, 1.000000000000000000, 0.9238795325112867385, 1.000000000000000000, 0.9238795325112867385, 1.000000000000000000, 0.9238795325112867385, 1.000000000000000000, 0.9238795325112867385, 1.000000000000000000, 0.9238795325112867385, 1.000000000000000000, 0.9238795325112867385, 1.000000000000000000, 0.9238795325112867385, 1.000000000000000000, 0.9238795325112867385, 1.000000000000000000, 0.9238795325112867385, 1.000000000000000000, 0.9238795325112867385, 1.000000000000000000, 0.9238795325112867385, 1.000000000000000000, 0.9238795325112867385, 1.000000000000000000, 0.9238795325112867385, 1.000000000000000000, 0.9238795325112867385, 1.000000000000000000, 0.9238795325112867385, 1.000000000000000000, 0.9238795325112867385, 1.000000000000000000, 0.9238795325112867385, 1.000000000000000000, 0.9238795325112867385, 1.000000000000000000, 0.9238795325112867385, 1.000000000000000000, 0.9238795325112867385, 1.000000000000000000, 0.9238795325112867385, 1.000000000000000000, 0.9238795325112867385, 1.000000000000000000, 0.9238795325112867385, 1.000000000000000000, 0.9238795325112867385, 1.000000000000000000, 0.9238795325112867385, 1.000000000000000000, 0.9238795325112867385, 1.000000000000000000),
 ( 1.000000000000000000, 0.9238795325112867385, 1.000000000000000000, 0.9238795325112867385, 1.000000000000000000, 0.9238795325112867385, 1.000000000000000000, 0.9238795325112867385, 1.000000000000000000, 0.9238795325112867385, 1.000000000000000000, 0.9238795325112867385, 1.000000000000000000, 0.9238795325112867385, 1.000000000000000000, 0.9238795325112867385, 1.000000000000000000, 0.9238795325112867385, 1.000000000000000000, 0.9238795325112867385, 1.000000000000000000, 0.9238795325112867385, 1.000000000000000000, 0.9238795325112867385, 1.000000000000000000, 0.9238795325112867385, 1.000000000000000000, 0.9238795325112867385, 1.000000000000000000, 0.9238795325112867385, 1.000000000000000000, 0.9238795325112867385, 1.000000000000000000, 0.9238795325112867385, 1.000000000000000000, 0.9238795325112867385, 1.000000000000000000, 0.9238795325112867385, 1.000000000000000000, 0.9238795325112867385, 1.000000000000000000, 0.9238795325112867385, 1.000000000000000000, 0.9238795325112867385, 1.000000000000000000, 0.9238795325112867385, 1.000000000000000000, 0.9238795325112867385, 1.000000000000000000, 0.9238795325112867385, 1.000000000000000000, 0.9238795325112867385, 1.000000000000000000, 0.9238795325112867385, 1.000000000000000000, 0.9238795325112867385, 1.000000000000000000, 0.9238795325112867385, 1.000000000000000000, 0.9238795325112867385, 1.000000000000000000, 0.9238795325112867385, 1.000000000000000000, 0.9238795325112867385, 1.000000000000000000, 0.9238795325112867385, 1.000000000000000000, 0.9238795325112867385, 1.000000000000000000, 0.9238795325112867385, 1.000000000000000000, 0.9238795325112867385, 1.000000000000000000, 0.9238795325112867385, 1.000000000000000000, 0.9238795325112867385, 1.000000000000000000, 0.9238795325112867385, 1.000000000000000000, 0.9238795325112867385, 1.000000000000000000, 0.9238795325112867385, 1.000000000000000000, 0.9238795325112867385, 1.000000000000000000, 0.9238795325112867385, 1.000000000000000000, 0.9238795325112867385, 1.000000000000000000, 0.9238795325112867385, 1.000000000000000000, 0.9238795325112867385, 1.000000000000000000, 0.9238795325112867385, 1.000000000000000000, 0.9238795325112867385, 1.000000000000000000, 0.9238795325112867385, 1.000000000000000000, 0.9238795325112867385, 1.000000000000000000),
 ( 1.000000000000000000, 0.9238795325112867385, 1.000000000000000000, 0.9238795325112867385, 1.000000000000000000, 0.9238795325112867385, 1.000000000000000000, 0.9238795325112867385, 1.000000000000000000, 0.9238795325112867385, 1.000000000000000000, 0.9238795325112867385, 1.000000000000000000, 0.9238795325112867385, 1.000000000000000000, 0.9238795325112867385, 1.000000000000000000, 0.9238795325112867385, 1.000000000000000000, 0.9238795325112867385, 1.000000000000000000, 0.9238795325112867385, 1.000000000000000000, 0.9238795325112867385, 1.000000000000000000, 0.9238795325112867385, 1.000000000000000000, 0.9238795325112867385, 1.000000000000000000, 0.9238795325112867385, 1.000000000000000000, 0.9238795325112867385, 1.000000000000000000, 0.9238795325112867385, 1.000000000000000000, 0.9238795325112867385, 1.000000000000000000, 0.9238795325112867385, 1.000000000000000000, 0.9238795325112867385, 1.000000000000000000, 0.9238795325112867385, 1.000000000000000000, 0.9238795325112867385, 1.000000000000000000, 0.9238795325112867385, 1.000000000000000000, 0.9238795325112867385, 1.000000000000000000, 0.9238795325112867385, 1.000000000000000000, 0.9238795325112867385, 1.000000000000000000, 0.9238795325112867385, 1.000000000000000000, 0.9238795325112867385, 1.000000000000000000, 0.9238795325112867385, 1.000000000000000000, 0.9238795325112867385, 1.000000000000000000, 0.9238795325112867385, 1.000000000000000000, 0.9238795325112867385, 1.000000000000000000, 0.9238795325112867385, 1.000000000000000000, 0.9238795325112867385, 1.000000000000000000, 0.9238795325112867385, 1.000000000000000000, 0.9238795325112867385, 1.000000000000000000, 0.9238795325112867385, 1.000000000000000000, 0.9238795325112867385, 1.000000000000000000, 0.9238795325112867385, 1.000000000000000000, 0.9238795325112867385, 1.000000000000000000, 0.9238795325112867385, 1.000000000000000000, 0.9238795325112867385, 1.000000000000000000, 0.9238795325112867385, 1.000000000000000000, 0.9238795325112867385, 1.000000000000000000, 0.9238795325112867385, 1.000000000000000000, 0.9238795325112867385, 1.000000000000000000, 0.9238795325112867385, 1.000000000000000000, 0.9238795325112867385, 1.000000000000000000, 0.9238795325112867385, 1.000000000000000000, 0.9238795325112867385, 1.000000000000000000) ) ) 
 REPRESENTATION_ITEM ( '' )  SURFACE ( )  );
#14977=CARTESIAN_POINT ( 'NONE',  ( -1.035533905932739751, 186.9500000000000171, 9.500000000000000000 ) ) ;
#14980=CARTESIAN_POINT ( 'NONE',  ( -2.500000000000003109, 186.6499999978150299, 5.964466094067263136 ) ) ;
#14982=COLOUR_RGB ( '', 0.72549020, 0.75294118, 0.79215686) ;
#14993=CARTESIAN_POINT ( 'NONE',  ( 2.500000000000000444, 186.3499999978150754, 5.964466094067262247 ) ) ;
#14999=CARTESIAN_POINT ( 'NONE',  ( 1.035533905932738197, 187.0199999975965568, 9.500000000000003553 ) ) ;
#15000=CARTESIAN_POINT ( 'NONE',  ( 1.326034168411047265, 228.1562120337857777, 9.877435289762864556 ) ) ;
#15002=CARTESIAN_POINT ( 'NONE',  ( -1.747606509155581689, 226.5054486174500994, 5.018058692477180394 ) ) ;
#15004=CARTESIAN_POINT ( 'NONE',  ( -0.8150890167390612007, 189.0566948412773343, 10.07644837850013531 ) ) ;
#15011=CARTESIAN_POINT ( 'NONE',  ( 2.774089264892111384, 227.6570220514033167, 8.409174098727280722 ) ) ;
#15017=CARTESIAN_POINT ( 'NONE',  ( -2.500000000000000444, 185.2000000000000171, 7.000000000000000000 ) ) ;
#15018=CARTESIAN_POINT ( 'NONE',  ( 1.581415667291661276, 227.8641612386227848, 5.847080766174051369 ) ) ;
#15019=FACE_OUTER_BOUND ( 'NONE', #6848, .T. ) ;
#15022=CARTESIAN_POINT ( 'NONE',  ( -1.461580736456473906, 188.7499999989075263, 8.461580736456474128 ) ) ;
#15024=CARTESIAN_POINT ( 'NONE',  ( 0.8561741729129455081, 188.5999999989074922, 4.933012699999999029 ) ) ;
#15027=CARTESIAN_POINT ( 'NONE',  ( -2.500000000000000444, 186.6999999978150697, 7.000000000000000000 ) ) ;
#15030=CARTESIAN_POINT ( 'NONE',  ( 2.392413146961774206, 188.9999999991792947, 7.742749230693430462 ) ) ;
#15037=CARTESIAN_POINT ( 'NONE',  ( -1.016439536705160407E-17, 186.2499999989074979, 4.933012699999999029 ) ) ;
#15043=LINE ( 'NONE', #5731, #9385 ) ;
#15054=( BOUNDED_CURVE ( )  B_SPLINE_CURVE ( 2, ( #8534, #1190, #7253, #13363, #12173, #9641, #3581, #11138, #6144 ),
 .UNSPECIFIED., .F., .F. ) 
 B_SPLINE_CURVE_WITH_KNOTS ( ( 3, 2, 2, 2, 3 ),
 ( 0.5714285714285713969, 0.5892857142857143016, 0.6071428571428570953, 0.6250000000000000000, 0.6428571428571429047 ),
 .UNSPECIFIED. ) 
 CURVE ( )  GEOMETRIC_REPRESENTATION_ITEM ( )  RATIONAL_B_SPLINE_CURVE ( ( 1.000000000000000000, 0.9238795325112867385, 1.000000000000000000, 0.9238795325112867385, 1.000000000000000000, 0.9238795325112867385, 1.000000000000000000, 0.9238795325112867385, 1.000000000000000000 ) ) 
 REPRESENTATION_ITEM ( '' )  );
#15055=CARTESIAN_POINT ( 'NONE',  ( -0.3932117513507903395, 228.2473332724799207, 10.14534249745510586 ) ) ;
#15068=CARTESIAN_POINT ( 'NONE',  ( -2.500000000000000444, 185.1499999978150584, 8.035533905932737753 ) ) ;
#15073=CARTESIAN_POINT ( 'NONE',  ( -2.500000000000000444, 185.9199999975965625, 5.964466094067261359 ) ) ;
#15074=CARTESIAN_POINT ( 'NONE',  ( 1.865071889996124055, 228.0459258470066857, 9.553136980667057188 ) ) ;
#15075=CARTESIAN_POINT ( 'NONE',  ( -2.623350778723538834, 226.8212935938476278, 5.948734516926445615 ) ) ;
#15085=CARTESIAN_POINT ( 'NONE',  ( 1.359424073589828197, 228.1503905913944834, 9.860327814513095035 ) ) ;
#15092=CARTESIAN_POINT ( 'NONE',  ( -4.946672411965113980E-16, 184.5999999999999943, 9.500000000000001776 ) ) ;
#15093=CARTESIAN_POINT ( 'NONE',  ( 0.1304739971030711432, 227.6100227634930775, 5.113114354890055502 ) ) ;
#15097=CARTESIAN_POINT ( 'NONE',  ( 0.07162589071487505954, 189.0001276426230561, 4.501026264287848910 ) ) ;
#15098=CARTESIAN_POINT ( 'NONE',  ( -2.500000000000000444, 185.2499999999999716, 8.035533905932737753 ) ) ;
#15101=CARTESIAN_POINT ( 'NONE',  ( -0.8561741729129455081, 187.0999999989075206, 4.933012699999999029 ) ) ;
#15105=CARTESIAN_POINT ( 'NONE',  ( 0.000000000000000000, 222.7460571280668091, 12.08513476933103625 ) ) ;
#15107=CARTESIAN_POINT ( 'NONE',  ( 2.461882965037902160, 189.3814125599426745, 5.297573457840181632 ) ) ;
#15110=CARTESIAN_POINT ( 'NONE',  ( 2.977271291746630411, 189.8591517725882625, 7.726790542730640254 ) ) ;
#15115=CARTESIAN_POINT ( 'NONE',  ( 2.066987300000000527, 185.8499999989074922, 7.000000000000000000 ) ) ;
#15121=CARTESIAN_POINT ( 'NONE',  ( -2.500000000000000444, 185.9500000000000455, 5.964466094067261359 ) ) ;
#15128=CLOSED_SHELL ( 'NONE', ( #9031, #10865, #8786, #3797, #1329, #3694, #2180, #9812, #2629, #7753, #4952, #4245, #5805, #8136, #11046, #12358, #14591, #3087, #5564, #12210, #12765, #3174, #2433, #683, #12553, #6691, #4152 ) ) ;
#15133=CARTESIAN_POINT ( 'NONE',  ( -0.4907341119409533992, 228.2426455014340263, 10.13156071145469639 ) ) ;
#15146=CARTESIAN_POINT ( 'NONE',  ( -6.844026213814746740E-16, 187.6999999978150697, 9.500000000000001776 ) ) ;
#15147=CARTESIAN_POINT ( 'NONE',  ( 1.035533905932737753, 188.8499999978150470, 4.500000000000000888 ) ) ;
#15149=EDGE_CURVE ( 'NONE', #898, #6574, #7458, .T. ) ;
#15151=CARTESIAN_POINT ( 'NONE',  ( -1.998997755520148800E-16, 189.7699999975965568, 4.500000000000000000 ) ) ;
#15152=CARTESIAN_POINT ( 'NONE',  ( -0.8817132232236292166, 228.8448810635624682, 8.679455557192847337 ) ) ;
#15153=CARTESIAN_POINT ( 'NONE',  ( -2.668764612700158079, 227.7307401636093687, 8.626063590916809076 ) ) ;
#15168=CARTESIAN_POINT ( 'NONE',  ( -1.035533905932739529, 185.2499999978150811, 9.500000000000003553 ) ) ;
#15169=CARTESIAN_POINT ( 'NONE',  ( -0.6092285535620440839, 227.6401390286306992, 5.200091846327095979 ) ) ;
#15173=CARTESIAN_POINT ( 'NONE',  ( -7.420008617947670970E-16, 188.5999999999999943, 9.500000000000001776 ) ) ;
#15175=CARTESIAN_POINT ( 'NONE',  ( 1.461580736456472351, 188.3499999989074922, 8.461580736456474128 ) ) ;
#15176=VERTEX_POINT ( 'NONE', #14773 ) ;
#15185=CARTESIAN_POINT ( 'NONE',  ( 2.687945937111228645, 189.8130902236854070, 8.690539078995184852 ) ) ;
#15186=CARTESIAN_POINT ( 'NONE',  ( 2.500000000000000444, 187.9499999978150697, 5.964466094067262247 ) ) ;
#15188=CARTESIAN_POINT ( 'NONE',  ( 1.974798917232459150, 228.1755836975312945, 6.746486589875083872 ) ) ;
#15193=CARTESIAN_POINT ( 'NONE',  ( 1.461580736456472573, 186.5499999989075093, 8.461580736456474128 ) ) ;
#15195=B_SPLINE_CURVE_WITH_KNOTS ( 'NONE', 1,
 ( #12057, #8416 ),
 .UNSPECIFIED., .F., .F.,
 ( 2, 2 ),
 ( 0.000000000000000000, 1.000000000000000000 ),
 .UNSPECIFIED. ) ;
#15206=CARTESIAN_POINT ( 'NONE',  ( 5.999999999999999112, 215.7452399395091618, 13.29567785264566027 ) ) ;
#15209=CARTESIAN_POINT ( 'NONE',  ( 0.000000000000000000, 186.4999999978150527, 4.500000000000000000 ) ) ;
#15220=CARTESIAN_POINT ( 'NONE',  ( 2.066987300000000083, 185.2499999989074979, 7.000000000000000000 ) ) ;
#15225=CARTESIAN_POINT ( 'NONE',  ( 2.500000000000000000, 189.5699999975965397, 7.000000000000000000 ) ) ;
#15226=CARTESIAN_POINT ( 'NONE',  ( -0.8219475227482178070, 228.8541360017199224, 8.706184346459185264 ) ) ;
#15227=CARTESIAN_POINT ( 'NONE',  ( -0.9647310034392982958, 228.2043607281333379, 10.01900208526334168 ) ) ;
#15245=CARTESIAN_POINT ( 'NONE',  ( 2.500000000000000444, 186.3499999978150754, 5.964466094067262247 ) ) ;
#15247=CARTESIAN_POINT ( 'NONE',  ( 1.747590535343585438, 228.0744605602133674, 9.637048244069795544 ) ) ;
#15252=CARTESIAN_POINT ( 'NONE',  ( -1.767766952966369320, 185.9000000000000057, 5.232233047033630235 ) ) ;
#15258=CARTESIAN_POINT ( 'NONE',  ( -2.389652190990207536, 189.9828712853605168, 5.408448231032084941 ) ) ;
#15260=CARTESIAN_POINT ( 'NONE',  ( 0.7947751900520840795, 189.0000000008628831, 4.622669032342844098 ) ) ;
#15261=CARTESIAN_POINT ( 'NONE',  ( 2.500000000000000444, 185.5300000002184788, 7.000000000000000000 ) ) ;
#15264=CARTESIAN_POINT ( 'NONE',  ( 1.986724198295925836, 228.2179917342068052, 6.868963418589798309 ) ) ;
#15266=CARTESIAN_POINT ( 'NONE',  ( 2.500000000000000444, 184.0000000000000000, 7.000000000000000000 ) ) ;
#15270=CARTESIAN_POINT ( 'NONE',  ( 2.066987300000000083, 185.7999999989075093, 7.856174172912946396 ) ) ;
#15275=CARTESIAN_POINT ( 'NONE',  ( -2.500000000000000888, 188.2999999978150356, 7.000000000000000000 ) ) ;
#15280=CARTESIAN_POINT ( 'NONE',  ( 1.461580736456473462, 184.3499999989074922, 5.538419263543526760 ) ) ;
#15284=CARTESIAN_POINT ( 'NONE',  ( 0.000000000000000000, 186.5669965222008386, 9.317226423031119253 ) ) ;
#15297=PRODUCT_DEFINITION_SHAPE ( 'NONE', 'NONE',  #10321 ) ;
#15301=CARTESIAN_POINT ( 'NONE',  ( -1.456896669277396583E-16, 188.8999999978150584, 4.500000000000000000 ) ) ;
#15307=CARTESIAN_POINT ( 'NONE',  ( 0.6359992007181909379, 226.3469529472061765, 4.550856198837272437 ) ) ;
#15311=ORIENTED_EDGE ( 'NONE', *, *, #11196, .F. ) ;
#15317=VECTOR ( 'NONE', #8144, 1000.000000000000114 ) ;
#15319=CYLINDRICAL_SURFACE ( 'NONE', #9457, 2.500000000000000444 ) ;
#15325=CARTESIAN_POINT ( 'NONE',  ( 2.500000000000000000, 188.7500000000000000, 8.035533905932739529 ) ) ;
#15327=CARTESIAN_POINT ( 'NONE',  ( -1.974809306405319154, 228.1756194782155944, 6.746589926531873616 ) ) ;
#15333=CARTESIAN_POINT ( 'NONE',  ( 1.035533905932738197, 187.8500000000000227, 9.500000000000003553 ) ) ;
#15342=SURFACE_SIDE_STYLE ('',( #8103 ) ) ;
#15346=CARTESIAN_POINT ( 'NONE',  ( 1.581415667291661276, 227.8641612386227848, 5.847080766174051369 ) ) ;
#15353=CARTESIAN_POINT ( 'NONE',  ( 2.066987299999999195, 189.1999999989075434, 7.856174172912946396 ) ) ;
#15357=( BOUNDED_CURVE ( )  B_SPLINE_CURVE ( 2, ( #9401, #8213, #11777, #5904, #143, #13127, #3800, #14313, #12233, #6282, #7098, #961, #13049, #15452, #11044, #9786, #14237, #4553, #14633, #3874, #5827, #6946, #11935, #1041, #3722, #8600, #7391, #5007, #8674, #7467, #12310, #11122, #9936, #14788, #12969, #2072, #13816, #1487, #12388, #4034, #377, #12703, #10249, #2689, #5162, #13892, #7541, #1799, #9066, #531, #5401, #2851, #12467, #15101, #13743, #1722, #3005, #608, #2928, #11507, #4197, #7777, #10016, #10325, #13655, #11278, #6445, #6365, #5246, #10091, #6596, #10169, #12624, #301, #1569, #7863, #5481, #6674, #15175, #1645, #5325, #8747, #14942, #15024, #7623, #8826, #4117, #453, #11201, #13579, #14864, #3952, #11431, #8909, #7699, #2771, #12548, #6521, #11355, #8989, #10403 ),
 .UNSPECIFIED., .F., .F. ) 
 B_SPLINE_CURVE_WITH_KNOTS ( ( 3, 2, 2, 2, 2, 2, 2, 2, 2, 2, 2, 2, 2, 2, 2, 2, 2, 2, 2, 2, 2, 2, 2, 2, 2, 2, 2, 2, 2, 2, 2, 2, 2, 2, 2, 2, 2, 2, 2, 2, 2, 2, 2, 2, 2, 2, 2, 2, 2, 2, 3 ),
 ( 0.000000000000000000, 0.01785714285714285615, 0.03571428571428571230, 0.05357142857142856845, 0.07142857142857142461, 0.08928571428571428770, 0.1071428571428571369, 0.1250000000000000000, 0.1428571428571428492, 0.1607142857142857262, 0.1785714285714285754, 0.1964285714285714246, 0.2142857142857142738, 0.2321428571428571508, 0.2500000000000000000, 0.2678571428571428492, 0.2857142857142856984, 0.3035714285714285476, 0.3214285714285714524, 0.3392857142857143016, 0.3571428571428571508, 0.3750000000000000000, 0.3928571428571428492, 0.4107142857142856984, 0.4285714285714285476, 0.4464285714285714524, 0.4642857142857143016, 0.4821428571428571508, 0.5000000000000000000, 0.5178571428571429047, 0.5357142857142856984, 0.5535714285714286031, 0.5714285714285713969, 0.5892857142857143016, 0.6071428571428570953, 0.6250000000000000000, 0.6428571428571429047, 0.6607142857142856984, 0.6785714285714286031, 0.6964285714285715079, 0.7142857142857143016, 0.7321428571428570953, 0.7500000000000000000, 0.7678571428571429047, 0.7857142857142856984, 0.8035714285714286031, 0.8214285714285713969, 0.8392857142857143016, 0.8571428571428570953, 0.8750000000000000000, 0.8928571428571429047 ),
 .UNSPECIFIED. ) 
 CURVE ( )  GEOMETRIC_REPRESENTATION_ITEM ( )  RATIONAL_B_SPLINE_CURVE ( ( 1.000000000000000000, 0.9238795325112867385, 1.000000000000000000, 0.9238795325112867385, 1.000000000000000000, 0.9238795325112867385, 1.000000000000000000, 0.9238795325112867385, 1.000000000000000000, 0.9238795325112867385, 1.000000000000000000, 0.9238795325112867385, 1.000000000000000000, 0.9238795325112867385, 1.000000000000000000, 0.9238795325112867385, 1.000000000000000000, 0.9238795325112867385, 1.000000000000000000, 0.9238795325112867385, 1.000000000000000000, 0.9238795325112867385, 1.000000000000000000, 0.9238795325112867385, 1.000000000000000000, 0.9238795325112867385, 1.000000000000000000, 0.9238795325112867385, 1.000000000000000000, 0.9238795325112867385, 1.000000000000000000, 0.9238795325112867385, 1.000000000000000000, 0.9238795325112867385, 1.000000000000000000, 0.9238795325112867385, 1.000000000000000000, 0.9238795325112867385, 1.000000000000000000, 0.9238795325112867385, 1.000000000000000000, 0.9238795325112867385, 1.000000000000000000, 0.9238795325112867385, 1.000000000000000000, 0.9238795325112867385, 1.000000000000000000, 0.9238795325112867385, 1.000000000000000000, 0.9238795325112867385, 1.000000000000000000, 0.9238795325112867385, 1.000000000000000000, 0.9238795325112867385, 1.000000000000000000, 0.9238795325112867385, 1.000000000000000000, 0.9238795325112867385, 1.000000000000000000, 0.9238795325112867385, 1.000000000000000000, 0.9238795325112867385, 1.000000000000000000, 0.9238795325112867385, 1.000000000000000000, 0.9238795325112867385, 1.000000000000000000, 0.9238795325112867385, 1.000000000000000000, 0.9238795325112867385, 1.000000000000000000, 0.9238795325112867385, 1.000000000000000000, 0.9238795325112867385, 1.000000000000000000, 0.9238795325112867385, 1.000000000000000000, 0.9238795325112867385, 1.000000000000000000, 0.9238795325112867385, 1.000000000000000000, 0.9238795325112867385, 1.000000000000000000, 0.9238795325112867385, 1.000000000000000000, 0.9238795325112867385, 1.000000000000000000, 0.9238795325112867385, 1.000000000000000000, 0.9238795325112867385, 1.000000000000000000, 0.9238795325112867385, 1.000000000000000000, 0.9238795325112867385, 1.000000000000000000, 0.9238795325112867385, 1.000000000000000000, 0.9238795325112867385, 1.000000000000000000, 0.9238795325112867385, 1.000000000000000000 ) ) 
 REPRESENTATION_ITEM ( '' )  );
#15360=CARTESIAN_POINT ( 'NONE',  ( 1.461580736456473462, 185.9499999989075150, 5.538419263543526760 ) ) ;
#15364=CARTESIAN_POINT ( 'NONE',  ( 5.999999999999999112, 188.6555110544239824, 3.692234042173051289 ) ) ;
#15367=EDGE_CURVE ( 'NONE', #8616, #7973, #4694, .T. ) ;
#15371=VERTEX_POINT ( 'NONE', #6006 ) ;
#15379=CARTESIAN_POINT ( 'NONE',  ( -9.825582188149883933E-17, 188.0999999978150754, 4.500000000000000000 ) ) ;
#15386=CARTESIAN_POINT ( 'NONE',  ( 2.899241599682305992, 227.5396000034540975, 8.063657412308430139 ) ) ;
#15387=CARTESIAN_POINT ( 'NONE',  ( -0.3932117513507903395, 228.2473332724799207, 10.14534249745510586 ) ) ;
#15391=CARTESIAN_POINT ( 'NONE',  ( -2.500000000000000444, 185.9499999978150697, 8.035533905932737753 ) ) ;
#15404=CARTESIAN_POINT ( 'NONE',  ( 1.035533905932738419, 185.3499999978151038, 9.500000000000003553 ) ) ;
#15405=CARTESIAN_POINT ( 'NONE',  ( -1.454385272030960907, 228.7057613863525489, 8.277669994545302501 ) ) ;
#15409=CARTESIAN_POINT ( 'NONE',  ( -1.035533905932739751, 186.9499999999999886, 9.500000000000003553 ) ) ;
#15416=CARTESIAN_POINT ( 'NONE',  ( -2.753814924773092976, 227.6725260165826796, 8.454791258317579050 ) ) ;
#15423=CARTESIAN_POINT ( 'NONE',  ( 0.6402346998162695701, 228.8776282932165600, 8.774031424212344277 ) ) ;
#15427=CARTESIAN_POINT ( 'NONE',  ( -1.461580736456473018, 185.3499999989074922, 5.538419263543526760 ) ) ;
#15429=CARTESIAN_POINT ( 'NONE',  ( -2.500000000000000444, 184.4499999999999886, 8.035533905932737753 ) ) ;
#15438=CARTESIAN_POINT ( 'NONE',  ( -1.461580736456473684, 185.5499999989075093, 8.461580736456474128 ) ) ;
#15449=VERTEX_POINT ( 'NONE', #12433 ) ;
#15452=CARTESIAN_POINT ( 'NONE',  ( 0.8561741729129461742, 185.0999999989075206, 9.066987299999999195 ) ) ;
#15453=CARTESIAN_POINT ( 'NONE',  ( 0.5183317123408758276, 227.6299956641393294, 5.170797231135993322 ) ) ;
#15459=CARTESIAN_POINT ( 'NONE',  ( 2.500000000000000000, 189.4999999978150527, 7.000000000000000000 ) ) ;
#15463=CARTESIAN_POINT ( 'NONE',  ( -2.500000000000000888, 189.2199999975965738, 8.035533905932737753 ) ) ;
#15464=CARTESIAN_POINT ( 'NONE',  ( -0.1984404311693547251, 226.3267777912124075, 4.491376718485652120 ) ) ;
#15468=AXIS2_PLACEMENT_3D ( 'NONE', #11375, #14886, #7955 ) ;
#15470=CARTESIAN_POINT ( 'NONE',  ( -1.035533905932739751, 188.4499999978150697, 9.500000000000000000 ) ) ;
#15471=( BOUNDED_SURFACE ( )  B_SPLINE_SURFACE ( 3, 2, ( 
 ( #998, #8498, #14271 ),
 ( #2183, #915, #6022 ),
 ( #13249, #5941, #9519 ),
 ( #11972, #7217, #3462 ),
 ( #10866, #9441, #14608 ),
 ( #13166, #10708, #15493 ),
 ( #4827, #12134, #11889 ),
 ( #6982, #11811, #2265 ),
 ( #1235, #10944, #15645 ),
 ( #7137, #43, #4589 ),
 ( #1078, #4908, #13326 ),
 ( #2428, #14843, #13720 ),
 ( #277, #5140, #7598 ),
 ( #14767, #356, #14686 ),
 ( #6340, #13558, #13406 ),
 ( #7520, #5304, #12287 ),
 ( #121, #11176, #1308 ),
 ( #12365, #9993, #12211 ),
 ( #12446, #3928, #1464 ),
 ( #7369, #5061, #11334 ),
 ( #13633, #6499, #4011 ),
 ( #2668, #1623, #431 ),
 ( #8576, #8804, #6421 ),
 ( #6183, #12524, #11022 ),
 ( #2748, #14919, #1546 ),
 ( #4986, #3775, #11255 ),
 ( #8888, #9836, #5222 ),
 ( #10070, #2828, #7676 ),
 ( #10150, #15004, #2515 ),
 ( #8652, #13483, #2587 ),
 ( #7442, #200, #1386 ),
 ( #6261, #11099, #9914 ) ),
 .UNSPECIFIED., .F., .F., .F. ) 
 B_SPLINE_SURFACE_WITH_KNOTS ( ( 4, 2, 2, 2, 2, 2, 2, 2, 2, 2, 2, 2, 2, 2, 2, 4 ),
 ( 3, 3 ),
 ( 0.006495126007820955193, 0.006901071383536445600, 0.007307016759251935140, 0.007712962134967425547, 0.008118907510682915954, 0.008524852886398405494, 0.008930798262113896768, 0.009742689013544875848, 0.01014863438926036539, 0.01055457976497585493, 0.01096052514069134620, 0.01136647051640683574, 0.01177241589212232528, 0.01217836126783781656, 0.01258430664355330610, 0.01299025201926879564 ),
 ( 0.000000000000000000, 1.000000000000000000 ),
 .UNSPECIFIED. ) 
 GEOMETRIC_REPRESENTATION_ITEM ( )  RATIONAL_B_SPLINE_SURFACE ( (
 ( 1.000000000000000000, 0.8259116554769078133, 1.000000000000000000),
 ( 1.000000000000000000, 0.8257451403044092642, 1.000000000000000000),
 ( 1.000000000000000000, 0.8262262825652272324, 1.000000000000000000),
 ( 1.000000000000000000, 0.8282882085239741121, 1.000000000000000000),
 ( 1.000000000000000000, 0.8298670479083970486, 1.000000000000000000),
 ( 1.000000000000000000, 0.8338618467773711851, 1.000000000000000000),
 ( 1.000000000000000000, 0.8362196290431722634, 1.000000000000000000),
 ( 1.000000000000000000, 0.8411780429153195016, 1.000000000000000000),
 ( 1.000000000000000000, 0.8438131714200759470, 1.000000000000000000),
 ( 1.000000000000000000, 0.8487328695746524376, 1.000000000000000000),
 ( 1.000000000000000000, 0.8510248968242735135, 1.000000000000000000),
 ( 1.000000000000000000, 0.8549300986948997760, 1.000000000000000000),
 ( 1.000000000000000000, 0.8565209868850615083, 1.000000000000000000),
 ( 1.000000000000000000, 0.8598120940792107758, 1.000000000000000000),
 ( 1.000000000000000000, 0.8600061557766143228, 1.000000000000000000),
 ( 1.000000000000000000, 0.8577564625823946853, 1.000000000000000000),
 ( 1.000000000000000000, 0.8565991989799338624, 1.000000000000000000),
 ( 1.000000000000000000, 0.8537317661690416726, 1.000000000000000000),
 ( 1.000000000000000000, 0.8520458150393346308, 1.000000000000000000),
 ( 1.000000000000000000, 0.8483981972192249366, 1.000000000000000000),
 ( 1.000000000000000000, 0.8464144394435542118, 1.000000000000000000),
 ( 1.000000000000000000, 0.8424405162120318646, 1.000000000000000000),
 ( 1.000000000000000000, 0.8404672314583410131, 1.000000000000000000),
 ( 1.000000000000000000, 0.8366782202000002666, 1.000000000000000000),
 ( 1.000000000000000000, 0.8348411284253109965, 1.000000000000000000),
 ( 1.000000000000000000, 0.8315664188806370927, 1.000000000000000000),
 ( 1.000000000000000000, 0.8301207044443068561, 1.000000000000000000),
 ( 1.000000000000000000, 0.8276856662744687121, 1.000000000000000000),
 ( 1.000000000000000000, 0.8267013226302402096, 1.000000000000000000),
 ( 1.000000000000000000, 0.8253456704432764468, 1.000000000000000000),
 ( 1.000000000000000000, 0.8249566822916403197, 1.000000000000000000),
 ( 1.000000000000000000, 0.8248771365966394153, 1.000000000000000000) ) ) 
 REPRESENTATION_ITEM ( '' )  SURFACE ( )  );
#15489=( BOUNDED_CURVE ( )  B_SPLINE_CURVE ( 2, ( #14306, #3415, #11928, #8286, #13120, #5897, #10744, #15603, #12402 ),
 .UNSPECIFIED., .F., .F. ) 
 B_SPLINE_CURVE_WITH_KNOTS ( ( 3, 2, 2, 2, 3 ),
 ( 0.07142857142857141073, 0.08928571428571427382, 0.1071428571428571230, 0.1250000000000000000, 0.1428571428571428492 ),
 .UNSPECIFIED. ) 
 CURVE ( )  GEOMETRIC_REPRESENTATION_ITEM ( )  RATIONAL_B_SPLINE_CURVE ( ( 1.000000000000000000, 0.9238795325112866275, 1.000000000000000000, 0.9238795325112867385, 1.000000000000000000, 0.9238795325112867385, 1.000000000000000000, 0.9238795325112867385, 1.000000000000000000 ) ) 
 REPRESENTATION_ITEM ( '' )  );
#15490=CARTESIAN_POINT ( 'NONE',  ( -2.500000000000000444, 185.8999999978150584, 7.000000000000000000 ) ) ;
#15491=CARTESIAN_POINT ( 'NONE',  ( 0.7764192831524953098, 228.2223555856212442, 10.07190823357606213 ) ) ;
#15493=CARTESIAN_POINT ( 'NONE',  ( -1.304415936767590489, 190.0585524576826799, 4.499160646538907571 ) ) ;
#15495=CARTESIAN_POINT ( 'NONE',  ( 1.767766952966368432, 187.8999999999999773, 8.767766952966368876 ) ) ;
#15500=CARTESIAN_POINT ( 'NONE',  ( 1.035533905932737753, 186.5499999999999829, 4.500000000000001776 ) ) ;
#15501=CARTESIAN_POINT ( 'NONE',  ( -2.361157410827141145, 226.6937665785872014, 5.572992748502056948 ) ) ;
#15503=CARTESIAN_POINT ( 'NONE',  ( 1.767766952966369320, 184.8300000002185186, 5.232233047033630235 ) ) ;
#15505=CARTESIAN_POINT ( 'NONE',  ( 0.8799020092372641377, 228.8451675208714562, 8.680282862240067843 ) ) ;
#15517=CARTESIAN_POINT ( 'NONE',  ( -2.066987300000000527, 185.3999999989075889, 6.143825827087054492 ) ) ;
#15521=CARTESIAN_POINT ( 'NONE',  ( 0.000000000000000000, 222.7460571280668091, 12.08513476933103625 ) ) ;
#15525=EDGE_CURVE ( 'NONE', #320, #8616, #10680, .T. ) ;
#15530=CARTESIAN_POINT ( 'NONE',  ( 1.500101834665445999, 227.8300896185262161, 5.748679984017036837 ) ) ;
#15533=VECTOR ( 'NONE', #9609, 1000.000000000000000 ) ;
#15538=CARTESIAN_POINT ( 'NONE',  ( 0.8561741729129460632, 186.6999999989075150, 9.066987299999999195 ) ) ;
#15545=CARTESIAN_POINT ( 'NONE',  ( 1.751153496549405775, 226.5057898163625794, 5.019064844972819017 ) ) ;
#15547=ORIENTED_EDGE ( 'NONE', *, *, #9136, .T. ) ;
#15562=CARTESIAN_POINT ( 'NONE',  ( 1.767766952966369098, 187.9999999978150527, 5.232233047033630235 ) ) ;
#15563=CARTESIAN_POINT ( 'NONE',  ( 1.625192428541204714, 228.1012562471100011, 9.715842694323066908 ) ) ;
#15578=CARTESIAN_POINT ( 'NONE',  ( -2.534040306409066190, 227.8072189287023832, 8.851078430691819321 ) ) ;
#15579=CARTESIAN_POINT ( 'NONE',  ( 0.3078036515352236546, 189.4415565186901347, 3.987496826561411911 ) ) ;
#15580=CARTESIAN_POINT ( 'NONE',  ( -2.500000000000000444, 185.8800000002185300, 5.964466094067261359 ) ) ;
#15582=CARTESIAN_POINT ( 'NONE',  ( -0.8818726034074957365, 227.6760006002180319, 5.303662110480990677 ) ) ;
#15587=CARTESIAN_POINT ( 'NONE',  ( 1.461580736456472573, 187.3499999989074922, 8.461580736456474128 ) ) ;
#15589=CARTESIAN_POINT ( 'NONE',  ( 0.8561741729129457301, 185.9999999989074979, 4.933012699999999029 ) ) ;
#15598=CARTESIAN_POINT ( 'NONE',  ( -2.066987300000000527, 186.9999999989075263, 6.143825827087054492 ) ) ;
#15602=CARTESIAN_POINT ( 'NONE',  ( 1.767766952966369320, 184.0999999999999943, 5.232233047033630235 ) ) ;
#15603=CARTESIAN_POINT ( 'NONE',  ( 2.500000000000000444, 185.4499999978150981, 8.035533905932739529 ) ) ;
#15605=CARTESIAN_POINT ( 'NONE',  ( -0.01285886373251123212, 189.6977690162252941, 10.38967773564543684 ) ) ;
#15610=CARTESIAN_POINT ( 'NONE',  ( -0.0007128680628333008105, 227.6089742637946642, 5.110086227958842819 ) ) ;
#15615=CARTESIAN_POINT ( 'NONE',  ( 1.461580736456472351, 187.5499999989075093, 8.461580736456474128 ) ) ;
#15620=CARTESIAN_POINT ( 'NONE',  ( -0.1001789588503840533, 226.3251931448050698, 4.486704830075608719 ) ) ;
#15629=EDGE_CURVE ( 'NONE', #12014, #1272, #12299, .T. ) ;
#15632=EDGE_CURVE ( 'NONE', #7444, #25, #5181, .T. ) ;
#15641=CARTESIAN_POINT ( 'NONE',  ( -1.767766952966369765, 187.5999999978150754, 8.767766952966368876 ) ) ;
#15643=CARTESIAN_POINT ( 'NONE',  ( 2.993808330938719564, 227.3535049858431591, 7.515946948957763496 ) ) ;
#15645=CARTESIAN_POINT ( 'NONE',  ( -1.972033150788811806, 190.0185192967513501, 4.950362254874026036 ) ) ;
#15650=ORIENTED_EDGE ( 'NONE', *, *, #5238, .F. ) ;
#15652=CARTESIAN_POINT ( 'NONE',  ( 1.734160753182337755, 226.5019027256826121, 5.007583146736123147 ) ) ;
#15655=CARTESIAN_POINT ( 'NONE',  ( -2.766897257556299117, 227.6625976227142019, 8.425578970441488735 ) ) ;
#15656=FILL_AREA_STYLE ('',( #14132 ) ) ;
#15658=CARTESIAN_POINT ( 'NONE',  ( -1.035533905932739751, 186.8800000002184731, 9.500000000000003553 ) ) ;
#15660=CARTESIAN_POINT ( 'NONE',  ( 1.052850409966403333, 227.7074407335792614, 5.394463008855642450 ) ) ;
#15666=CARTESIAN_POINT ( 'NONE',  ( 2.066987300000000083, 188.2499999989075263, 7.000000000000000000 ) ) ;
#15668=CARTESIAN_POINT ( 'NONE',  ( 2.066987300000000971, 187.4999999989075548, 6.143825827087054492 ) ) ;
#15670=ORIENTED_EDGE ( 'NONE', *, *, #14464, .T. ) ;
#15676=CARTESIAN_POINT ( 'NONE',  ( 5.999999999999999112, 189.3270225533669020, 3.938484906660877805 ) ) ;
#15677=CARTESIAN_POINT ( 'NONE',  ( -2.066987300000000971, 187.0999999989075206, 7.856174172912944620 ) ) ;
#15679=CARTESIAN_POINT ( 'NONE',  ( 0.8615349496598407875, 189.0583051017248977, 10.06290867563976654 ) ) ;
#15682=CARTESIAN_POINT ( 'NONE',  ( -1.767766952966369320, 188.9999999978150527, 5.232233047033630235 ) ) ;
#15689=CARTESIAN_POINT ( 'NONE',  ( 1.727282114035952443, 228.5870706176066278, 7.934884284728715542 ) ) ;
#15695=CARTESIAN_POINT ( 'NONE',  ( 0.8561741729129452860, 188.5999999989074922, 4.933012699999999029 ) ) ;
#15702=CARTESIAN_POINT ( 'NONE',  ( -1.240485740468941556, 226.4108687305035232, 4.739277288743133809 ) ) ;
#15706=CARTESIAN_POINT ( 'NONE',  ( -7.352245982167326943E-16, 188.4999999978150527, 9.500000000000001776 ) ) ;
#15726=CARTESIAN_POINT ( 'NONE',  ( -7.352245982167326943E-16, 188.4999999978150527, 9.500000000000001776 ) ) ;
#15727=AXIS2_PLACEMENT_3D ( 'NONE', #12188, #2319, #7192 ) ;
#15728=CARTESIAN_POINT ( 'NONE',  ( 2.691218579993890803, 227.7172414894967858, 8.586351398698511161 ) ) ;
#15729=CARTESIAN_POINT ( 'NONE',  ( -2.940898392866930777E-15, 228.9118723800512498, 8.872930300147352511 ) ) ;
ENDSEC;
END-ISO-10303-21;
